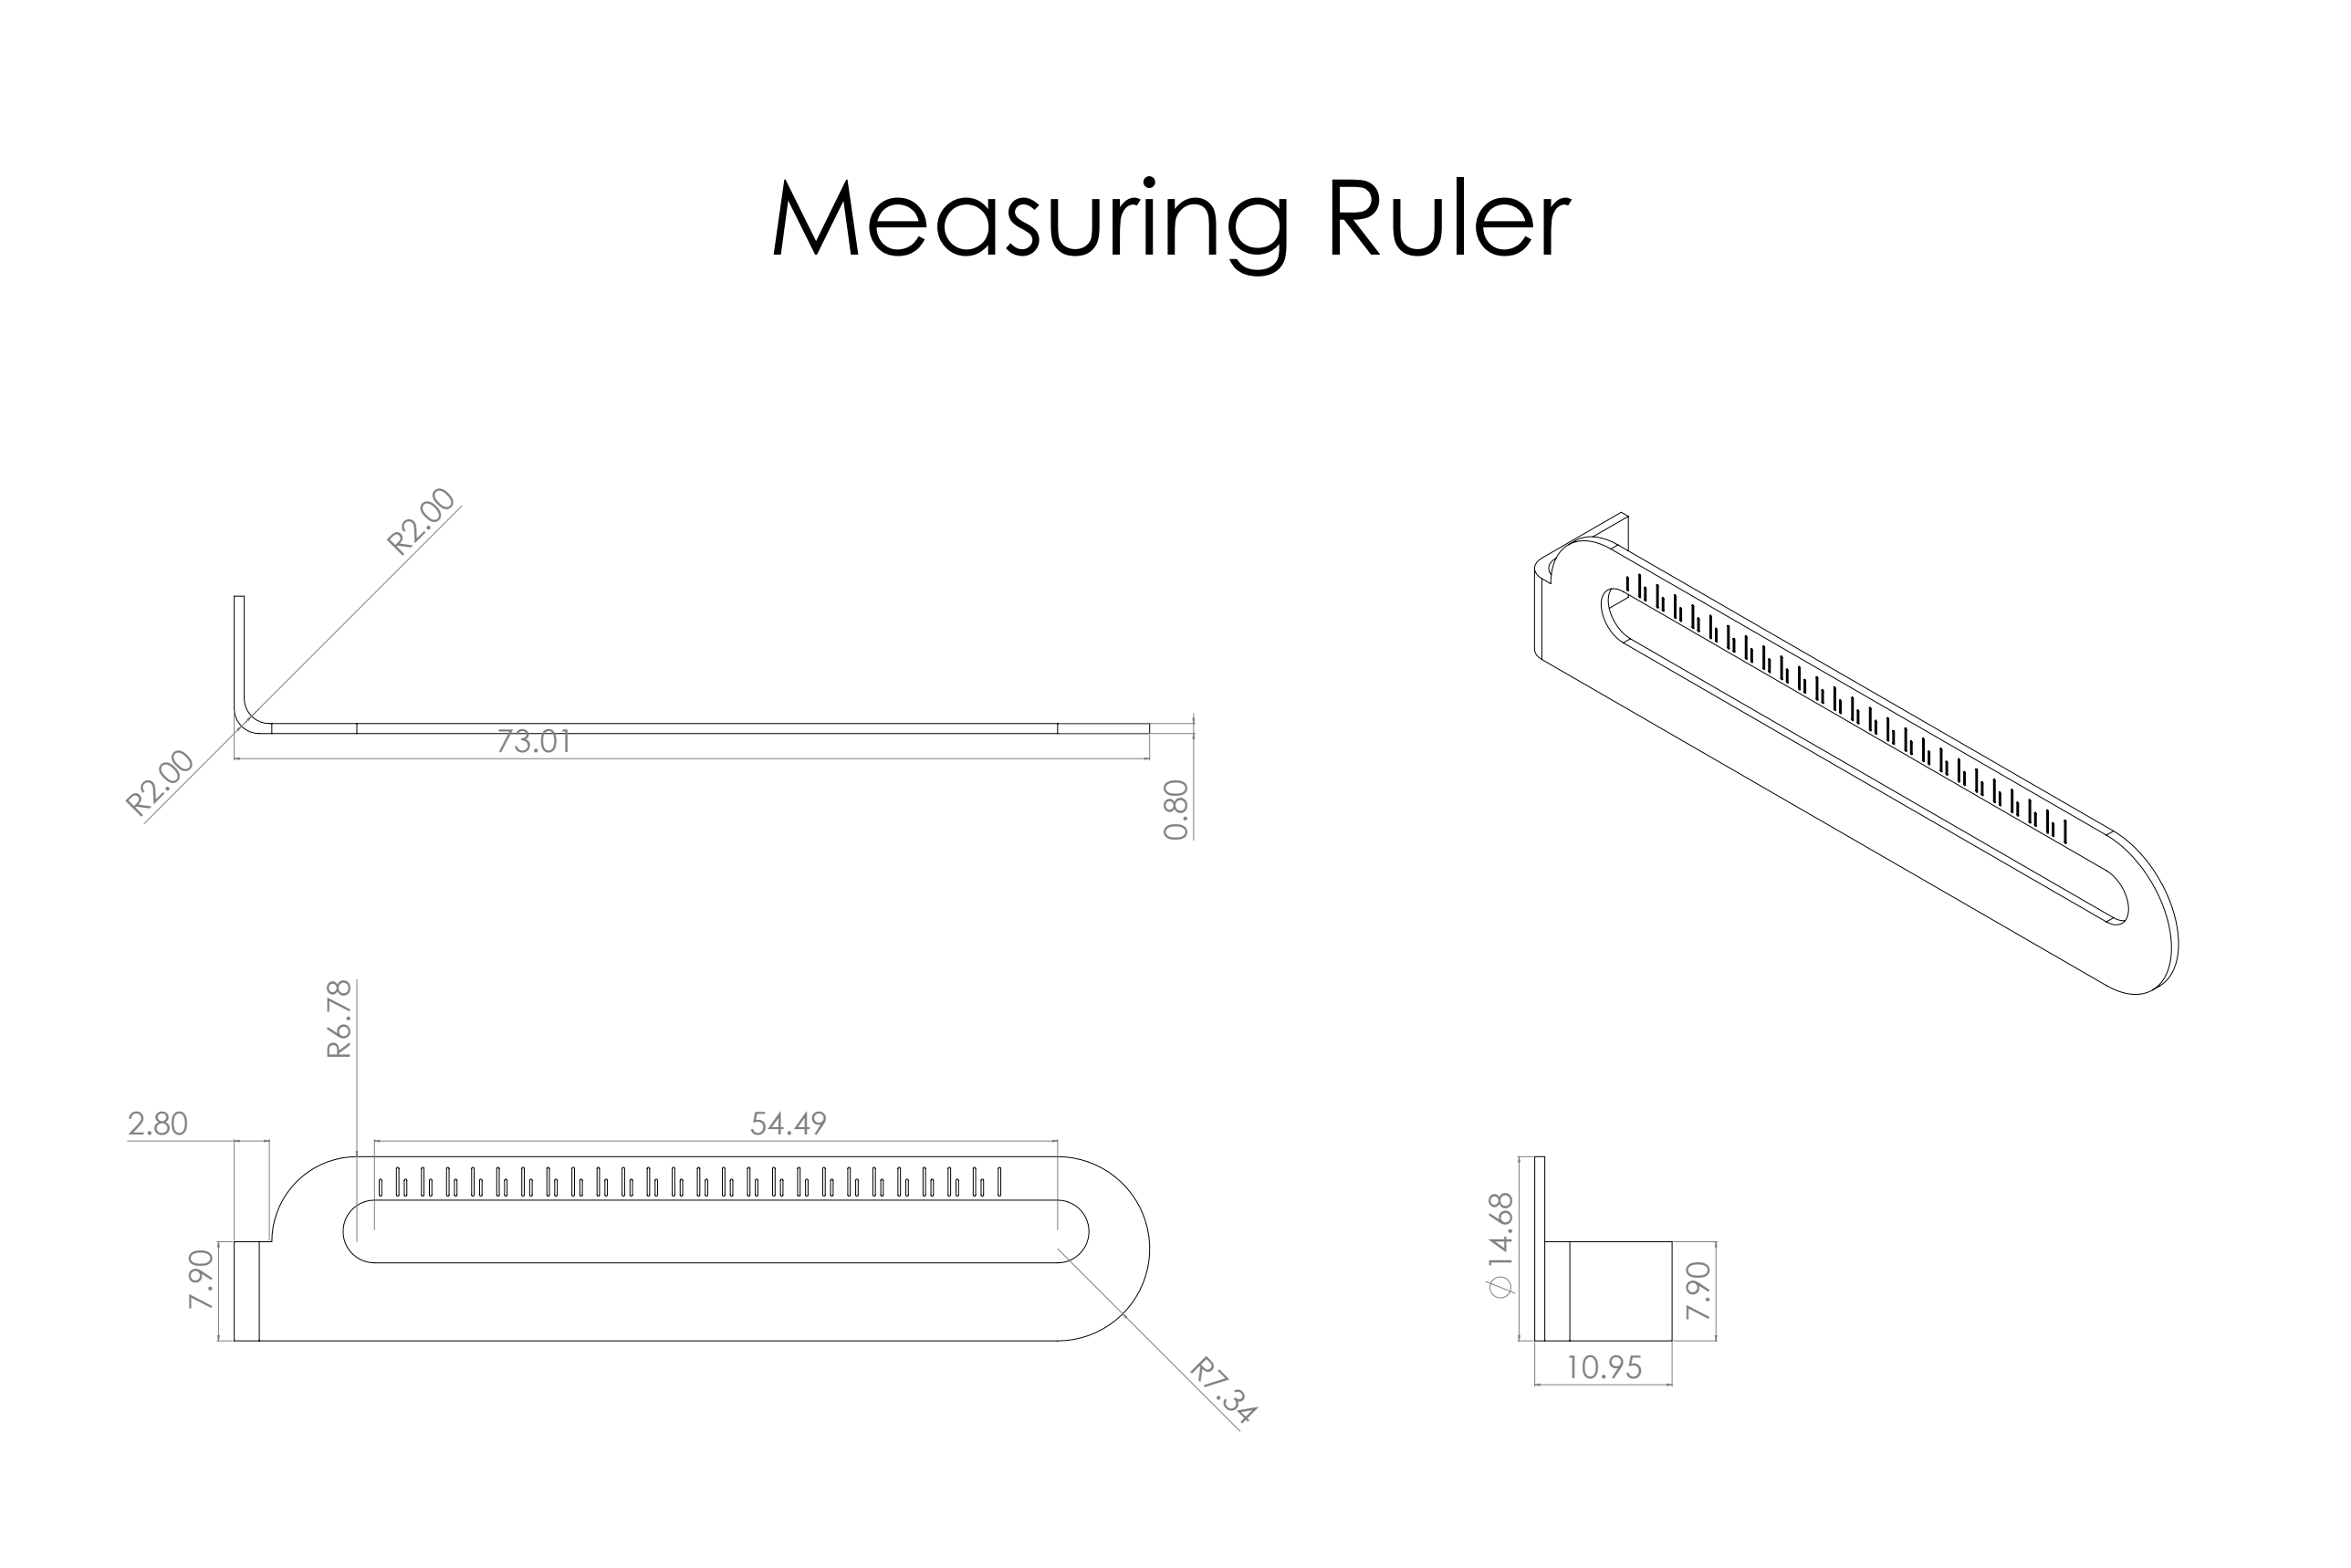
ISO-10303-21;
HEADER;
FILE_DESCRIPTION (('STEP AP214'),
    '1' );
FILE_NAME ('Measuring Ruler.step',
    '2026-10-24T22:54:28',
    ( '' ),
    ( '' ),
    'SwSTEP 2.0',
    'SolidWorks 2025',
    '' );
FILE_SCHEMA (( 'AUTOMOTIVE_DESIGN' ));
ENDSEC;

DATA;
#22=CIRCLE ( 'NONE', #10506, 0.1000000000000028644 ) ;
#24=ORIENTED_EDGE ( 'NONE', *, *, #28416, .F. ) ;
#30=EDGE_CURVE ( 'NONE', #25319, #33264, #34800, .T. ) ;
#32=ORIENTED_EDGE ( 'NONE', *, *, #7574, .F. ) ;
#37=DIRECTION ( 'NONE',  ( 1.000000000000000000, 0.000000000000000000, 0.000000000000000000 ) ) ;
#41=ORIENTED_EDGE ( 'NONE', *, *, #18908, .F. ) ;
#44=DIRECTION ( 'NONE',  ( -0.000000000000000000, -0.000000000000000000, 1.000000000000000000 ) ) ;
#48=CIRCLE ( 'NONE', #2012, 0.1000000000000028644 ) ;
#49=CARTESIAN_POINT ( 'NONE',  ( -32.87867591359218977, -26.64985754041175525, 6.700000000000000178 ) ) ;
#51=ORIENTED_EDGE ( 'NONE', *, *, #25814, .F. ) ;
#52=FACE_BOUND ( 'NONE', #30582, .T. ) ;
#54=EDGE_LOOP ( 'NONE', ( #15981, #402, #1244, #38858 ) ) ;
#57=EDGE_CURVE ( 'NONE', #6790, #7577, #6515, .T. ) ;
#60=ORIENTED_EDGE ( 'NONE', *, *, #39491, .F. ) ;
#63=CARTESIAN_POINT ( 'NONE',  ( -19.07867591359219972, -24.55319635012989110, 6.800000000000000711 ) ) ;
#69=DIRECTION ( 'NONE',  ( 0.000000000000000000, 0.000000000000000000, 1.000000000000000000 ) ) ;
#80=EDGE_CURVE ( 'NONE', #2391, #5443, #34066, .T. ) ;
#89=DIRECTION ( 'NONE',  ( -0.000000000000000000, -0.000000000000000000, 1.000000000000000000 ) ) ;
#92=CARTESIAN_POINT ( 'NONE',  ( -14.44874870218064089, -26.64985754041175525, 6.700000000000000178 ) ) ;
#93=ORIENTED_EDGE ( 'NONE', *, *, #2114, .F. ) ;
#96=AXIS2_PLACEMENT_3D ( 'NONE', #13585, #39295, #10487 ) ;
#107=VECTOR ( 'NONE', #13832, 1000.000000000000000 ) ;
#112=CARTESIAN_POINT ( 'NONE',  ( -40.44874870218063734, -26.64985754041175525, 6.700000000000000178 ) ) ;
#116=EDGE_CURVE ( 'NONE', #25222, #15928, #15693, .T. ) ;
#121=EDGE_LOOP ( 'NONE', ( #23412, #22869, #10746, #16528 ) ) ;
#138=VECTOR ( 'NONE', #4313, 1000.000000000000000 ) ;
#160=VERTEX_POINT ( 'NONE', #28468 ) ;
#162=DIRECTION ( 'NONE',  ( 1.000000000000000000, 0.000000000000000000, 0.000000000000000000 ) ) ;
#168=EDGE_CURVE ( 'NONE', #27559, #13108, #28679, .T. ) ;
#169=VERTEX_POINT ( 'NONE', #9734 ) ;
#172=ADVANCED_FACE ( 'NONE', ( #34882 ), #28059, .T. ) ;
#179=LINE ( 'NONE', #33956, #26669 ) ;
#182=CARTESIAN_POINT ( 'NONE',  ( -32.44874870218063734, -26.64985754041175525, 6.700000000000000178 ) ) ;
#188=EDGE_LOOP ( 'NONE', ( #27353, #29698, #8514, #37884 ) ) ;
#192=AXIS2_PLACEMENT_3D ( 'NONE', #26818, #39356, #4992 ) ;
#194=DIRECTION ( 'NONE',  ( -0.000000000000000000, -1.000000000000000000, -0.000000000000000000 ) ) ;
#203=ORIENTED_EDGE ( 'NONE', *, *, #13724, .F. ) ;
#205=CARTESIAN_POINT ( 'NONE',  ( -31.07867591359219617, -26.64985754041175525, 6.700000000000000178 ) ) ;
#210=VECTOR ( 'NONE', #7329, 1000.000000000000000 ) ;
#212=VERTEX_POINT ( 'NONE', #19008 ) ;
#219=VECTOR ( 'NONE', #28713, 1000.000000000000000 ) ;
#221=ORIENTED_EDGE ( 'NONE', *, *, #39543, .T. ) ;
#228=CARTESIAN_POINT ( 'NONE',  ( -38.34874870218063592, -25.49307895267003587, 6.800000000000000711 ) ) ;
#229=VECTOR ( 'NONE', #9739, 1000.000000000000000 ) ;
#230=AXIS2_PLACEMENT_3D ( 'NONE', #30843, #30009, #20734 ) ;
#232=ORIENTED_EDGE ( 'NONE', *, *, #27570, .F. ) ;
#236=EDGE_CURVE ( 'NONE', #37067, #38999, #489, .T. ) ;
#239=ORIENTED_EDGE ( 'NONE', *, *, #18400, .F. ) ;
#245=FACE_BOUND ( 'NONE', #8668, .T. ) ;
#247=ORIENTED_EDGE ( 'NONE', *, *, #38016, .F. ) ;
#253=ORIENTED_EDGE ( 'NONE', *, *, #18491, .F. ) ;
#256=CARTESIAN_POINT ( 'NONE',  ( -20.24874870218063805, -26.64985754041175525, 6.800000000000000711 ) ) ;
#261=CARTESIAN_POINT ( 'NONE',  ( -31.07867591359219617, -26.64985754041175525, 6.700000000000000178 ) ) ;
#264=EDGE_CURVE ( 'NONE', #4144, #39141, #13023, .T. ) ;
#273=VERTEX_POINT ( 'NONE', #6042 ) ;
#287=ORIENTED_EDGE ( 'NONE', *, *, #2540, .F. ) ;
#291=VECTOR ( 'NONE', #8251, 1000.000000000000000 ) ;
#292=ORIENTED_EDGE ( 'NONE', *, *, #32328, .T. ) ;
#295=CARTESIAN_POINT ( 'NONE',  ( -28.44874870218064444, -26.64985754041175525, 6.700000000000000178 ) ) ;
#301=VERTEX_POINT ( 'NONE', #29083 ) ;
#308=AXIS2_PLACEMENT_3D ( 'NONE', #26975, #18099, #31499 ) ;
#316=CARTESIAN_POINT ( 'NONE',  ( -20.24874870218063805, -25.49307895267003587, 6.800000000000000711 ) ) ;
#324=CIRCLE ( 'NONE', #4910, 0.1000000000000028644 ) ;
#325=AXIS2_PLACEMENT_3D ( 'NONE', #22553, #3830, #34311 ) ;
#333=CARTESIAN_POINT ( 'NONE',  ( -40.87867591359218977, -26.64985754041175525, 6.700000000000000178 ) ) ;
#334=LINE ( 'NONE', #37983, #38784 ) ;
#335=VECTOR ( 'NONE', #17674, 1000.000000000000000 ) ;
#337=DIRECTION ( 'NONE',  ( -0.000000000000000000, -0.000000000000000000, 1.000000000000000000 ) ) ;
#339=CARTESIAN_POINT ( 'NONE',  ( -18.44874870218064089, -26.64985754041175525, 6.800000000000000711 ) ) ;
#340=ORIENTED_EDGE ( 'NONE', *, *, #35850, .F. ) ;
#342=ADVANCED_FACE ( 'NONE', ( #36253 ), #23687, .F. ) ;
#351=EDGE_CURVE ( 'NONE', #2784, #15795, #11729, .T. ) ;
#356=AXIS2_PLACEMENT_3D ( 'NONE', #19003, #36206, #4906 ) ;
#365=ORIENTED_EDGE ( 'NONE', *, *, #29479, .F. ) ;
#366=PLANE ( 'NONE',  #31779 ) ;
#375=LINE ( 'NONE', #9824, #24005 ) ;
#387=AXIS2_PLACEMENT_3D ( 'NONE', #30030, #29821, #1845 ) ;
#388=AXIS2_PLACEMENT_3D ( 'NONE', #3065, #40471, #13104 ) ;
#390=CARTESIAN_POINT ( 'NONE',  ( -19.07867591359219972, -24.55319635012989110, 6.700000000000000178 ) ) ;
#397=ORIENTED_EDGE ( 'NONE', *, *, #11518, .F. ) ;
#402=ORIENTED_EDGE ( 'NONE', *, *, #15855, .F. ) ;
#403=CARTESIAN_POINT ( 'NONE',  ( -10.97867591359219475, -24.55319635012989110, 6.800000000000000711 ) ) ;
#405=ORIENTED_EDGE ( 'NONE', *, *, #6491, .T. ) ;
#406=CARTESIAN_POINT ( 'NONE',  ( 0.9213240864078056092, -26.64985754041175525, 6.800000000000000711 ) ) ;
#407=EDGE_CURVE ( 'NONE', #9686, #33055, #7841, .T. ) ;
#408=VERTEX_POINT ( 'NONE', #26392 ) ;
#414=VECTOR ( 'NONE', #27211, 1000.000000000000000 ) ;
#423=VECTOR ( 'NONE', #27841, 1000.000000000000000 ) ;
#430=EDGE_LOOP ( 'NONE', ( #38499, #2239, #5855, #4124 ) ) ;
#438=DIRECTION ( 'NONE',  ( 1.000000000000000000, 0.000000000000000000, 0.000000000000000000 ) ) ;
#439=FACE_OUTER_BOUND ( 'NONE', #33105, .T. ) ;
#442=ORIENTED_EDGE ( 'NONE', *, *, #39133, .F. ) ;
#444=DIRECTION ( 'NONE',  ( 1.000000000000000000, 0.000000000000000000, 0.000000000000000000 ) ) ;
#450=ORIENTED_EDGE ( 'NONE', *, *, #24702, .T. ) ;
#456=FACE_BOUND ( 'NONE', #19493, .T. ) ;
#457=ORIENTED_EDGE ( 'NONE', *, *, #19911, .F. ) ;
#469=DIRECTION ( 'NONE',  ( 1.000000000000000000, 0.000000000000000000, -0.000000000000000000 ) ) ;
#472=CARTESIAN_POINT ( 'NONE',  ( 7.021324086407807030, -26.64985754041175525, 6.800000000000000711 ) ) ;
#477=CARTESIAN_POINT ( 'NONE',  ( -36.44874870218064444, -26.64985754041175525, 6.800000000000000711 ) ) ;
#480=EDGE_CURVE ( 'NONE', #34939, #11908, #22301, .T. ) ;
#482=VECTOR ( 'NONE', #26893, 1000.000000000000000 ) ;
#484=AXIS2_PLACEMENT_3D ( 'NONE', #25294, #37829, #22816 ) ;
#489=LINE ( 'NONE', #19409, #17633 ) ;
#492=CARTESIAN_POINT ( 'NONE',  ( 3.121324086407806231, -24.55319635012989110, 6.800000000000000711 ) ) ;
#504=ORIENTED_EDGE ( 'NONE', *, *, #40555, .F. ) ;
#510=CIRCLE ( 'NONE', #40591, 0.1000000000000028644 ) ;
#511=AXIS2_PLACEMENT_3D ( 'NONE', #33114, #5508, #36395 ) ;
#512=DIRECTION ( 'NONE',  ( 1.000000000000000000, -0.000000000000000000, 0.000000000000000000 ) ) ;
#513=VERTEX_POINT ( 'NONE', #23285 ) ;
#525=CARTESIAN_POINT ( 'NONE',  ( -28.44874870218064444, -26.64985754041175525, 6.800000000000000711 ) ) ;
#528=EDGE_CURVE ( 'NONE', #40182, #12066, #7030, .T. ) ;
#529=DIRECTION ( 'NONE',  ( 0.000000000000000000, 1.000000000000000000, 0.000000000000000000 ) ) ;
#534=DIRECTION ( 'NONE',  ( 0.000000000000000000, 1.000000000000000000, 0.000000000000000000 ) ) ;
#543=EDGE_CURVE ( 'NONE', #29781, #29208, #27533, .T. ) ;
#547=CARTESIAN_POINT ( 'NONE',  ( -31.07867591359219617, -26.64985754041175525, 6.700000000000000178 ) ) ;
#554=ADVANCED_FACE ( 'NONE', ( #16885 ), #25774, .F. ) ;
#563=CIRCLE ( 'NONE', #18272, 0.1000000000000028644 ) ;
#570=AXIS2_PLACEMENT_3D ( 'NONE', #16960, #5023, #19858 ) ;
#578=DIRECTION ( 'NONE',  ( -0.000000000000000000, -0.000000000000000000, 1.000000000000000000 ) ) ;
#594=CARTESIAN_POINT ( 'NONE',  ( -26.87867591359219333, -26.64985754041175525, 6.700000000000000178 ) ) ;
#605=ORIENTED_EDGE ( 'NONE', *, *, #39024, .T. ) ;
#607=ORIENTED_EDGE ( 'NONE', *, *, #26724, .T. ) ;
#608=VECTOR ( 'NONE', #5163, 1000.000000000000000 ) ;
#619=DIRECTION ( 'NONE',  ( 0.000000000000000000, 0.000000000000000000, -1.000000000000000000 ) ) ;
#630=EDGE_LOOP ( 'NONE', ( #15162, #24602, #9016, #12961 ) ) ;
#641=ADVANCED_FACE ( 'NONE', ( #18306 ), #6386, .T. ) ;
#642=AXIS2_PLACEMENT_3D ( 'NONE', #18718, #9661, #9043 ) ;
#650=VERTEX_POINT ( 'NONE', #31702 ) ;
#653=CARTESIAN_POINT ( 'NONE',  ( -8.448748702180639114, -26.64985754041175525, 6.700000000000000178 ) ) ;
#656=EDGE_LOOP ( 'NONE', ( #16676, #14194, #23824, #26128 ) ) ;
#659=ORIENTED_EDGE ( 'NONE', *, *, #28607, .F. ) ;
#661=CARTESIAN_POINT ( 'NONE',  ( -4.978675913592189417, -26.64985754041175525, 6.800000000000000711 ) ) ;
#662=ORIENTED_EDGE ( 'NONE', *, *, #39276, .T. ) ;
#682=ADVANCED_FACE ( 'NONE', ( #22247 ), #28186, .F. ) ;
#683=AXIS2_PLACEMENT_3D ( 'NONE', #24668, #40497, #3294 ) ;
#687=CARTESIAN_POINT ( 'NONE',  ( 5.121324086407808451, -26.64985754041175525, 6.800000000000000711 ) ) ;
#697=AXIS2_PLACEMENT_3D ( 'NONE', #25369, #6431, #21672 ) ;
#699=VERTEX_POINT ( 'NONE', #31500 ) ;
#706=CARTESIAN_POINT ( 'NONE',  ( 2.921324086407800280, -26.64985754041175525, 6.700000000000000178 ) ) ;
#710=CARTESIAN_POINT ( 'NONE',  ( -24.87867591359218977, -26.64985754041175525, 6.700000000000000178 ) ) ;
#719=AXIS2_PLACEMENT_3D ( 'NONE', #16756, #1542, #11181 ) ;
#721=DIRECTION ( 'NONE',  ( -1.000000000000000000, 0.000000000000000000, 0.000000000000000000 ) ) ;
#730=EDGE_CURVE ( 'NONE', #28082, #6110, #14379, .T. ) ;
#739=VECTOR ( 'NONE', #13481, 1000.000000000000000 ) ;
#740=DIRECTION ( 'NONE',  ( 1.000000000000000000, 0.000000000000000000, -0.000000000000000000 ) ) ;
#744=VERTEX_POINT ( 'NONE', #2705 ) ;
#745=AXIS2_PLACEMENT_3D ( 'NONE', #8431, #24083, #11717 ) ;
#746=ORIENTED_EDGE ( 'NONE', *, *, #18980, .F. ) ;
#752=ORIENTED_EDGE ( 'NONE', *, *, #26701, .T. ) ;
#756=CYLINDRICAL_SURFACE ( 'NONE', #23191, 0.1000000000000028644 ) ;
#759=CARTESIAN_POINT ( 'NONE',  ( 6.921324086407803833, -24.55319635012989110, 6.800000000000000711 ) ) ;
#779=ADVANCED_FACE ( 'NONE', ( #28815 ), #25521, .F. ) ;
#793=EDGE_CURVE ( 'NONE', #37191, #15824, #9816, .T. ) ;
#794=LINE ( 'NONE', #22821, #9570 ) ;
#796=ORIENTED_EDGE ( 'NONE', *, *, #39201, .T. ) ;
#801=ORIENTED_EDGE ( 'NONE', *, *, #26499, .T. ) ;
#806=ORIENTED_EDGE ( 'NONE', *, *, #32982, .T. ) ;
#813=AXIS2_PLACEMENT_3D ( 'NONE', #2939, #28428, #28639 ) ;
#817=CARTESIAN_POINT ( 'NONE',  ( 5.751251297819365504, -25.49307895267003587, 6.700000000000000178 ) ) ;
#821=CYLINDRICAL_SURFACE ( 'NONE', #26427, 0.1000000000000028644 ) ;
#825=ORIENTED_EDGE ( 'NONE', *, *, #17697, .T. ) ;
#826=VERTEX_POINT ( 'NONE', #19549 ) ;
#840=CYLINDRICAL_SURFACE ( 'NONE', #9559, 0.1000000000000028644 ) ;
#844=CARTESIAN_POINT ( 'NONE',  ( 5.751251297819365504, -26.64985754041175525, 6.700000000000000178 ) ) ;
#846=LINE ( 'NONE', #13981, #2059 ) ;
#848=EDGE_LOOP ( 'NONE', ( #12316, #20240, #26085, #37691 ) ) ;
#849=ORIENTED_EDGE ( 'NONE', *, *, #22675, .F. ) ;
#854=EDGE_CURVE ( 'NONE', #36422, #301, #38867, .T. ) ;
#856=ORIENTED_EDGE ( 'NONE', *, *, #2258, .T. ) ;
#857=ADVANCED_FACE ( 'NONE', ( #8582 ), #23435, .F. ) ;
#860=ORIENTED_EDGE ( 'NONE', *, *, #25488, .F. ) ;
#861=FACE_BOUND ( 'NONE', #37475, .T. ) ;
#863=VERTEX_POINT ( 'NONE', #8375 ) ;
#865=EDGE_CURVE ( 'NONE', #14656, #4406, #26525, .T. ) ;
#876=LINE ( 'NONE', #31758, #28712 ) ;
#877=EDGE_CURVE ( 'NONE', #28154, #25277, #11252, .T. ) ;
#899=CARTESIAN_POINT ( 'NONE',  ( -54.01549048184568846, -38.28842912540938670, 4.800000000000000711 ) ) ;
#901=CYLINDRICAL_SURFACE ( 'NONE', #8152, 0.1000000000000028644 ) ;
#907=EDGE_CURVE ( 'NONE', #5789, #22409, #33321, .T. ) ;
#915=AXIS2_PLACEMENT_3D ( 'NONE', #29380, #4276, #4480 ) ;
#916=EDGE_CURVE ( 'NONE', #8305, #24066, #39886, .T. ) ;
#927=ORIENTED_EDGE ( 'NONE', *, *, #964, .F. ) ;
#930=ORIENTED_EDGE ( 'NONE', *, *, #27699, .T. ) ;
#935=EDGE_LOOP ( 'NONE', ( #34001, #29049, #22823, #20751 ) ) ;
#941=CARTESIAN_POINT ( 'NONE',  ( -4.878675913592187108, -26.64985754041175525, 6.700000000000000178 ) ) ;
#942=DIRECTION ( 'NONE',  ( 1.000000000000000000, 0.000000000000000000, -0.000000000000000000 ) ) ;
#943=CIRCLE ( 'NONE', #6193, 0.1000000000000028644 ) ;
#946=VECTOR ( 'NONE', #20283, 1000.000000000000000 ) ;
#956=CARTESIAN_POINT ( 'NONE',  ( -34.34874870218063592, -26.64985754041175525, 6.700000000000000178 ) ) ;
#964=EDGE_CURVE ( 'NONE', #14571, #23320, #17842, .T. ) ;
#967=CARTESIAN_POINT ( 'NONE',  ( -26.34874870218063947, -25.49307895267003587, 6.700000000000000178 ) ) ;
#970=EDGE_LOOP ( 'NONE', ( #15579, #17607, #22271, #8008 ) ) ;
#972=LINE ( 'NONE', #29558, #210 ) ;
#986=CARTESIAN_POINT ( 'NONE',  ( -26.34874870218063947, -26.64985754041175525, 6.700000000000000178 ) ) ;
#993=CARTESIAN_POINT ( 'NONE',  ( -32.87867591359218977, -24.55319635012989110, 6.700000000000000178 ) ) ;
#1000=ADVANCED_FACE ( 'NONE', ( #27123 ), #39673, .F. ) ;
#1001=AXIS2_PLACEMENT_3D ( 'NONE', #28881, #26404, #13835 ) ;
#1013=ORIENTED_EDGE ( 'NONE', *, *, #7946, .T. ) ;
#1018=FACE_OUTER_BOUND ( 'NONE', #9894, .T. ) ;
#1020=EDGE_LOOP ( 'NONE', ( #6917, #5481, #6006, #10397 ) ) ;
#1046=CARTESIAN_POINT ( 'NONE',  ( 4.921324086407802056, -26.64985754041175525, 6.800000000000000711 ) ) ;
#1049=EDGE_CURVE ( 'NONE', #35752, #27725, #24236, .T. ) ;
#1053=DIRECTION ( 'NONE',  ( 0.000000000000000000, 0.000000000000000000, 1.000000000000000000 ) ) ;
#1056=ORIENTED_EDGE ( 'NONE', *, *, #36941, .T. ) ;
#1062=CIRCLE ( 'NONE', #24030, 0.1000000000000028644 ) ;
#1065=DIRECTION ( 'NONE',  ( 0.000000000000000000, 0.000000000000000000, 1.000000000000000000 ) ) ;
#1066=ADVANCED_FACE ( 'NONE', ( #18462 ), #18664, .F. ) ;
#1074=CARTESIAN_POINT ( 'NONE',  ( -40.44874870218063734, -25.49307895267003587, 6.700000000000000178 ) ) ;
#1086=LINE ( 'NONE', #32373, #21513 ) ;
#1091=DIRECTION ( 'NONE',  ( -0.000000000000000000, -0.000000000000000000, -1.000000000000000000 ) ) ;
#1096=EDGE_CURVE ( 'NONE', #25156, #27940, #9398, .T. ) ;
#1104=EDGE_CURVE ( 'NONE', #38102, #33506, #2654, .T. ) ;
#1108=CIRCLE ( 'NONE', #9635, 0.1000000000000028644 ) ;
#1111=CARTESIAN_POINT ( 'NONE',  ( -34.44874870218064444, -26.64985754041175525, 6.800000000000000711 ) ) ;
#1125=CARTESIAN_POINT ( 'NONE',  ( -40.44874870218063734, -25.49307895267003587, 6.700000000000000178 ) ) ;
#1135=CIRCLE ( 'NONE', #6382, 0.1000000000000028644 ) ;
#1142=VERTEX_POINT ( 'NONE', #37201 ) ;
#1148=EDGE_CURVE ( 'NONE', #7017, #3657, #26261, .T. ) ;
#1149=VERTEX_POINT ( 'NONE', #37403 ) ;
#1152=DIRECTION ( 'NONE',  ( -0.000000000000000000, -0.000000000000000000, 1.000000000000000000 ) ) ;
#1166=CIRCLE ( 'NONE', #39261, 0.1000000000000028644 ) ;
#1173=DIRECTION ( 'NONE',  ( -0.000000000000000000, -0.000000000000000000, 1.000000000000000000 ) ) ;
#1174=ORIENTED_EDGE ( 'NONE', *, *, #2356, .F. ) ;
#1187=LINE ( 'NONE', #35955, #946 ) ;
#1190=VERTEX_POINT ( 'NONE', #4067 ) ;
#1195=DIRECTION ( 'NONE',  ( 0.000000000000000000, 1.000000000000000000, 0.000000000000000000 ) ) ;
#1207=AXIS2_PLACEMENT_3D ( 'NONE', #23187, #22594, #13911 ) ;
#1211=CYLINDRICAL_SURFACE ( 'NONE', #10209, 0.1000000000000028644 ) ;
#1216=AXIS2_PLACEMENT_3D ( 'NONE', #27119, #20943, #2227 ) ;
#1220=PLANE ( 'NONE',  #30647 ) ;
#1223=EDGE_LOOP ( 'NONE', ( #35956, #16011, #20211, #34093 ) ) ;
#1235=CARTESIAN_POINT ( 'NONE',  ( -40.44874870218063734, -26.64985754041175525, 6.700000000000000178 ) ) ;
#1237=ORIENTED_EDGE ( 'NONE', *, *, #1249, .T. ) ;
#1238=DIRECTION ( 'NONE',  ( 0.000000000000000000, 0.000000000000000000, 1.000000000000000000 ) ) ;
#1244=ORIENTED_EDGE ( 'NONE', *, *, #36356, .F. ) ;
#1249=EDGE_CURVE ( 'NONE', #12996, #5611, #7868, .T. ) ;
#1251=CARTESIAN_POINT ( 'NONE',  ( -14.24874870218063450, -25.49307895267003587, 6.700000000000000178 ) ) ;
#1255=DIRECTION ( 'NONE',  ( 1.000000000000000000, 0.000000000000000000, 0.000000000000000000 ) ) ;
#1267=EDGE_CURVE ( 'NONE', #26853, #22787, #24958, .T. ) ;
#1269=VERTEX_POINT ( 'NONE', #3673 ) ;
#1273=AXIS2_PLACEMENT_3D ( 'NONE', #4046, #3453, #6716 ) ;
#1285=CARTESIAN_POINT ( 'NONE',  ( -35.07867591359219972, -24.55319635012989110, 6.700000000000000178 ) ) ;
#1287=CARTESIAN_POINT ( 'NONE',  ( -5.078675913592192614, -26.64985754041175525, 6.800000000000000711 ) ) ;
#1291=CARTESIAN_POINT ( 'NONE',  ( 7.121324086407810228, -26.64985754041175525, 6.700000000000000178 ) ) ;
#1293=FACE_OUTER_BOUND ( 'NONE', #4220, .T. ) ;
#1298=LINE ( 'NONE', #26205, #3633 ) ;
#1299=FACE_OUTER_BOUND ( 'NONE', #3763, .T. ) ;
#1303=CYLINDRICAL_SURFACE ( 'NONE', #14814, 0.1000000000000028644 ) ;
#1316=DIRECTION ( 'NONE',  ( -0.000000000000000000, -0.000000000000000000, 1.000000000000000000 ) ) ;
#1326=CARTESIAN_POINT ( 'NONE',  ( -5.078675913592192614, -24.55319635012989110, 6.800000000000000711 ) ) ;
#1343=ORIENTED_EDGE ( 'NONE', *, *, #10404, .T. ) ;
#1344=CARTESIAN_POINT ( 'NONE',  ( -2.448748702180640446, -26.64985754041175525, 6.800000000000000711 ) ) ;
#1345=VECTOR ( 'NONE', #9294, 1000.000000000000000 ) ;
#1346=VERTEX_POINT ( 'NONE', #25375 ) ;
#1349=DIRECTION ( 'NONE',  ( -1.000000000000000000, 0.000000000000000000, 0.000000000000000000 ) ) ;
#1352=DIRECTION ( 'NONE',  ( 0.000000000000000000, 0.000000000000000000, 1.000000000000000000 ) ) ;
#1364=ORIENTED_EDGE ( 'NONE', *, *, #15068, .T. ) ;
#1368=CARTESIAN_POINT ( 'NONE',  ( -29.07867591359219617, -24.55319635012989110, 6.700000000000000178 ) ) ;
#1378=EDGE_CURVE ( 'NONE', #22687, #28211, #22091, .T. ) ;
#1389=CARTESIAN_POINT ( 'NONE',  ( -22.97867591359219119, -26.64985754041175525, 6.700000000000000178 ) ) ;
#1406=DIRECTION ( 'NONE',  ( -0.000000000000000000, -0.000000000000000000, 1.000000000000000000 ) ) ;
#1408=CARTESIAN_POINT ( 'NONE',  ( -6.878675913592188884, -26.64985754041175525, 6.800000000000000711 ) ) ;
#1412=FACE_OUTER_BOUND ( 'NONE', #24496, .T. ) ;
#1427=CARTESIAN_POINT ( 'NONE',  ( -20.87867591359218977, -24.55319635012989110, 6.700000000000000178 ) ) ;
#1435=CYLINDRICAL_SURFACE ( 'NONE', #15585, 0.1000000000000028644 ) ;
#1439=ORIENTED_EDGE ( 'NONE', *, *, #10916, .F. ) ;
#1445=CYLINDRICAL_SURFACE ( 'NONE', #14804, 0.1000000000000028644 ) ;
#1448=DIRECTION ( 'NONE',  ( 0.000000000000000000, 0.000000000000000000, 1.000000000000000000 ) ) ;
#1456=CARTESIAN_POINT ( 'NONE',  ( -4.248748702180636272, -26.64985754041175525, 6.700000000000000178 ) ) ;
#1461=CARTESIAN_POINT ( 'NONE',  ( -16.44874870218064089, -26.64985754041175525, 6.700000000000000178 ) ) ;
#1464=ORIENTED_EDGE ( 'NONE', *, *, #37587, .F. ) ;
#1472=FACE_OUTER_BOUND ( 'NONE', #14916, .T. ) ;
#1477=CARTESIAN_POINT ( 'NONE',  ( -14.44874870218064089, -25.49307895267003587, 6.800000000000000711 ) ) ;
#1478=CARTESIAN_POINT ( 'NONE',  ( 1.751251297819361730, -26.64985754041175525, 6.700000000000000178 ) ) ;
#1490=VECTOR ( 'NONE', #40411, 1000.000000000000000 ) ;
#1497=ORIENTED_EDGE ( 'NONE', *, *, #13901, .F. ) ;
#1528=ORIENTED_EDGE ( 'NONE', *, *, #12883, .F. ) ;
#1532=EDGE_CURVE ( 'NONE', #34807, #36832, #20388, .T. ) ;
#1535=ORIENTED_EDGE ( 'NONE', *, *, #18438, .F. ) ;
#1542=DIRECTION ( 'NONE',  ( 1.000000000000000000, -0.000000000000000000, 0.000000000000000000 ) ) ;
#1546=ADVANCED_FACE ( 'NONE', ( #35270 ), #19994, .F. ) ;
#1547=VERTEX_POINT ( 'NONE', #1477 ) ;
#1552=EDGE_LOOP ( 'NONE', ( #32484, #9373, #40170, #13436 ) ) ;
#1554=FACE_OUTER_BOUND ( 'NONE', #12637, .T. ) ;
#1555=LINE ( 'NONE', #1760, #19571 ) ;
#1558=CARTESIAN_POINT ( 'NONE',  ( -42.83131703149249603, -27.06993018339339585, 6.800000000000000711 ) ) ;
#1563=ORIENTED_EDGE ( 'NONE', *, *, #10637, .F. ) ;
#1569=CARTESIAN_POINT ( 'NONE',  ( -40.34874870218063592, -26.64985754041175525, 6.700000000000000178 ) ) ;
#1578=VECTOR ( 'NONE', #27868, 1000.000000000000000 ) ;
#1588=AXIS2_PLACEMENT_3D ( 'NONE', #33095, #29997, #36380 ) ;
#1593=AXIS2_PLACEMENT_3D ( 'NONE', #1881, #39938, #8632 ) ;
#1605=DIRECTION ( 'NONE',  ( 0.000000000000000000, 0.000000000000000000, 1.000000000000000000 ) ) ;
#1606=ORIENTED_EDGE ( 'NONE', *, *, #8051, .T. ) ;
#1608=AXIS2_PLACEMENT_3D ( 'NONE', #15904, #35622, #3386 ) ;
#1609=EDGE_LOOP ( 'NONE', ( #12170, #36601, #32369, #22372 ) ) ;
#1611=DIRECTION ( 'NONE',  ( 0.000000000000000000, 1.000000000000000000, 0.000000000000000000 ) ) ;
#1616=AXIS2_PLACEMENT_3D ( 'NONE', #28205, #37666, #37 ) ;
#1623=ORIENTED_EDGE ( 'NONE', *, *, #25818, .F. ) ;
#1625=ADVANCED_FACE ( 'NONE', ( #36450 ), #39738, .F. ) ;
#1632=ORIENTED_EDGE ( 'NONE', *, *, #32386, .F. ) ;
#1634=VERTEX_POINT ( 'NONE', #39327 ) ;
#1635=VECTOR ( 'NONE', #32985, 1000.000000000000000 ) ;
#1646=ADVANCED_FACE ( 'NONE', ( #4754 ), #33787, .T. ) ;
#1648=CARTESIAN_POINT ( 'NONE',  ( -10.97867591359219475, -26.64985754041175525, 6.800000000000000711 ) ) ;
#1651=ORIENTED_EDGE ( 'NONE', *, *, #17090, .F. ) ;
#1662=VERTEX_POINT ( 'NONE', #21427 ) ;
#1670=VECTOR ( 'NONE', #17832, 1000.000000000000000 ) ;
#1672=VERTEX_POINT ( 'NONE', #27382 ) ;
#1682=DIRECTION ( 'NONE',  ( -0.000000000000000000, -0.000000000000000000, 1.000000000000000000 ) ) ;
#1689=CARTESIAN_POINT ( 'NONE',  ( -40.87867591359218977, -26.64985754041175525, 6.700000000000000178 ) ) ;
#1694=DIRECTION ( 'NONE',  ( 0.000000000000000000, 1.000000000000000000, 0.000000000000000000 ) ) ;
#1699=CARTESIAN_POINT ( 'NONE',  ( -34.87867591359218977, -26.64985754041175525, 6.700000000000000178 ) ) ;
#1701=ADVANCED_FACE ( 'NONE', ( #1892 ), #8641, .F. ) ;
#1709=DIRECTION ( 'NONE',  ( 1.000000000000000000, 0.000000000000000000, 0.000000000000000000 ) ) ;
#1714=FACE_OUTER_BOUND ( 'NONE', #25111, .T. ) ;
#1720=ORIENTED_EDGE ( 'NONE', *, *, #30483, .F. ) ;
#1726=EDGE_CURVE ( 'NONE', #37911, #1142, #33590, .T. ) ;
#1728=CIRCLE ( 'NONE', #31979, 0.1000000000000028644 ) ;
#1739=EDGE_CURVE ( 'NONE', #13396, #17894, #21216, .T. ) ;
#1741=CYLINDRICAL_SURFACE ( 'NONE', #26897, 0.1000000000000028644 ) ;
#1751=EDGE_CURVE ( 'NONE', #39647, #9655, #36653, .T. ) ;
#1752=ORIENTED_EDGE ( 'NONE', *, *, #9288, .F. ) ;
#1759=CARTESIAN_POINT ( 'NONE',  ( -16.24874870218063450, -26.64985754041175525, 6.700000000000000178 ) ) ;
#1760=CARTESIAN_POINT ( 'NONE',  ( -38.87867591359218977, -24.55319635012989110, 6.700000000000000178 ) ) ;
#1763=CARTESIAN_POINT ( 'NONE',  ( -14.87867591359218977, -24.55319635012989110, 6.800000000000000711 ) ) ;
#1765=CARTESIAN_POINT ( 'NONE',  ( -42.44874870218064444, -26.64985754041175525, 6.800000000000000711 ) ) ;
#1776=ADVANCED_FACE ( 'NONE', ( #26788 ), #18106, .T. ) ;
#1783=CIRCLE ( 'NONE', #5060, 0.1000000000000028644 ) ;
#1789=CARTESIAN_POINT ( 'NONE',  ( -21.07867591359219617, -24.55319635012989110, 6.700000000000000178 ) ) ;
#1794=AXIS2_PLACEMENT_3D ( 'NONE', #16703, #23114, #7454 ) ;
#1797=FACE_OUTER_BOUND ( 'NONE', #1223, .T. ) ;
#1810=VERTEX_POINT ( 'NONE', #22041 ) ;
#1816=ORIENTED_EDGE ( 'NONE', *, *, #22261, .T. ) ;
#1824=ORIENTED_EDGE ( 'NONE', *, *, #4744, .F. ) ;
#1825=AXIS2_PLACEMENT_3D ( 'NONE', #26664, #13699, #35935 ) ;
#1831=FACE_OUTER_BOUND ( 'NONE', #14855, .T. ) ;
#1835=VERTEX_POINT ( 'NONE', #22257 ) ;
#1836=CARTESIAN_POINT ( 'NONE',  ( -4.878675913592187108, -26.64985754041175525, 6.700000000000000178 ) ) ;
#1845=DIRECTION ( 'NONE',  ( -1.000000000000000000, 0.000000000000000000, 0.000000000000000000 ) ) ;
#1846=ORIENTED_EDGE ( 'NONE', *, *, #6440, .T. ) ;
#1847=VECTOR ( 'NONE', #38622, 1000.000000000000000 ) ;
#1853=DIRECTION ( 'NONE',  ( 1.000000000000000000, -0.000000000000000000, 0.000000000000000000 ) ) ;
#1854=VERTEX_POINT ( 'NONE', #19145 ) ;
#1856=AXIS2_PLACEMENT_3D ( 'NONE', #19788, #35652, #4360 ) ;
#1858=ORIENTED_EDGE ( 'NONE', *, *, #20133, .T. ) ;
#1863=DIRECTION ( 'NONE',  ( 0.000000000000000000, 0.000000000000000000, 1.000000000000000000 ) ) ;
#1865=DIRECTION ( 'NONE',  ( 0.000000000000000000, 0.000000000000000000, -1.000000000000000000 ) ) ;
#1866=ORIENTED_EDGE ( 'NONE', *, *, #31728, .F. ) ;
#1870=EDGE_LOOP ( 'NONE', ( #14802, #25233, #20620, #14309 ) ) ;
#1874=VERTEX_POINT ( 'NONE', #34209 ) ;
#1875=EDGE_CURVE ( 'NONE', #37531, #18951, #31711, .T. ) ;
#1881=CARTESIAN_POINT ( 'NONE',  ( -38.97867591359219119, -24.55319635012989110, 6.700000000000000178 ) ) ;
#1886=ORIENTED_EDGE ( 'NONE', *, *, #30787, .T. ) ;
#1891=ADVANCED_FACE ( 'NONE', ( #11099 ), #39514, .F. ) ;
#1892=FACE_OUTER_BOUND ( 'NONE', #37559, .T. ) ;
#1894=DIRECTION ( 'NONE',  ( -0.000000000000000000, -0.000000000000000000, 1.000000000000000000 ) ) ;
#1908=CYLINDRICAL_SURFACE ( 'NONE', #36747, 0.1000000000000028644 ) ;
#1914=DIRECTION ( 'NONE',  ( 1.000000000000000000, 0.000000000000000000, 0.000000000000000000 ) ) ;
#1915=EDGE_LOOP ( 'NONE', ( #25208, #504, #34556, #14770 ) ) ;
#1922=CARTESIAN_POINT ( 'NONE',  ( -24.24874870218063450, -26.64985754041175525, 6.700000000000000178 ) ) ;
#1923=ORIENTED_EDGE ( 'NONE', *, *, #27065, .T. ) ;
#1927=VECTOR ( 'NONE', #36002, 1000.000000000000000 ) ;
#1938=EDGE_CURVE ( 'NONE', #11548, #21166, #3302, .T. ) ;
#1950=VECTOR ( 'NONE', #31112, 1000.000000000000000 ) ;
#1951=CARTESIAN_POINT ( 'NONE',  ( -42.34874870218063592, -25.49307895267003587, 6.700000000000000178 ) ) ;
#1963=AXIS2_PLACEMENT_3D ( 'NONE', #24863, #34356, #162 ) ;
#1977=ORIENTED_EDGE ( 'NONE', *, *, #3672, .F. ) ;
#1980=VERTEX_POINT ( 'NONE', #9444 ) ;
#1985=DIRECTION ( 'NONE',  ( 0.000000000000000000, 0.000000000000000000, 1.000000000000000000 ) ) ;
#2012=AXIS2_PLACEMENT_3D ( 'NONE', #37068, #27397, #30291 ) ;
#2021=ORIENTED_EDGE ( 'NONE', *, *, #4492, .F. ) ;
#2027=ORIENTED_EDGE ( 'NONE', *, *, #21238, .T. ) ;
#2039=CARTESIAN_POINT ( 'NONE',  ( -52.01549048184568846, -30.94667987854474234, 4.800000000000000711 ) ) ;
#2041=CIRCLE ( 'NONE', #39505, 0.1000000000000028644 ) ;
#2046=CARTESIAN_POINT ( 'NONE',  ( 2.921324086407800280, -26.64985754041175525, 6.700000000000000178 ) ) ;
#2051=CARTESIAN_POINT ( 'NONE',  ( 3.551251297819357777, -25.49307895267003587, 6.800000000000000711 ) ) ;
#2054=LINE ( 'NONE', #27347, #37824 ) ;
#2059=VECTOR ( 'NONE', #22867, 1000.000000000000000 ) ;
#2064=CIRCLE ( 'NONE', #23726, 0.1000000000000028644 ) ;
#2066=ADVANCED_FACE ( 'NONE', ( #19129 ), #29751, .F. ) ;
#2068=CYLINDRICAL_SURFACE ( 'NONE', #40521, 0.1000000000000028644 ) ;
#2070=ORIENTED_EDGE ( 'NONE', *, *, #18627, .T. ) ;
#2073=VERTEX_POINT ( 'NONE', #32454 ) ;
#2079=ORIENTED_EDGE ( 'NONE', *, *, #27186, .T. ) ;
#2091=CARTESIAN_POINT ( 'NONE',  ( -36.97867591359219119, -26.64985754041175525, 6.800000000000000711 ) ) ;
#2101=CIRCLE ( 'NONE', #19838, 0.1000000000000028644 ) ;
#2109=EDGE_CURVE ( 'NONE', #33369, #14626, #30795, .T. ) ;
#2114=EDGE_CURVE ( 'NONE', #39964, #16562, #33886, .T. ) ;
#2117=CARTESIAN_POINT ( 'NONE',  ( -10.44874870218064089, -25.49307895267003587, 6.800000000000000711 ) ) ;
#2121=CARTESIAN_POINT ( 'NONE',  ( -37.07867591359219261, -26.64985754041175525, 6.700000000000000178 ) ) ;
#2124=ORIENTED_EDGE ( 'NONE', *, *, #23648, .F. ) ;
#2128=DIRECTION ( 'NONE',  ( 0.000000000000000000, 0.000000000000000000, -1.000000000000000000 ) ) ;
#2136=ORIENTED_EDGE ( 'NONE', *, *, #11028, .F. ) ;
#2141=VERTEX_POINT ( 'NONE', #12018 ) ;
#2144=DIRECTION ( 'NONE',  ( -0.000000000000000000, -0.000000000000000000, 1.000000000000000000 ) ) ;
#2148=EDGE_CURVE ( 'NONE', #18519, #2141, #6073, .T. ) ;
#2157=FACE_OUTER_BOUND ( 'NONE', #188, .T. ) ;
#2167=EDGE_CURVE ( 'NONE', #3715, #26905, #3424, .T. ) ;
#2168=EDGE_LOOP ( 'NONE', ( #22253, #14634, #30880, #6210 ) ) ;
#2169=DIRECTION ( 'NONE',  ( 0.000000000000000000, 0.000000000000000000, 1.000000000000000000 ) ) ;
#2170=EDGE_CURVE ( 'NONE', #10700, #14079, #25417, .T. ) ;
#2177=VERTEX_POINT ( 'NONE', #112 ) ;
#2185=FACE_OUTER_BOUND ( 'NONE', #9760, .T. ) ;
#2191=AXIS2_PLACEMENT_3D ( 'NONE', #9283, #25359, #37897 ) ;
#2198=CARTESIAN_POINT ( 'NONE',  ( -24.87867591359218977, -26.64985754041175525, 6.800000000000000711 ) ) ;
#2202=DIRECTION ( 'NONE',  ( 1.000000000000000000, 0.000000000000000000, 0.000000000000000000 ) ) ;
#2214=DIRECTION ( 'NONE',  ( 1.000000000000000000, 0.000000000000000000, 0.000000000000000000 ) ) ;
#2220=EDGE_LOOP ( 'NONE', ( #19687, #27231, #11268, #39519 ) ) ;
#2226=ORIENTED_EDGE ( 'NONE', *, *, #20409, .T. ) ;
#2227=DIRECTION ( 'NONE',  ( 1.000000000000000000, 0.000000000000000000, 0.000000000000000000 ) ) ;
#2228=VECTOR ( 'NONE', #35385, 1000.000000000000000 ) ;
#2233=DIRECTION ( 'NONE',  ( -0.000000000000000000, -0.000000000000000000, 1.000000000000000000 ) ) ;
#2239=ORIENTED_EDGE ( 'NONE', *, *, #3669, .T. ) ;
#2246=CARTESIAN_POINT ( 'NONE',  ( -42.24874870218063450, -25.49307895267003587, 6.800000000000000711 ) ) ;
#2248=CARTESIAN_POINT ( 'NONE',  ( 3.021324086407803478, -26.64985754041175525, 6.700000000000000178 ) ) ;
#2258=EDGE_CURVE ( 'NONE', #12826, #20627, #22745, .T. ) ;
#2267=ORIENTED_EDGE ( 'NONE', *, *, #10039, .F. ) ;
#2270=VERTEX_POINT ( 'NONE', #1326 ) ;
#2275=ORIENTED_EDGE ( 'NONE', *, *, #4572, .T. ) ;
#2288=VECTOR ( 'NONE', #1694, 1000.000000000000000 ) ;
#2296=DIRECTION ( 'NONE',  ( 1.000000000000000000, 0.000000000000000000, 0.000000000000000000 ) ) ;
#2298=CARTESIAN_POINT ( 'NONE',  ( -18.24874870218063450, -25.49307895267003587, 6.700000000000000178 ) ) ;
#2307=CARTESIAN_POINT ( 'NONE',  ( -17.07867591359219617, -26.64985754041175525, 6.700000000000000178 ) ) ;
#2311=ADVANCED_FACE ( 'NONE', ( #39571 ), #33434, .F. ) ;
#2312=ORIENTED_EDGE ( 'NONE', *, *, #26458, .T. ) ;
#2324=LINE ( 'NONE', #31286, #29415 ) ;
#2325=AXIS2_PLACEMENT_3D ( 'NONE', #18583, #2989, #2368 ) ;
#2326=ORIENTED_EDGE ( 'NONE', *, *, #6440, .F. ) ;
#2329=ORIENTED_EDGE ( 'NONE', *, *, #16967, .F. ) ;
#2334=PLANE ( 'NONE',  #38990 ) ;
#2343=ORIENTED_EDGE ( 'NONE', *, *, #13097, .T. ) ;
#2345=EDGE_CURVE ( 'NONE', #33227, #4406, #24338, .T. ) ;
#2353=DIRECTION ( 'NONE',  ( 0.000000000000000000, 0.000000000000000000, 1.000000000000000000 ) ) ;
#2356=EDGE_CURVE ( 'NONE', #15938, #25969, #9713, .T. ) ;
#2368=DIRECTION ( 'NONE',  ( 0.000000000000000000, 0.000000000000000000, 1.000000000000000000 ) ) ;
#2386=ORIENTED_EDGE ( 'NONE', *, *, #14915, .F. ) ;
#2388=PLANE ( 'NONE',  #22227 ) ;
#2389=CIRCLE ( 'NONE', #35879, 2.500000000000002220 ) ;
#2391=VERTEX_POINT ( 'NONE', #27826 ) ;
#2399=ADVANCED_FACE ( 'NONE', ( #22292 ), #37301, .T. ) ;
#2406=EDGE_CURVE ( 'NONE', #25329, #39282, #6226, .T. ) ;
#2408=EDGE_CURVE ( 'NONE', #3093, #24473, #34891, .T. ) ;
#2410=DIRECTION ( 'NONE',  ( 0.000000000000000000, 1.000000000000000000, 0.000000000000000000 ) ) ;
#2420=ORIENTED_EDGE ( 'NONE', *, *, #24147, .F. ) ;
#2427=PLANE ( 'NONE',  #3026 ) ;
#2429=DIRECTION ( 'NONE',  ( -0.000000000000000000, -0.000000000000000000, 1.000000000000000000 ) ) ;
#2435=ORIENTED_EDGE ( 'NONE', *, *, #24869, .F. ) ;
#2437=PRODUCT_DEFINITION_CONTEXT ( 'detailed design', #18152, 'design' ) ;
#2438=ORIENTED_EDGE ( 'NONE', *, *, #17073, .F. ) ;
#2450=DIRECTION ( 'NONE',  ( 1.000000000000000000, 0.000000000000000000, 0.000000000000000000 ) ) ;
#2451=AXIS2_PLACEMENT_3D ( 'NONE', #38153, #18603, #31188 ) ;
#2452=CIRCLE ( 'NONE', #7688, 0.1000000000000028644 ) ;
#2455=DIRECTION ( 'NONE',  ( -0.000000000000000000, -0.000000000000000000, 1.000000000000000000 ) ) ;
#2459=EDGE_CURVE ( 'NONE', #32758, #699, #21468, .T. ) ;
#2465=ORIENTED_EDGE ( 'NONE', *, *, #16374, .T. ) ;
#2466=DIRECTION ( 'NONE',  ( 0.000000000000000000, 0.000000000000000000, 1.000000000000000000 ) ) ;
#2471=FACE_OUTER_BOUND ( 'NONE', #39837, .T. ) ;
#2485=DIRECTION ( 'NONE',  ( 1.000000000000000000, -0.000000000000000000, 0.000000000000000000 ) ) ;
#2497=CARTESIAN_POINT ( 'NONE',  ( -30.97867591359219119, -24.55319635012989110, 6.700000000000000178 ) ) ;
#2505=DIRECTION ( 'NONE',  ( 1.000000000000000000, 0.000000000000000000, 0.000000000000000000 ) ) ;
#2512=AXIS2_PLACEMENT_3D ( 'NONE', #3061, #34548, #38005 ) ;
#2517=DIRECTION ( 'NONE',  ( 0.000000000000000000, 0.000000000000000000, -1.000000000000000000 ) ) ;
#2529=DIRECTION ( 'NONE',  ( 0.000000000000000000, 0.000000000000000000, 1.000000000000000000 ) ) ;
#2535=CARTESIAN_POINT ( 'NONE',  ( 1.751251297819361730, -26.64985754041175525, 6.800000000000000711 ) ) ;
#2540=EDGE_CURVE ( 'NONE', #21166, #26423, #18557, .T. ) ;
#2542=DIRECTION ( 'NONE',  ( 1.000000000000000000, 0.000000000000000000, 0.000000000000000000 ) ) ;
#2551=ORIENTED_EDGE ( 'NONE', *, *, #18908, .T. ) ;
#2552=DIRECTION ( 'NONE',  ( 1.000000000000000000, 0.000000000000000000, 0.000000000000000000 ) ) ;
#2555=LINE ( 'NONE', #37703, #38851 ) ;
#2564=ORIENTED_EDGE ( 'NONE', *, *, #16447, .T. ) ;
#2573=DIRECTION ( 'NONE',  ( -0.000000000000000000, -1.000000000000000000, -0.000000000000000000 ) ) ;
#2580=EDGE_CURVE ( 'NONE', #29188, #40280, #39417, .T. ) ;
#2584=VERTEX_POINT ( 'NONE', #63 ) ;
#2586=VECTOR ( 'NONE', #39592, 1000.000000000000000 ) ;
#2587=LINE ( 'NONE', #15923, #15386 ) ;
#2596=EDGE_CURVE ( 'NONE', #17770, #15824, #30395, .T. ) ;
#2600=ORIENTED_EDGE ( 'NONE', *, *, #26276, .F. ) ;
#2611=DIRECTION ( 'NONE',  ( 0.000000000000000000, 0.000000000000000000, 1.000000000000000000 ) ) ;
#2621=CARTESIAN_POINT ( 'NONE',  ( -6.878675913592188884, -26.64985754041175525, 6.700000000000000178 ) ) ;
#2634=ADVANCED_FACE ( 'NONE', ( #40252 ), #27292, .F. ) ;
#2635=FACE_OUTER_BOUND ( 'NONE', #28603, .T. ) ;
#2639=DIRECTION ( 'NONE',  ( -0.000000000000000000, -0.000000000000000000, 1.000000000000000000 ) ) ;
#2640=CARTESIAN_POINT ( 'NONE',  ( -24.24874870218063450, -26.64985754041175525, 6.700000000000000178 ) ) ;
#2643=CARTESIAN_POINT ( 'NONE',  ( -31.07867591359219617, -26.64985754041175525, 6.800000000000000711 ) ) ;
#2654=LINE ( 'NONE', #25067, #28202 ) ;
#2656=DIRECTION ( 'NONE',  ( 0.000000000000000000, 0.000000000000000000, 1.000000000000000000 ) ) ;
#2660=CIRCLE ( 'NONE', #9179, 0.1000000000000028644 ) ;
#2663=CARTESIAN_POINT ( 'NONE',  ( -12.44874870218064267, -26.64985754041175525, 6.800000000000000711 ) ) ;
#2669=FACE_OUTER_BOUND ( 'NONE', #24846, .T. ) ;
#2670=CARTESIAN_POINT ( 'NONE',  ( -32.24874870218063450, -25.49307895267003587, 6.800000000000000711 ) ) ;
#2687=PLANE ( 'NONE',  #5345 ) ;
#2692=EDGE_CURVE ( 'NONE', #18497, #35180, #36018, .T. ) ;
#2693=VERTEX_POINT ( 'NONE', #8956 ) ;
#2698=VERTEX_POINT ( 'NONE', #18225 ) ;
#2705=CARTESIAN_POINT ( 'NONE',  ( -22.24874870218063094, -26.64985754041175525, 6.800000000000000711 ) ) ;
#2710=ORIENTED_EDGE ( 'NONE', *, *, #14447, .F. ) ;
#2713=ORIENTED_EDGE ( 'NONE', *, *, #16177, .T. ) ;
#2714=ORIENTED_EDGE ( 'NONE', *, *, #3312, .F. ) ;
#2718=AXIS2_PLACEMENT_3D ( 'NONE', #26055, #337, #6713 ) ;
#2725=FACE_OUTER_BOUND ( 'NONE', #4617, .T. ) ;
#2729=VERTEX_POINT ( 'NONE', #21541 ) ;
#2734=LINE ( 'NONE', #30105, #10837 ) ;
#2735=EDGE_LOOP ( 'NONE', ( #2713, #31186, #38254, #24909 ) ) ;
#2743=ORIENTED_EDGE ( 'NONE', *, *, #11848, .T. ) ;
#2756=CIRCLE ( 'NONE', #17813, 0.1000000000000028644 ) ;
#2757=EDGE_LOOP ( 'NONE', ( #4590, #16075, #13154, #2079 ) ) ;
#2762=ADVANCED_FACE ( 'NONE', ( #17811 ), #18848, .F. ) ;
#2767=DIRECTION ( 'NONE',  ( 1.000000000000000000, 0.000000000000000000, 0.000000000000000000 ) ) ;
#2768=CARTESIAN_POINT ( 'NONE',  ( -20.34874870218063947, -25.49307895267003587, 6.700000000000000178 ) ) ;
#2769=FACE_OUTER_BOUND ( 'NONE', #7988, .T. ) ;
#2775=CYLINDRICAL_SURFACE ( 'NONE', #5545, 0.1000000000000028644 ) ;
#2776=LINE ( 'NONE', #2988, #4179 ) ;
#2777=CARTESIAN_POINT ( 'NONE',  ( -30.97867591359219119, -26.64985754041175525, 6.700000000000000178 ) ) ;
#2783=LINE ( 'NONE', #92, #29740 ) ;
#2784=VERTEX_POINT ( 'NONE', #15763 ) ;
#2785=DIRECTION ( 'NONE',  ( 1.000000000000000000, 0.000000000000000000, 0.000000000000000000 ) ) ;
#2787=ORIENTED_EDGE ( 'NONE', *, *, #38252, .F. ) ;
#2791=EDGE_CURVE ( 'NONE', #34298, #15456, #334, .T. ) ;
#2795=DIRECTION ( 'NONE',  ( -0.000000000000000000, -1.000000000000000000, -0.000000000000000000 ) ) ;
#2798=DIRECTION ( 'NONE',  ( 0.000000000000000000, 1.000000000000000000, 0.000000000000000000 ) ) ;
#2804=ORIENTED_EDGE ( 'NONE', *, *, #10458, .F. ) ;
#2807=DIRECTION ( 'NONE',  ( -1.000000000000000000, 0.000000000000000000, 0.000000000000000000 ) ) ;
#2810=ORIENTED_EDGE ( 'NONE', *, *, #3895, .T. ) ;
#2819=DIRECTION ( 'NONE',  ( 1.000000000000000000, 0.000000000000000000, 0.000000000000000000 ) ) ;
#2821=EDGE_CURVE ( 'NONE', #15366, #19353, #12874, .T. ) ;
#2826=FACE_OUTER_BOUND ( 'NONE', #30564, .T. ) ;
#2836=EDGE_CURVE ( 'NONE', #29646, #9655, #23675, .T. ) ;
#2843=ORIENTED_EDGE ( 'NONE', *, *, #13113, .F. ) ;
#2853=EDGE_CURVE ( 'NONE', #28333, #35369, #3846, .T. ) ;
#2870=VERTEX_POINT ( 'NONE', #12666 ) ;
#2873=EDGE_CURVE ( 'NONE', #699, #18231, #22, .T. ) ;
#2877=CARTESIAN_POINT ( 'NONE',  ( -26.44874870218064089, -25.49307895267003587, 6.700000000000000178 ) ) ;
#2882=ORIENTED_EDGE ( 'NONE', *, *, #26330, .T. ) ;
#2886=EDGE_CURVE ( 'NONE', #7569, #10217, #33549, .T. ) ;
#2890=EDGE_LOOP ( 'NONE', ( #24900, #29553, #8918, #31388 ) ) ;
#2892=EDGE_LOOP ( 'NONE', ( #752, #2843, #31101, #8869 ) ) ;
#2893=AXIS2_PLACEMENT_3D ( 'NONE', #6882, #28906, #25819 ) ;
#2894=ORIENTED_EDGE ( 'NONE', *, *, #5735, .F. ) ;
#2900=VERTEX_POINT ( 'NONE', #10181 ) ;
#2912=CARTESIAN_POINT ( 'NONE',  ( 7.121324086407810228, -26.64985754041175525, 6.800000000000000711 ) ) ;
#2914=ADVANCED_FACE ( 'NONE', ( #17160 ), #29137, .F. ) ;
#2921=EDGE_CURVE ( 'NONE', #37024, #36180, #4023, .T. ) ;
#2924=VECTOR ( 'NONE', #30398, 1000.000000000000000 ) ;
#2927=ADVANCED_FACE ( 'NONE', ( #23160 ), #23562, .T. ) ;
#2933=FACE_OUTER_BOUND ( 'NONE', #10768, .T. ) ;
#2939=CARTESIAN_POINT ( 'NONE',  ( -29.07867591359219617, -26.64985754041175525, 6.700000000000000178 ) ) ;
#2940=ORIENTED_EDGE ( 'NONE', *, *, #7153, .T. ) ;
#2944=VERTEX_POINT ( 'NONE', #38584 ) ;
#2948=ORIENTED_EDGE ( 'NONE', *, *, #17006, .T. ) ;
#2951=VERTEX_POINT ( 'NONE', #10390 ) ;
#2954=PLANE ( 'NONE',  #20224 ) ;
#2960=CARTESIAN_POINT ( 'NONE',  ( 1.551251297819356001, -26.64985754041175525, 6.700000000000000178 ) ) ;
#2979=CARTESIAN_POINT ( 'NONE',  ( 5.751251297819365504, -26.64985754041175525, 6.800000000000000711 ) ) ;
#2981=ADVANCED_FACE ( 'NONE', ( #4231 ), #39188, .F. ) ;
#2988=CARTESIAN_POINT ( 'NONE',  ( -28.87867591359218977, -24.55319635012989110, 6.700000000000000178 ) ) ;
#2989=DIRECTION ( 'NONE',  ( -1.000000000000000000, 0.000000000000000000, 0.000000000000000000 ) ) ;
#2991=FACE_OUTER_BOUND ( 'NONE', #3896, .T. ) ;
#2994=AXIS2_PLACEMENT_3D ( 'NONE', #26694, #30179, #11019 ) ;
#3003=DIRECTION ( 'NONE',  ( -0.000000000000000000, -1.000000000000000000, -0.000000000000000000 ) ) ;
#3005=FACE_OUTER_BOUND ( 'NONE', #40567, .T. ) ;
#3009=FACE_OUTER_BOUND ( 'NONE', #16422, .T. ) ;
#3017=CIRCLE ( 'NONE', #26005, 0.1000000000000028644 ) ;
#3018=DIRECTION ( 'NONE',  ( -1.000000000000000000, 0.000000000000000000, 0.000000000000000000 ) ) ;
#3020=CARTESIAN_POINT ( 'NONE',  ( -36.44874870218064444, -25.49307895267003587, 6.800000000000000711 ) ) ;
#3022=CARTESIAN_POINT ( 'NONE',  ( -28.24874870218063805, -25.49307895267003587, 6.700000000000000178 ) ) ;
#3026=AXIS2_PLACEMENT_3D ( 'NONE', #14948, #11231, #40066 ) ;
#3033=LINE ( 'NONE', #31212, #6500 ) ;
#3042=ORIENTED_EDGE ( 'NONE', *, *, #26643, .F. ) ;
#3048=VECTOR ( 'NONE', #16281, 1000.000000000000000 ) ;
#3050=DIRECTION ( 'NONE',  ( 1.000000000000000000, 0.000000000000000000, 0.000000000000000000 ) ) ;
#3052=ORIENTED_EDGE ( 'NONE', *, *, #12468, .T. ) ;
#3061=CARTESIAN_POINT ( 'NONE',  ( -34.34874870218063592, -25.49307895267003587, 6.800000000000000711 ) ) ;
#3065=CARTESIAN_POINT ( 'NONE',  ( -18.34874870218063947, -26.64985754041175525, 6.700000000000000178 ) ) ;
#3067=DIRECTION ( 'NONE',  ( 0.000000000000000000, 0.000000000000000000, 1.000000000000000000 ) ) ;
#3068=ORIENTED_EDGE ( 'NONE', *, *, #28132, .F. ) ;
#3069=EDGE_CURVE ( 'NONE', #4028, #40382, #32262, .T. ) ;
#3076=VERTEX_POINT ( 'NONE', #11584 ) ;
#3082=CARTESIAN_POINT ( 'NONE',  ( -6.448748702180637338, -25.49307895267003587, 6.800000000000000711 ) ) ;
#3084=DIRECTION ( 'NONE',  ( 0.000000000000000000, 0.000000000000000000, 1.000000000000000000 ) ) ;
#3088=ORIENTED_EDGE ( 'NONE', *, *, #8921, .T. ) ;
#3092=CARTESIAN_POINT ( 'NONE',  ( -26.24874870218063450, -26.64985754041175525, 6.700000000000000178 ) ) ;
#3093=VERTEX_POINT ( 'NONE', #21702 ) ;
#3095=EDGE_CURVE ( 'NONE', #17020, #3093, #14479, .T. ) ;
#3097=ORIENTED_EDGE ( 'NONE', *, *, #6200, .T. ) ;
#3101=VERTEX_POINT ( 'NONE', #21288 ) ;
#3112=AXIS2_PLACEMENT_3D ( 'NONE', #38420, #10221, #7739 ) ;
#3116=CIRCLE ( 'NONE', #34051, 0.1000000000000028644 ) ;
#3119=DIRECTION ( 'NONE',  ( 1.000000000000000000, 0.000000000000000000, 0.000000000000000000 ) ) ;
#3121=FACE_OUTER_BOUND ( 'NONE', #16633, .T. ) ;
#3126=ORIENTED_EDGE ( 'NONE', *, *, #16718, .F. ) ;
#3132=DIRECTION ( 'NONE',  ( 0.000000000000000000, 1.000000000000000000, 0.000000000000000000 ) ) ;
#3136=ORIENTED_EDGE ( 'NONE', *, *, #2345, .T. ) ;
#3139=AXIS2_PLACEMENT_3D ( 'NONE', #13570, #7789, #3936 ) ;
#3145=AXIS2_PLACEMENT_3D ( 'NONE', #32185, #12812, #28876 ) ;
#3147=CARTESIAN_POINT ( 'NONE',  ( -9.078675913592196167, -24.55319635012989110, 6.700000000000000178 ) ) ;
#3148=ORIENTED_EDGE ( 'NONE', *, *, #13426, .F. ) ;
#3159=FACE_BOUND ( 'NONE', #38953, .T. ) ;
#3163=EDGE_CURVE ( 'NONE', #12201, #3101, #8559, .T. ) ;
#3165=DIRECTION ( 'NONE',  ( 1.000000000000000000, -0.000000000000000000, 0.000000000000000000 ) ) ;
#3167=EDGE_CURVE ( 'NONE', #40638, #37085, #34918, .T. ) ;
#3168=FACE_OUTER_BOUND ( 'NONE', #28355, .T. ) ;
#3169=VERTEX_POINT ( 'NONE', #23311 ) ;
#3190=CARTESIAN_POINT ( 'NONE',  ( -18.44874870218064089, -26.64985754041175525, 6.700000000000000178 ) ) ;
#3193=CARTESIAN_POINT ( 'NONE',  ( -6.248748702180631831, -26.64985754041175525, 6.700000000000000178 ) ) ;
#3196=DIRECTION ( 'NONE',  ( 1.000000000000000000, -0.000000000000000000, 0.000000000000000000 ) ) ;
#3200=VECTOR ( 'NONE', #2455, 1000.000000000000000 ) ;
#3230=PLANE ( 'NONE',  #27251 ) ;
#3243=CARTESIAN_POINT ( 'NONE',  ( -10.34874870218063769, -26.64985754041175525, 6.700000000000000178 ) ) ;
#3257=ORIENTED_EDGE ( 'NONE', *, *, #36684, .T. ) ;
#3261=VECTOR ( 'NONE', #12879, 1000.000000000000000 ) ;
#3263=CARTESIAN_POINT ( 'NONE',  ( 6.921324086407803833, -26.64985754041175525, 6.700000000000000178 ) ) ;
#3294=DIRECTION ( 'NONE',  ( 0.000000000000000000, 0.000000000000000000, 1.000000000000000000 ) ) ;
#3300=EDGE_CURVE ( 'NONE', #25120, #25461, #5379, .T. ) ;
#3302=CIRCLE ( 'NONE', #5912, 0.1000000000000028644 ) ;
#3303=ORIENTED_EDGE ( 'NONE', *, *, #38854, .T. ) ;
#3309=EDGE_LOOP ( 'NONE', ( #36708, #38314, #1720, #31914 ) ) ;
#3311=VERTEX_POINT ( 'NONE', #33604 ) ;
#3312=EDGE_CURVE ( 'NONE', #23027, #9241, #5790, .T. ) ;
#3321=CYLINDRICAL_SURFACE ( 'NONE', #25271, 0.1000000000000028644 ) ;
#3330=EDGE_CURVE ( 'NONE', #13148, #20646, #6623, .T. ) ;
#3332=VECTOR ( 'NONE', #34733, 1000.000000000000000 ) ;
#3338=CARTESIAN_POINT ( 'NONE',  ( -4.878675913592187108, -26.64985754041175525, 6.800000000000000711 ) ) ;
#3342=DIRECTION ( 'NONE',  ( 0.000000000000000000, 1.000000000000000000, 0.000000000000000000 ) ) ;
#3346=EDGE_CURVE ( 'NONE', #33732, #3833, #33188, .T. ) ;
#3358=VECTOR ( 'NONE', #29635, 1000.000000000000000 ) ;
#3359=CARTESIAN_POINT ( 'NONE',  ( -14.24874870218063450, -26.64985754041175525, 6.700000000000000178 ) ) ;
#3362=ADVANCED_FACE ( 'NONE', ( #2725 ), #36464, .F. ) ;
#3364=DIRECTION ( 'NONE',  ( -0.000000000000000000, -0.000000000000000000, 1.000000000000000000 ) ) ;
#3378=EDGE_CURVE ( 'NONE', #30874, #38045, #17111, .T. ) ;
#3379=CARTESIAN_POINT ( 'NONE',  ( -51.21549048184568420, -30.38627270959228710, 4.000000000000000000 ) ) ;
#3386=DIRECTION ( 'NONE',  ( 1.000000000000000000, 0.000000000000000000, 0.000000000000000000 ) ) ;
#3391=CARTESIAN_POINT ( 'NONE',  ( -34.24874870218063450, -26.64985754041175525, 6.800000000000000711 ) ) ;
#3398=LINE ( 'NONE', #34886, #229 ) ;
#3402=EDGE_CURVE ( 'NONE', #408, #14576, #40133, .T. ) ;
#3406=EDGE_LOOP ( 'NONE', ( #32169, #39923, #28166, #25877 ) ) ;
#3410=ORIENTED_EDGE ( 'NONE', *, *, #4155, .F. ) ;
#3414=CARTESIAN_POINT ( 'NONE',  ( -37.07867591359219261, -26.64985754041175525, 6.700000000000000178 ) ) ;
#3424=LINE ( 'NONE', #12444, #7899 ) ;
#3427=EDGE_CURVE ( 'NONE', #15456, #160, #48, .T. ) ;
#3432=LINE ( 'NONE', #29125, #39737 ) ;
#3437=DIRECTION ( 'NONE',  ( -0.000000000000000000, -0.000000000000000000, 1.000000000000000000 ) ) ;
#3447=EDGE_CURVE ( 'NONE', #19353, #20724, #23052, .T. ) ;
#3448=EDGE_CURVE ( 'NONE', #17630, #38045, #5583, .T. ) ;
#3453=DIRECTION ( 'NONE',  ( 0.000000000000000000, 0.000000000000000000, 1.000000000000000000 ) ) ;
#3474=CARTESIAN_POINT ( 'NONE',  ( 1.121324086407811338, -24.55319635012989110, 6.700000000000000178 ) ) ;
#3476=ORIENTED_EDGE ( 'NONE', *, *, #11914, .F. ) ;
#3477=CARTESIAN_POINT ( 'NONE',  ( -16.44874870218064089, -26.64985754041175525, 6.800000000000000711 ) ) ;
#3478=LINE ( 'NONE', #33592, #20811 ) ;
#3486=ORIENTED_EDGE ( 'NONE', *, *, #17233, .F. ) ;
#3489=EDGE_CURVE ( 'NONE', #513, #650, #9901, .T. ) ;
#3492=EDGE_CURVE ( 'NONE', #31820, #30682, #34836, .T. ) ;
#3493=CARTESIAN_POINT ( 'NONE',  ( -2.978675913592195190, -26.64985754041175525, 6.800000000000000711 ) ) ;
#3494=CARTESIAN_POINT ( 'NONE',  ( -8.348748702180635917, -26.64985754041175525, 6.700000000000000178 ) ) ;
#3498=ORIENTED_EDGE ( 'NONE', *, *, #20216, .T. ) ;
#3504=FACE_OUTER_BOUND ( 'NONE', #26138, .T. ) ;
#3524=VERTEX_POINT ( 'NONE', #3742 ) ;
#3528=CARTESIAN_POINT ( 'NONE',  ( 11.65737507970504439, -29.56993018339339940, 6.000000000000000000 ) ) ;
#3531=ORIENTED_EDGE ( 'NONE', *, *, #10084, .T. ) ;
#3541=CIRCLE ( 'NONE', #10089, 0.1000000000000028644 ) ;
#3545=ORIENTED_EDGE ( 'NONE', *, *, #17006, .F. ) ;
#3553=DIRECTION ( 'NONE',  ( 1.000000000000000000, 0.000000000000000000, 0.000000000000000000 ) ) ;
#3569=ORIENTED_EDGE ( 'NONE', *, *, #24702, .F. ) ;
#3574=CIRCLE ( 'NONE', #4234, 0.1000000000000028644 ) ;
#3583=FACE_OUTER_BOUND ( 'NONE', #12150, .T. ) ;
#3586=DIRECTION ( 'NONE',  ( 0.000000000000000000, 0.000000000000000000, 1.000000000000000000 ) ) ;
#3590=AXIS2_PLACEMENT_3D ( 'NONE', #23486, #17281, #20381 ) ;
#3598=VERTEX_POINT ( 'NONE', #23066 ) ;
#3601=EDGE_LOOP ( 'NONE', ( #37257, #11839, #2804, #30674 ) ) ;
#3608=DIRECTION ( 'NONE',  ( 1.000000000000000000, 0.000000000000000000, 0.000000000000000000 ) ) ;
#3609=ORIENTED_EDGE ( 'NONE', *, *, #7770, .T. ) ;
#3615=ORIENTED_EDGE ( 'NONE', *, *, #37587, .T. ) ;
#3622=ORIENTED_EDGE ( 'NONE', *, *, #38845, .F. ) ;
#3627=ORIENTED_EDGE ( 'NONE', *, *, #26001, .T. ) ;
#3633=VECTOR ( 'NONE', #35875, 1000.000000000000000 ) ;
#3641=CARTESIAN_POINT ( 'NONE',  ( -30.34874870218063947, -26.64985754041175525, 6.700000000000000178 ) ) ;
#3642=CARTESIAN_POINT ( 'NONE',  ( -30.34874870218063947, -26.64985754041175525, 6.800000000000000711 ) ) ;
#3646=DIRECTION ( 'NONE',  ( -0.000000000000000000, -1.000000000000000000, -0.000000000000000000 ) ) ;
#3654=EDGE_CURVE ( 'NONE', #13108, #18315, #10536, .T. ) ;
#3657=VERTEX_POINT ( 'NONE', #26550 ) ;
#3658=AXIS2_PLACEMENT_3D ( 'NONE', #36462, #5377, #8237 ) ;
#3660=EDGE_CURVE ( 'NONE', #2270, #27725, #32936, .T. ) ;
#3663=AXIS2_PLACEMENT_3D ( 'NONE', #7452, #13230, #35679 ) ;
#3664=CARTESIAN_POINT ( 'NONE',  ( -40.97867591359219119, -26.64985754041175525, 6.700000000000000178 ) ) ;
#3668=ORIENTED_EDGE ( 'NONE', *, *, #57, .F. ) ;
#3669=EDGE_CURVE ( 'NONE', #12826, #5793, #19960, .T. ) ;
#3672=EDGE_CURVE ( 'NONE', #3169, #15928, #20158, .T. ) ;
#3673=CARTESIAN_POINT ( 'NONE',  ( -23.07867591359219617, -24.55319635012989110, 6.700000000000000178 ) ) ;
#3677=VERTEX_POINT ( 'NONE', #844 ) ;
#3689=ORIENTED_EDGE ( 'NONE', *, *, #36684, .F. ) ;
#3691=AXIS2_PLACEMENT_3D ( 'NONE', #39772, #12383, #36683 ) ;
#3695=DIRECTION ( 'NONE',  ( 1.000000000000000000, 0.000000000000000000, -0.000000000000000000 ) ) ;
#3698=CIRCLE ( 'NONE', #37186, 0.1000000000000028644 ) ;
#3699=EDGE_CURVE ( 'NONE', #2951, #9053, #26343, .T. ) ;
#3706=FACE_OUTER_BOUND ( 'NONE', #25613, .T. ) ;
#3710=ORIENTED_EDGE ( 'NONE', *, *, #34804, .F. ) ;
#3713=FACE_OUTER_BOUND ( 'NONE', #630, .T. ) ;
#3715=VERTEX_POINT ( 'NONE', #20357 ) ;
#3740=DIRECTION ( 'NONE',  ( 1.000000000000000000, 0.000000000000000000, 0.000000000000000000 ) ) ;
#3742=CARTESIAN_POINT ( 'NONE',  ( -22.24874870218063450, -26.64985754041175525, 6.700000000000000178 ) ) ;
#3743=CARTESIAN_POINT ( 'NONE',  ( -32.24874870218063450, -25.49307895267003587, 6.700000000000000178 ) ) ;
#3749=FACE_OUTER_BOUND ( 'NONE', #22002, .T. ) ;
#3753=AXIS2_PLACEMENT_3D ( 'NONE', #2091, #24084, #14212 ) ;
#3756=ORIENTED_EDGE ( 'NONE', *, *, #15718, .T. ) ;
#3757=FACE_BOUND ( 'NONE', #36746, .T. ) ;
#3761=CARTESIAN_POINT ( 'NONE',  ( -28.44874870218064444, -25.49307895267003587, 6.700000000000000178 ) ) ;
#3762=EDGE_CURVE ( 'NONE', #27559, #34769, #8591, .T. ) ;
#3763=EDGE_LOOP ( 'NONE', ( #7650, #7726, #6876, #28087 ) ) ;
#3771=VERTEX_POINT ( 'NONE', #37021 ) ;
#3772=EDGE_LOOP ( 'NONE', ( #28412, #31133, #9049, #3622 ) ) ;
#3781=VECTOR ( 'NONE', #38443, 1000.000000000000000 ) ;
#3787=CARTESIAN_POINT ( 'NONE',  ( 4.921324086407802056, -26.64985754041175525, 6.700000000000000178 ) ) ;
#3795=LINE ( 'NONE', #19417, #35566 ) ;
#3800=EDGE_CURVE ( 'NONE', #18519, #31377, #13143, .T. ) ;
#3801=ORIENTED_EDGE ( 'NONE', *, *, #23984, .F. ) ;
#3808=VECTOR ( 'NONE', #39803, 1000.000000000000000 ) ;
#3811=VERTEX_POINT ( 'NONE', #34793 ) ;
#3815=ORIENTED_EDGE ( 'NONE', *, *, #11270, .F. ) ;
#3819=ORIENTED_EDGE ( 'NONE', *, *, #34391, .F. ) ;
#3830=DIRECTION ( 'NONE',  ( 0.000000000000000000, 0.000000000000000000, 1.000000000000000000 ) ) ;
#3833=VERTEX_POINT ( 'NONE', #9848 ) ;
#3835=CARTESIAN_POINT ( 'NONE',  ( -20.87867591359218977, -24.55319635012989110, 6.800000000000000711 ) ) ;
#3846=LINE ( 'NONE', #35131, #7227 ) ;
#3855=EDGE_CURVE ( 'NONE', #25870, #36487, #23079, .T. ) ;
#3858=CARTESIAN_POINT ( 'NONE',  ( -1.078675913592196167, -26.64985754041175525, 6.700000000000000178 ) ) ;
#3863=CARTESIAN_POINT ( 'NONE',  ( -12.44874870218064267, -25.49307895267003587, 6.700000000000000178 ) ) ;
#3865=DIRECTION ( 'NONE',  ( -0.000000000000000000, -0.000000000000000000, 1.000000000000000000 ) ) ;
#3866=VERTEX_POINT ( 'NONE', #40508 ) ;
#3872=EDGE_LOOP ( 'NONE', ( #3689, #3486, #29987, #31844 ) ) ;
#3875=CARTESIAN_POINT ( 'NONE',  ( -22.44874870218064089, -26.64985754041175525, 6.700000000000000178 ) ) ;
#3881=ORIENTED_EDGE ( 'NONE', *, *, #35632, .F. ) ;
#3888=DIRECTION ( 'NONE',  ( 0.000000000000000000, 0.000000000000000000, 1.000000000000000000 ) ) ;
#3895=EDGE_CURVE ( 'NONE', #22787, #9079, #34183, .T. ) ;
#3896=EDGE_LOOP ( 'NONE', ( #15633, #1632, #6291, #8277 ) ) ;
#3897=CYLINDRICAL_SURFACE ( 'NONE', #13830, 2.500000000000002220 ) ;
#3901=CARTESIAN_POINT ( 'NONE',  ( 11.65737507970504439, -27.06993018339339940, 6.800000000000000711 ) ) ;
#3909=ORIENTED_EDGE ( 'NONE', *, *, #9581, .F. ) ;
#3930=ORIENTED_EDGE ( 'NONE', *, *, #18262, .T. ) ;
#3931=ORIENTED_EDGE ( 'NONE', *, *, #36941, .F. ) ;
#3932=AXIS2_PLACEMENT_3D ( 'NONE', #8235, #11127, #36264 ) ;
#3936=DIRECTION ( 'NONE',  ( 1.000000000000000000, 0.000000000000000000, 0.000000000000000000 ) ) ;
#3945=ORIENTED_EDGE ( 'NONE', *, *, #17399, .F. ) ;
#3946=DIRECTION ( 'NONE',  ( 1.000000000000000000, 0.000000000000000000, 0.000000000000000000 ) ) ;
#3949=CARTESIAN_POINT ( 'NONE',  ( 5.551251297819359110, -26.64985754041175525, 6.700000000000000178 ) ) ;
#3952=ORIENTED_EDGE ( 'NONE', *, *, #38992, .F. ) ;
#3962=FACE_BOUND ( 'NONE', #16065, .T. ) ;
#3964=ORIENTED_EDGE ( 'NONE', *, *, #3660, .F. ) ;
#3967=VECTOR ( 'NONE', #18154, 1000.000000000000000 ) ;
#3968=EDGE_LOOP ( 'NONE', ( #12840, #27144, #6953, #34302 ) ) ;
#3971=CARTESIAN_POINT ( 'NONE',  ( -40.97867591359219119, -24.55319635012989110, 6.700000000000000178 ) ) ;
#3974=DIRECTION ( 'NONE',  ( 0.000000000000000000, 0.000000000000000000, 1.000000000000000000 ) ) ;
#3995=DIRECTION ( 'NONE',  ( -0.000000000000000000, -1.000000000000000000, -0.000000000000000000 ) ) ;
#4000=CARTESIAN_POINT ( 'NONE',  ( -6.248748702180631831, -26.64985754041175525, 6.800000000000000711 ) ) ;
#4002=LINE ( 'NONE', #16520, #6221 ) ;
#4007=CARTESIAN_POINT ( 'NONE',  ( 5.121324086407808451, -24.55319635012989110, 6.700000000000000178 ) ) ;
#4023=CIRCLE ( 'NONE', #27001, 2.499999999999996891 ) ;
#4028=VERTEX_POINT ( 'NONE', #35194 ) ;
#4031=ADVANCED_FACE ( 'NONE', ( #32694 ), #19525, .F. ) ;
#4041=DIRECTION ( 'NONE',  ( -0.000000000000000000, -0.000000000000000000, 1.000000000000000000 ) ) ;
#4046=CARTESIAN_POINT ( 'NONE',  ( -40.97867591359219119, -26.64985754041175525, 6.800000000000000711 ) ) ;
#4052=AXIS2_PLACEMENT_3D ( 'NONE', #25499, #15615, #27965 ) ;
#4067=CARTESIAN_POINT ( 'NONE',  ( 1.121324086407811338, -26.64985754041175525, 6.700000000000000178 ) ) ;
#4076=DIRECTION ( 'NONE',  ( -0.000000000000000000, -0.000000000000000000, 1.000000000000000000 ) ) ;
#4088=FACE_OUTER_BOUND ( 'NONE', #21208, .T. ) ;
#4091=CARTESIAN_POINT ( 'NONE',  ( 5.551251297819359110, -25.49307895267003587, 6.700000000000000178 ) ) ;
#4092=EDGE_CURVE ( 'NONE', #5244, #28284, #2041, .T. ) ;
#4094=DIRECTION ( 'NONE',  ( -0.000000000000000000, -1.000000000000000000, -0.000000000000000000 ) ) ;
#4100=ORIENTED_EDGE ( 'NONE', *, *, #38297, .T. ) ;
#4101=DIRECTION ( 'NONE',  ( -1.000000000000000000, 0.000000000000000000, 0.000000000000000000 ) ) ;
#4102=ADVANCED_FACE ( 'NONE', ( #21142 ), #8146, .T. ) ;
#4107=DIRECTION ( 'NONE',  ( 0.000000000000000000, 0.000000000000000000, -1.000000000000000000 ) ) ;
#4109=VECTOR ( 'NONE', #24731, 1000.000000000000000 ) ;
#4113=DIRECTION ( 'NONE',  ( -0.000000000000000000, -0.000000000000000000, 1.000000000000000000 ) ) ;
#4115=DIRECTION ( 'NONE',  ( 0.000000000000000000, 0.000000000000000000, 1.000000000000000000 ) ) ;
#4118=FACE_OUTER_BOUND ( 'NONE', #13101, .T. ) ;
#4124=ORIENTED_EDGE ( 'NONE', *, *, #17105, .T. ) ;
#4127=LINE ( 'NONE', #2663, #8332 ) ;
#4129=FACE_OUTER_BOUND ( 'NONE', #15584, .T. ) ;
#4135=DIRECTION ( 'NONE',  ( 1.000000000000000000, 0.000000000000000000, 0.000000000000000000 ) ) ;
#4139=CARTESIAN_POINT ( 'NONE',  ( -15.07867591359219439, -24.55319635012989110, 6.700000000000000178 ) ) ;
#4140=AXIS2_PLACEMENT_3D ( 'NONE', #17782, #34902, #6266 ) ;
#4144=VERTEX_POINT ( 'NONE', #18646 ) ;
#4152=ORIENTED_EDGE ( 'NONE', *, *, #32289, .F. ) ;
#4155=EDGE_CURVE ( 'NONE', #10309, #8273, #5221, .T. ) ;
#4157=EDGE_CURVE ( 'NONE', #27773, #21932, #29647, .T. ) ;
#4158=CARTESIAN_POINT ( 'NONE',  ( 1.551251297819356001, -26.64985754041175525, 6.800000000000000711 ) ) ;
#4159=ORIENTED_EDGE ( 'NONE', *, *, #19877, .F. ) ;
#4165=AXIS2_PLACEMENT_3D ( 'NONE', #661, #38303, #22686 ) ;
#4168=CARTESIAN_POINT ( 'NONE',  ( -25.07867591359219617, -24.55319635012989110, 6.700000000000000178 ) ) ;
#4175=DIRECTION ( 'NONE',  ( -0.000000000000000000, -0.000000000000000000, 1.000000000000000000 ) ) ;
#4179=VECTOR ( 'NONE', #33858, 1000.000000000000000 ) ;
#4180=CARTESIAN_POINT ( 'NONE',  ( -32.44874870218063734, -26.64985754041175525, 6.700000000000000178 ) ) ;
#4194=DIRECTION ( 'NONE',  ( -0.000000000000000000, -0.000000000000000000, 1.000000000000000000 ) ) ;
#4213=LINE ( 'NONE', #23142, #19482 ) ;
#4214=EDGE_CURVE ( 'NONE', #35240, #7017, #18171, .T. ) ;
#4220=EDGE_LOOP ( 'NONE', ( #29010, #34951, #25458, #26842 ) ) ;
#4224=DIRECTION ( 'NONE',  ( -0.000000000000000000, -1.000000000000000000, -0.000000000000000000 ) ) ;
#4231=FACE_OUTER_BOUND ( 'NONE', #31859, .T. ) ;
#4232=AXIS2_PLACEMENT_3D ( 'NONE', #23405, #35581, #23014 ) ;
#4234=AXIS2_PLACEMENT_3D ( 'NONE', #39315, #38712, #39111 ) ;
#4241=AXIS2_PLACEMENT_3D ( 'NONE', #40332, #15841, #31299 ) ;
#4242=LINE ( 'NONE', #16766, #24136 ) ;
#4243=ORIENTED_EDGE ( 'NONE', *, *, #22801, .T. ) ;
#4248=ORIENTED_EDGE ( 'NONE', *, *, #11834, .F. ) ;
#4252=ORIENTED_EDGE ( 'NONE', *, *, #35132, .F. ) ;
#4257=CARTESIAN_POINT ( 'NONE',  ( 1.121324086407811338, -26.64985754041175525, 6.700000000000000178 ) ) ;
#4265=VERTEX_POINT ( 'NONE', #37115 ) ;
#4271=LINE ( 'NONE', #39016, #18168 ) ;
#4276=DIRECTION ( 'NONE',  ( 1.000000000000000000, -0.000000000000000000, 0.000000000000000000 ) ) ;
#4286=FACE_OUTER_BOUND ( 'NONE', #22251, .T. ) ;
#4287=AXIS2_PLACEMENT_3D ( 'NONE', #2046, #29624, #29430 ) ;
#4294=LINE ( 'NONE', #23612, #3781 ) ;
#4298=DIRECTION ( 'NONE',  ( 0.000000000000000000, 0.000000000000000000, 1.000000000000000000 ) ) ;
#4301=EDGE_CURVE ( 'NONE', #6453, #2951, #8287, .T. ) ;
#4305=CARTESIAN_POINT ( 'NONE',  ( -10.24874870218063450, -26.64985754041175525, 6.800000000000000711 ) ) ;
#4308=EDGE_LOOP ( 'NONE', ( #6577, #29939, #38675, #39208 ) ) ;
#4312=CARTESIAN_POINT ( 'NONE',  ( -6.978675913592191193, -26.64985754041175525, 6.800000000000000711 ) ) ;
#4313=DIRECTION ( 'NONE',  ( -0.000000000000000000, -0.000000000000000000, 1.000000000000000000 ) ) ;
#4320=AXIS2_PLACEMENT_3D ( 'NONE', #3092, #18276, #15609 ) ;
#4322=AXIS2_PLACEMENT_3D ( 'NONE', #14388, #15006, #21195 ) ;
#4324=DIRECTION ( 'NONE',  ( 1.000000000000000000, 0.000000000000000000, 0.000000000000000000 ) ) ;
#4329=VECTOR ( 'NONE', #5012, 1000.000000000000000 ) ;
#4339=CARTESIAN_POINT ( 'NONE',  ( -36.97867591359219119, -26.64985754041175525, 6.700000000000000178 ) ) ;
#4350=ORIENTED_EDGE ( 'NONE', *, *, #15951, .T. ) ;
#4351=VECTOR ( 'NONE', #19120, 1000.000000000000000 ) ;
#4360=DIRECTION ( 'NONE',  ( 1.000000000000000000, 0.000000000000000000, 0.000000000000000000 ) ) ;
#4362=ORIENTED_EDGE ( 'NONE', *, *, #2791, .T. ) ;
#4365=DIRECTION ( 'NONE',  ( 1.000000000000000000, 0.000000000000000000, 0.000000000000000000 ) ) ;
#4369=FACE_OUTER_BOUND ( 'NONE', #18702, .T. ) ;
#4370=PLANE ( 'NONE',  #14875 ) ;
#4372=DIRECTION ( 'NONE',  ( -0.000000000000000000, -1.000000000000000000, -0.000000000000000000 ) ) ;
#4379=CARTESIAN_POINT ( 'NONE',  ( -4.248748702180636272, -26.64985754041175525, 6.700000000000000178 ) ) ;
#4387=AXIS2_PLACEMENT_3D ( 'NONE', #27264, #33883, #12014 ) ;
#4390=CIRCLE ( 'NONE', #10298, 0.1000000000000028644 ) ;
#4391=CARTESIAN_POINT ( 'NONE',  ( -4.978675913592189417, -24.55319635012989110, 6.700000000000000178 ) ) ;
#4393=EDGE_LOOP ( 'NONE', ( #6668, #17644, #20082, #37851 ) ) ;
#4400=DIRECTION ( 'NONE',  ( -0.000000000000000000, -0.000000000000000000, 1.000000000000000000 ) ) ;
#4401=CARTESIAN_POINT ( 'NONE',  ( -10.87867591359219155, -24.55319635012989110, 6.800000000000000711 ) ) ;
#4405=FACE_OUTER_BOUND ( 'NONE', #21105, .T. ) ;
#4406=VERTEX_POINT ( 'NONE', #21890 ) ;
#4411=EDGE_LOOP ( 'NONE', ( #7261, #14166, #16448, #34763 ) ) ;
#4415=AXIS2_PLACEMENT_3D ( 'NONE', #37432, #16225, #25098 ) ;
#4418=AXIS2_PLACEMENT_3D ( 'NONE', #26393, #38923, #23294 ) ;
#4425=VERTEX_POINT ( 'NONE', #2979 ) ;
#4433=CARTESIAN_POINT ( 'NONE',  ( -20.44874870218064444, -26.64985754041175525, 6.800000000000000711 ) ) ;
#4435=DIRECTION ( 'NONE',  ( -0.000000000000000000, -0.000000000000000000, 1.000000000000000000 ) ) ;
#4441=ORIENTED_EDGE ( 'NONE', *, *, #2167, .F. ) ;
#4444=AXIS2_PLACEMENT_3D ( 'NONE', #38323, #10122, #34878 ) ;
#4446=AXIS2_PLACEMENT_3D ( 'NONE', #36574, #2429, #8353 ) ;
#4458=ORIENTED_EDGE ( 'NONE', *, *, #7264, .T. ) ;
#4474=CARTESIAN_POINT ( 'NONE',  ( -32.97867591359219119, -26.64985754041175525, 6.700000000000000178 ) ) ;
#4480=DIRECTION ( 'NONE',  ( 0.000000000000000000, 0.000000000000000000, -1.000000000000000000 ) ) ;
#4482=CARTESIAN_POINT ( 'NONE',  ( -11.07867591359219794, -24.55319635012989110, 6.700000000000000178 ) ) ;
#4485=VECTOR ( 'NONE', #38614, 1000.000000000000000 ) ;
#4490=CARTESIAN_POINT ( 'NONE',  ( -22.87867591359218977, -26.64985754041175525, 6.700000000000000178 ) ) ;
#4492=EDGE_CURVE ( 'NONE', #20522, #9487, #10929, .T. ) ;
#4500=VERTEX_POINT ( 'NONE', #23508 ) ;
#4504=DIRECTION ( 'NONE',  ( 1.000000000000000000, 0.000000000000000000, 0.000000000000000000 ) ) ;
#4507=ORIENTED_EDGE ( 'NONE', *, *, #11914, .T. ) ;
#4509=VECTOR ( 'NONE', #17851, 1000.000000000000000 ) ;
#4514=EDGE_CURVE ( 'NONE', #36371, #25629, #23732, .T. ) ;
#4517=DIRECTION ( 'NONE',  ( 0.000000000000000000, 1.000000000000000000, 0.000000000000000000 ) ) ;
#4521=ORIENTED_EDGE ( 'NONE', *, *, #15019, .F. ) ;
#4528=EDGE_CURVE ( 'NONE', #4832, #6790, #17102, .T. ) ;
#4536=DIRECTION ( 'NONE',  ( 0.000000000000000000, 0.000000000000000000, 1.000000000000000000 ) ) ;
#4538=AXIS2_PLACEMENT_3D ( 'NONE', #3971, #16292, #23092 ) ;
#4539=EDGE_CURVE ( 'NONE', #32235, #8986, #22906, .T. ) ;
#4543=LINE ( 'NONE', #17667, #14581 ) ;
#4546=ORIENTED_EDGE ( 'NONE', *, *, #33575, .F. ) ;
#4551=ORIENTED_EDGE ( 'NONE', *, *, #18980, .T. ) ;
#4559=CARTESIAN_POINT ( 'NONE',  ( -18.24874870218063450, -26.64985754041175525, 6.700000000000000178 ) ) ;
#4563=DIRECTION ( 'NONE',  ( 1.000000000000000000, 0.000000000000000000, 0.000000000000000000 ) ) ;
#4567=CARTESIAN_POINT ( 'NONE',  ( -16.97867591359219475, -24.55319635012989110, 6.700000000000000178 ) ) ;
#4572=EDGE_CURVE ( 'NONE', #28407, #3811, #25791, .T. ) ;
#4583=CARTESIAN_POINT ( 'NONE',  ( 5.751251297819365504, -25.49307895267003587, 6.700000000000000178 ) ) ;
#4585=VERTEX_POINT ( 'NONE', #33182 ) ;
#4590=ORIENTED_EDGE ( 'NONE', *, *, #24841, .T. ) ;
#4591=CARTESIAN_POINT ( 'NONE',  ( -15.07867591359219439, -26.64985754041175525, 6.700000000000000178 ) ) ;
#4592=DIRECTION ( 'NONE',  ( 0.000000000000000000, 1.000000000000000000, 0.000000000000000000 ) ) ;
#4602=CARTESIAN_POINT ( 'NONE',  ( -0.2487487021806331078, -26.64985754041175525, 6.800000000000000711 ) ) ;
#4603=ORIENTED_EDGE ( 'NONE', *, *, #28455, .F. ) ;
#4610=AXIS2_PLACEMENT_3D ( 'NONE', #5051, #32862, #39212 ) ;
#4617=EDGE_LOOP ( 'NONE', ( #34756, #10277, #8001, #23565 ) ) ;
#4620=ADVANCED_FACE ( 'NONE', ( #8851 ), #23886, .F. ) ;
#4622=ORIENTED_EDGE ( 'NONE', *, *, #14827, .T. ) ;
#4623=CARTESIAN_POINT ( 'NONE',  ( -14.97867591359219119, -26.64985754041175525, 6.700000000000000178 ) ) ;
#4625=ORIENTED_EDGE ( 'NONE', *, *, #37239, .F. ) ;
#4628=LINE ( 'NONE', #20452, #28830 ) ;
#4632=DIRECTION ( 'NONE',  ( 0.000000000000000000, 0.000000000000000000, 1.000000000000000000 ) ) ;
#4646=VECTOR ( 'NONE', #21031, 1000.000000000000000 ) ;
#4654=DIRECTION ( 'NONE',  ( 1.000000000000000000, 0.000000000000000000, 0.000000000000000000 ) ) ;
#4668=DIRECTION ( 'NONE',  ( -0.000000000000000000, -1.000000000000000000, -0.000000000000000000 ) ) ;
#4677=EDGE_LOOP ( 'NONE', ( #22942, #38986, #34738, #33814 ) ) ;
#4685=DIRECTION ( 'NONE',  ( 0.000000000000000000, 1.000000000000000000, 0.000000000000000000 ) ) ;
#4686=CARTESIAN_POINT ( 'NONE',  ( -10.44874870218064089, -26.64985754041175525, 6.700000000000000178 ) ) ;
#4692=CARTESIAN_POINT ( 'NONE',  ( -44.23414840393349579, -23.60493063168010153, 6.800000000000000711 ) ) ;
#4717=LINE ( 'NONE', #32928, #20366 ) ;
#4728=ORIENTED_EDGE ( 'NONE', *, *, #1875, .F. ) ;
#4733=CARTESIAN_POINT ( 'NONE',  ( -16.24874870218063450, -26.64985754041175525, 6.800000000000000711 ) ) ;
#4744=EDGE_CURVE ( 'NONE', #21196, #22883, #2756, .T. ) ;
#4746=ORIENTED_EDGE ( 'NONE', *, *, #11028, .T. ) ;
#4753=DIRECTION ( 'NONE',  ( 1.000000000000000000, 0.000000000000000000, 0.000000000000000000 ) ) ;
#4754=FACE_OUTER_BOUND ( 'NONE', #38298, .T. ) ;
#4761=CARTESIAN_POINT ( 'NONE',  ( -22.44874870218064089, -26.64985754041175525, 6.700000000000000178 ) ) ;
#4766=CARTESIAN_POINT ( 'NONE',  ( -7.078675913592194391, -26.64985754041175525, 6.700000000000000178 ) ) ;
#4790=EDGE_LOOP ( 'NONE', ( #8217, #38242, #16637, #40483 ) ) ;
#4805=DIRECTION ( 'NONE',  ( -0.000000000000000000, -0.000000000000000000, 1.000000000000000000 ) ) ;
#4808=CARTESIAN_POINT ( 'NONE',  ( -34.44874870218064444, -25.49307895267003587, 6.700000000000000178 ) ) ;
#4819=CARTESIAN_POINT ( 'NONE',  ( -35.07867591359219972, -26.64985754041175525, 6.700000000000000178 ) ) ;
#4822=DIRECTION ( 'NONE',  ( 1.000000000000000000, 0.000000000000000000, 0.000000000000000000 ) ) ;
#4823=FACE_OUTER_BOUND ( 'NONE', #17882, .T. ) ;
#4825=VECTOR ( 'NONE', #18143, 1000.000000000000000 ) ;
#4828=ORIENTED_EDGE ( 'NONE', *, *, #30544, .F. ) ;
#4831=CIRCLE ( 'NONE', #14654, 0.1000000000000028644 ) ;
#4832=VERTEX_POINT ( 'NONE', #1456 ) ;
#4839=EDGE_CURVE ( 'NONE', #33506, #35057, #11091, .T. ) ;
#4842=ORIENTED_EDGE ( 'NONE', *, *, #35132, .T. ) ;
#4847=FACE_OUTER_BOUND ( 'NONE', #37542, .T. ) ;
#4854=VECTOR ( 'NONE', #8552, 1000.000000000000000 ) ;
#4863=VECTOR ( 'NONE', #5598, 1000.000000000000000 ) ;
#4869=EDGE_CURVE ( 'NONE', #25288, #31282, #24273, .T. ) ;
#4881=AXIS2_PLACEMENT_3D ( 'NONE', #5832, #8280, #14872 ) ;
#4882=ADVANCED_FACE ( 'NONE', ( #24472 ), #21193, .F. ) ;
#4890=ORIENTED_EDGE ( 'NONE', *, *, #80, .F. ) ;
#4891=CIRCLE ( 'NONE', #6231, 2.500000000000002220 ) ;
#4892=PLANE ( 'NONE',  #31853 ) ;
#4893=CARTESIAN_POINT ( 'NONE',  ( -36.24874870218063450, -26.64985754041175525, 6.700000000000000178 ) ) ;
#4900=ORIENTED_EDGE ( 'NONE', *, *, #17343, .F. ) ;
#4906=DIRECTION ( 'NONE',  ( 0.000000000000000000, 0.000000000000000000, -1.000000000000000000 ) ) ;
#4907=ORIENTED_EDGE ( 'NONE', *, *, #28416, .T. ) ;
#4910=AXIS2_PLACEMENT_3D ( 'NONE', #5636, #18175, #30767 ) ;
#4911=AXIS2_PLACEMENT_3D ( 'NONE', #20494, #14318, #26888 ) ;
#4916=VECTOR ( 'NONE', #15508, 1000.000000000000000 ) ;
#4924=ORIENTED_EDGE ( 'NONE', *, *, #25531, .F. ) ;
#4930=VERTEX_POINT ( 'NONE', #23850 ) ;
#4932=ADVANCED_FACE ( 'NONE', ( #33975 ), #15004, .T. ) ;
#4934=EDGE_CURVE ( 'NONE', #863, #14484, #14790, .T. ) ;
#4935=VERTEX_POINT ( 'NONE', #39501 ) ;
#4940=ORIENTED_EDGE ( 'NONE', *, *, #31498, .F. ) ;
#4948=DIRECTION ( 'NONE',  ( -0.000000000000000000, -0.000000000000000000, 1.000000000000000000 ) ) ;
#4949=ORIENTED_EDGE ( 'NONE', *, *, #39881, .T. ) ;
#4957=VECTOR ( 'NONE', #11637, 1000.000000000000000 ) ;
#4959=DIRECTION ( 'NONE',  ( 1.000000000000000000, 0.000000000000000000, 0.000000000000000000 ) ) ;
#4961=DIRECTION ( 'NONE',  ( 1.000000000000000000, 0.000000000000000000, -0.000000000000000000 ) ) ;
#4973=LINE ( 'NONE', #17709, #10149 ) ;
#4977=DIRECTION ( 'NONE',  ( 0.000000000000000000, 0.000000000000000000, 1.000000000000000000 ) ) ;
#4978=CIRCLE ( 'NONE', #27982, 0.1000000000000028644 ) ;
#4984=CYLINDRICAL_SURFACE ( 'NONE', #7589, 0.1000000000000028644 ) ;
#4987=CARTESIAN_POINT ( 'NONE',  ( -25.07867591359219617, -26.64985754041175525, 6.700000000000000178 ) ) ;
#4989=LINE ( 'NONE', #32804, #14108 ) ;
#4992=DIRECTION ( 'NONE',  ( 1.000000000000000000, 0.000000000000000000, 0.000000000000000000 ) ) ;
#5005=ORIENTED_EDGE ( 'NONE', *, *, #9333, .F. ) ;
#5011=EDGE_CURVE ( 'NONE', #36027, #10700, #34327, .T. ) ;
#5012=DIRECTION ( 'NONE',  ( -0.000000000000000000, -0.000000000000000000, 1.000000000000000000 ) ) ;
#5017=LINE ( 'NONE', #20054, #3808 ) ;
#5023=DIRECTION ( 'NONE',  ( 0.000000000000000000, 0.000000000000000000, 1.000000000000000000 ) ) ;
#5028=ADVANCED_FACE ( 'NONE', ( #40120 ), #2687, .F. ) ;
#5041=VECTOR ( 'NONE', #37740, 1000.000000000000000 ) ;
#5046=CARTESIAN_POINT ( 'NONE',  ( -20.97867591359219475, -26.64985754041175525, 6.800000000000000711 ) ) ;
#5051=CARTESIAN_POINT ( 'NONE',  ( -8.978675913592192970, -26.64985754041175525, 6.700000000000000178 ) ) ;
#5055=DIRECTION ( 'NONE',  ( -0.000000000000000000, -0.000000000000000000, 1.000000000000000000 ) ) ;
#5060=AXIS2_PLACEMENT_3D ( 'NONE', #18013, #26884, #8543 ) ;
#5073=EDGE_CURVE ( 'NONE', #37085, #9686, #6771, .T. ) ;
#5076=DIRECTION ( 'NONE',  ( 0.000000000000000000, 0.000000000000000000, 1.000000000000000000 ) ) ;
#5089=VERTEX_POINT ( 'NONE', #28382 ) ;
#5101=DIRECTION ( 'NONE',  ( -0.000000000000000000, -0.000000000000000000, 1.000000000000000000 ) ) ;
#5103=DIRECTION ( 'NONE',  ( 0.000000000000000000, 1.000000000000000000, 0.000000000000000000 ) ) ;
#5105=CARTESIAN_POINT ( 'NONE',  ( -26.87867591359219333, -26.64985754041175525, 6.800000000000000711 ) ) ;
#5109=EDGE_CURVE ( 'NONE', #28333, #18637, #38050, .T. ) ;
#5117=AXIS2_PLACEMENT_3D ( 'NONE', #13719, #32667, #10011 ) ;
#5118=DIRECTION ( 'NONE',  ( 1.000000000000000000, 0.000000000000000000, 0.000000000000000000 ) ) ;
#5126=PLANE ( 'NONE',  #21569 ) ;
#5129=AXIS2_PLACEMENT_3D ( 'NONE', #36415, #8187, #26945 ) ;
#5134=CARTESIAN_POINT ( 'NONE',  ( -24.24874870218063450, -26.64985754041175525, 6.800000000000000711 ) ) ;
#5136=DIRECTION ( 'NONE',  ( 0.000000000000000000, 0.000000000000000000, -1.000000000000000000 ) ) ;
#5139=ORIENTED_EDGE ( 'NONE', *, *, #23602, .F. ) ;
#5141=LINE ( 'NONE', #22179, #335 ) ;
#5147=EDGE_LOOP ( 'NONE', ( #39421, #20925, #29885, #31121 ) ) ;
#5151=ORIENTED_EDGE ( 'NONE', *, *, #14720, .F. ) ;
#5155=DIRECTION ( 'NONE',  ( 1.000000000000000000, 0.000000000000000000, 0.000000000000000000 ) ) ;
#5159=ORIENTED_EDGE ( 'NONE', *, *, #33812, .T. ) ;
#5160=DIRECTION ( 'NONE',  ( 0.000000000000000000, 1.000000000000000000, 0.000000000000000000 ) ) ;
#5163=DIRECTION ( 'NONE',  ( -0.000000000000000000, -0.000000000000000000, 1.000000000000000000 ) ) ;
#5177=CARTESIAN_POINT ( 'NONE',  ( -36.87867591359218977, -26.64985754041175525, 6.800000000000000711 ) ) ;
#5179=DIRECTION ( 'NONE',  ( 0.000000000000000000, 0.000000000000000000, 1.000000000000000000 ) ) ;
#5181=CARTESIAN_POINT ( 'NONE',  ( 3.651251297819360531, -26.64985754041175525, 6.700000000000000178 ) ) ;
#5182=ORIENTED_EDGE ( 'NONE', *, *, #28685, .F. ) ;
#5188=ORIENTED_EDGE ( 'NONE', *, *, #34210, .T. ) ;
#5191=DIRECTION ( 'NONE',  ( 0.000000000000000000, 1.000000000000000000, 0.000000000000000000 ) ) ;
#5195=ORIENTED_EDGE ( 'NONE', *, *, #10863, .T. ) ;
#5199=VECTOR ( 'NONE', #12699, 1000.000000000000000 ) ;
#5219=AXIS2_PLACEMENT_3D ( 'NONE', #28928, #16551, #25632 ) ;
#5221=LINE ( 'NONE', #8904, #5314 ) ;
#5223=ADVANCED_FACE ( 'NONE', ( #38512 ), #10912, .F. ) ;
#5224=DIRECTION ( 'NONE',  ( 0.000000000000000000, 0.000000000000000000, 1.000000000000000000 ) ) ;
#5232=CARTESIAN_POINT ( 'NONE',  ( 5.021324086407805254, -24.55319635012989110, 6.700000000000000178 ) ) ;
#5238=PLANE ( 'NONE',  #14687 ) ;
#5243=CARTESIAN_POINT ( 'NONE',  ( -18.87867591359219333, -24.55319635012989110, 6.700000000000000178 ) ) ;
#5244=VERTEX_POINT ( 'NONE', #23680 ) ;
#5255=VECTOR ( 'NONE', #6690, 1000.000000000000000 ) ;
#5257=DIRECTION ( 'NONE',  ( 0.000000000000000000, 0.000000000000000000, 1.000000000000000000 ) ) ;
#5259=ORIENTED_EDGE ( 'NONE', *, *, #2873, .F. ) ;
#5261=DIRECTION ( 'NONE',  ( 1.000000000000000000, 0.000000000000000000, 0.000000000000000000 ) ) ;
#5265=DIRECTION ( 'NONE',  ( 1.000000000000000000, 0.000000000000000000, -0.000000000000000000 ) ) ;
#5280=ADVANCED_FACE ( 'NONE', ( #13405 ), #25979, .F. ) ;
#5284=AXIS2_PLACEMENT_3D ( 'NONE', #26803, #7453, #10729 ) ;
#5291=DIRECTION ( 'NONE',  ( -0.000000000000000000, -0.000000000000000000, 1.000000000000000000 ) ) ;
#5299=VERTEX_POINT ( 'NONE', #29659 ) ;
#5300=ADVANCED_FACE ( 'NONE', ( #1472 ), #14005, .F. ) ;
#5301=CIRCLE ( 'NONE', #28319, 0.1000000000000028644 ) ;
#5312=CARTESIAN_POINT ( 'NONE',  ( -4.448748702180642667, -26.64985754041175525, 6.700000000000000178 ) ) ;
#5314=VECTOR ( 'NONE', #24355, 1000.000000000000000 ) ;
#5315=CARTESIAN_POINT ( 'NONE',  ( -8.248748702180632719, -26.64985754041175525, 6.800000000000000711 ) ) ;
#5321=CARTESIAN_POINT ( 'NONE',  ( -18.87867591359219333, -26.64985754041175525, 6.700000000000000178 ) ) ;
#5330=ORIENTED_EDGE ( 'NONE', *, *, #24841, .F. ) ;
#5334=EDGE_LOOP ( 'NONE', ( #5182, #27575, #7327, #28510 ) ) ;
#5341=ORIENTED_EDGE ( 'NONE', *, *, #26282, .F. ) ;
#5345=AXIS2_PLACEMENT_3D ( 'NONE', #12105, #14386, #5136 ) ;
#5356=LINE ( 'NONE', #12122, #16059 ) ;
#5363=ORIENTED_EDGE ( 'NONE', *, *, #1726, .T. ) ;
#5377=DIRECTION ( 'NONE',  ( -1.000000000000000000, 0.000000000000000000, 0.000000000000000000 ) ) ;
#5379=LINE ( 'NONE', #8856, #5964 ) ;
#5382=DIRECTION ( 'NONE',  ( 0.000000000000000000, 0.000000000000000000, 1.000000000000000000 ) ) ;
#5391=EDGE_CURVE ( 'NONE', #11501, #26758, #2101, .T. ) ;
#5392=CARTESIAN_POINT ( 'NONE',  ( -18.44874870218064089, -25.49307895267003587, 6.700000000000000178 ) ) ;
#5395=DIRECTION ( 'NONE',  ( -0.000000000000000000, -0.000000000000000000, 1.000000000000000000 ) ) ;
#5402=EDGE_CURVE ( 'NONE', #40691, #2270, #39729, .T. ) ;
#5419=LINE ( 'NONE', #11569, #13437 ) ;
#5423=ORIENTED_EDGE ( 'NONE', *, *, #6943, .T. ) ;
#5425=DIRECTION ( 'NONE',  ( -0.000000000000000000, -0.000000000000000000, 1.000000000000000000 ) ) ;
#5428=CARTESIAN_POINT ( 'NONE',  ( -26.44874870218064089, -25.49307895267003587, 6.700000000000000178 ) ) ;
#5430=FACE_OUTER_BOUND ( 'NONE', #25314, .T. ) ;
#5434=CARTESIAN_POINT ( 'NONE',  ( 0.9213240864078056092, -24.55319635012989110, 6.700000000000000178 ) ) ;
#5435=DIRECTION ( 'NONE',  ( -0.000000000000000000, -1.000000000000000000, -0.000000000000000000 ) ) ;
#5437=ORIENTED_EDGE ( 'NONE', *, *, #14775, .T. ) ;
#5441=VECTOR ( 'NONE', #6477, 1000.000000000000000 ) ;
#5442=DIRECTION ( 'NONE',  ( -0.000000000000000000, -0.000000000000000000, 1.000000000000000000 ) ) ;
#5443=VERTEX_POINT ( 'NONE', #34202 ) ;
#5451=CARTESIAN_POINT ( 'NONE',  ( -42.44874870218064444, -26.64985754041175525, 6.700000000000000178 ) ) ;
#5453=CARTESIAN_POINT ( 'NONE',  ( -32.34874870218063592, -25.49307895267003587, 6.700000000000000178 ) ) ;
#5454=ADVANCED_FACE ( 'NONE', ( #28400 ), #34814, .F. ) ;
#5455=LINE ( 'NONE', #17785, #26064 ) ;
#5472=LINE ( 'NONE', #12462, #20278 ) ;
#5477=VECTOR ( 'NONE', #38979, 1000.000000000000000 ) ;
#5481=ORIENTED_EDGE ( 'NONE', *, *, #22427, .F. ) ;
#5486=CARTESIAN_POINT ( 'NONE',  ( -16.34874870218063592, -26.64985754041175525, 6.800000000000000711 ) ) ;
#5489=CARTESIAN_POINT ( 'NONE',  ( 1.121324086407811338, -26.64985754041175525, 6.800000000000000711 ) ) ;
#5490=DIRECTION ( 'NONE',  ( -0.000000000000000000, -0.000000000000000000, 1.000000000000000000 ) ) ;
#5495=EDGE_LOOP ( 'NONE', ( #9432, #29567, #37334, #13445 ) ) ;
#5508=DIRECTION ( 'NONE',  ( -0.000000000000000000, -0.000000000000000000, 1.000000000000000000 ) ) ;
#5512=PLANE ( 'NONE',  #32765 ) ;
#5521=ORIENTED_EDGE ( 'NONE', *, *, #10304, .F. ) ;
#5523=EDGE_CURVE ( 'NONE', #31377, #37191, #31501, .T. ) ;
#5530=VERTEX_POINT ( 'NONE', #37858 ) ;
#5534=VECTOR ( 'NONE', #37854, 1000.000000000000000 ) ;
#5537=EDGE_LOOP ( 'NONE', ( #33426, #26109, #21146, #39525, #33214 ) ) ;
#5544=CARTESIAN_POINT ( 'NONE',  ( 3.751251297819363728, -26.64985754041175525, 6.700000000000000178 ) ) ;
#5545=AXIS2_PLACEMENT_3D ( 'NONE', #40010, #14476, #9123 ) ;
#5555=ORIENTED_EDGE ( 'NONE', *, *, #16967, .T. ) ;
#5566=ADVANCED_FACE ( 'NONE', ( #25116 ), #34610, .F. ) ;
#5567=CARTESIAN_POINT ( 'NONE',  ( -30.24874870218063450, -26.64985754041175525, 6.700000000000000178 ) ) ;
#5573=CARTESIAN_POINT ( 'NONE',  ( -33.07867591359219972, -26.64985754041175525, 6.800000000000000711 ) ) ;
#5579=DIRECTION ( 'NONE',  ( 0.000000000000000000, -1.000000000000000000, 0.000000000000000000 ) ) ;
#5581=EDGE_CURVE ( 'NONE', #10252, #32142, #15843, .T. ) ;
#5582=EDGE_CURVE ( 'NONE', #30328, #29646, #9044, .T. ) ;
#5583=LINE ( 'NONE', #30714, #4646 ) ;
#5587=ORIENTED_EDGE ( 'NONE', *, *, #18430, .F. ) ;
#5594=VECTOR ( 'NONE', #7551, 1000.000000000000000 ) ;
#5598=DIRECTION ( 'NONE',  ( -0.000000000000000000, -0.000000000000000000, 1.000000000000000000 ) ) ;
#5601=DIRECTION ( 'NONE',  ( 0.000000000000000000, 0.000000000000000000, 1.000000000000000000 ) ) ;
#5604=LINE ( 'NONE', #30731, #15499 ) ;
#5605=CARTESIAN_POINT ( 'NONE',  ( 5.751251297819365504, -26.64985754041175525, 6.800000000000000711 ) ) ;
#5611=VERTEX_POINT ( 'NONE', #37450 ) ;
#5618=FACE_OUTER_BOUND ( 'NONE', #20905, .T. ) ;
#5624=DIRECTION ( 'NONE',  ( -0.000000000000000000, -0.000000000000000000, 1.000000000000000000 ) ) ;
#5631=CIRCLE ( 'NONE', #22722, 0.1000000000000028644 ) ;
#5633=EDGE_CURVE ( 'NONE', #650, #10252, #9247, .T. ) ;
#5636=CARTESIAN_POINT ( 'NONE',  ( -26.34874870218063947, -25.49307895267003587, 6.700000000000000178 ) ) ;
#5642=EDGE_CURVE ( 'NONE', #4832, #15795, #7378, .T. ) ;
#5644=DIRECTION ( 'NONE',  ( -0.000000000000000000, -0.000000000000000000, 1.000000000000000000 ) ) ;
#5648=ORIENTED_EDGE ( 'NONE', *, *, #40236, .F. ) ;
#5653=CARTESIAN_POINT ( 'NONE',  ( -6.978675913592191193, -26.64985754041175525, 6.700000000000000178 ) ) ;
#5657=DIRECTION ( 'NONE',  ( -0.000000000000000000, -1.000000000000000000, -0.000000000000000000 ) ) ;
#5661=AXIS2_PLACEMENT_3D ( 'NONE', #23400, #11424, #36364 ) ;
#5662=AXIS2_PLACEMENT_3D ( 'NONE', #19730, #23224, #25908 ) ;
#5663=EDGE_LOOP ( 'NONE', ( #32801, #30202, #33750, #22974 ) ) ;
#5670=LINE ( 'NONE', #18208, #23214 ) ;
#5680=CARTESIAN_POINT ( 'NONE',  ( -0.4487487021806388365, -25.49307895267003587, 6.700000000000000178 ) ) ;
#5681=DIRECTION ( 'NONE',  ( 0.000000000000000000, 0.000000000000000000, 1.000000000000000000 ) ) ;
#5690=AXIS2_PLACEMENT_3D ( 'NONE', #19486, #18867, #12686 ) ;
#5694=CIRCLE ( 'NONE', #3753, 0.1000000000000028644 ) ;
#5705=VERTEX_POINT ( 'NONE', #32126 ) ;
#5717=VECTOR ( 'NONE', #39706, 1000.000000000000000 ) ;
#5731=DIRECTION ( 'NONE',  ( -1.000000000000000000, 0.000000000000000000, 0.000000000000000000 ) ) ;
#5735=EDGE_CURVE ( 'NONE', #20646, #1547, #35212, .T. ) ;
#5739=CARTESIAN_POINT ( 'NONE',  ( 5.021324086407805254, -26.64985754041175525, 6.700000000000000178 ) ) ;
#5741=VERTEX_POINT ( 'NONE', #1427 ) ;
#5748=AXIS2_PLACEMENT_3D ( 'NONE', #1951, #7896, #20859 ) ;
#5749=DIRECTION ( 'NONE',  ( 0.000000000000000000, -0.000000000000000000, 1.000000000000000000 ) ) ;
#5751=EDGE_LOOP ( 'NONE', ( #40519, #36610, #36898, #6468 ) ) ;
#5753=ORIENTED_EDGE ( 'NONE', *, *, #32289, .T. ) ;
#5755=LINE ( 'NONE', #28542, #34558 ) ;
#5766=DIRECTION ( 'NONE',  ( 1.000000000000000000, 0.000000000000000000, 0.000000000000000000 ) ) ;
#5770=ORIENTED_EDGE ( 'NONE', *, *, #21819, .T. ) ;
#5773=EDGE_CURVE ( 'NONE', #2073, #26853, #6984, .T. ) ;
#5789=VERTEX_POINT ( 'NONE', #23238 ) ;
#5790=LINE ( 'NONE', #40355, #11847 ) ;
#5793=VERTEX_POINT ( 'NONE', #35609 ) ;
#5795=LINE ( 'NONE', #40361, #4109 ) ;
#5798=CARTESIAN_POINT ( 'NONE',  ( -0.3487487021806359722, -25.49307895267003587, 6.800000000000000711 ) ) ;
#5818=CARTESIAN_POINT ( 'NONE',  ( -14.24874870218063450, -26.64985754041175525, 6.700000000000000178 ) ) ;
#5819=ADVANCED_FACE ( 'NONE', ( #4118 ), #821, .F. ) ;
#5823=EDGE_CURVE ( 'NONE', #27773, #26423, #39061, .T. ) ;
#5825=VECTOR ( 'NONE', #34273, 1000.000000000000000 ) ;
#5829=VECTOR ( 'NONE', #17337, 1000.000000000000000 ) ;
#5832=CARTESIAN_POINT ( 'NONE',  ( -32.34874870218063592, -25.49307895267003587, 6.700000000000000178 ) ) ;
#5855=ORIENTED_EDGE ( 'NONE', *, *, #34299, .T. ) ;
#5858=EDGE_CURVE ( 'NONE', #21009, #37250, #30426, .T. ) ;
#5864=EDGE_CURVE ( 'NONE', #26146, #34445, #11457, .T. ) ;
#5872=DIRECTION ( 'NONE',  ( -0.000000000000000000, -1.000000000000000000, -0.000000000000000000 ) ) ;
#5876=AXIS2_PLACEMENT_3D ( 'NONE', #3190, #18378, #25181 ) ;
#5877=LINE ( 'NONE', #28093, #28062 ) ;
#5878=DIRECTION ( 'NONE',  ( 1.000000000000000000, 0.000000000000000000, -0.000000000000000000 ) ) ;
#5889=CARTESIAN_POINT ( 'NONE',  ( -0.2487487021806331078, -25.49307895267003587, 6.800000000000000711 ) ) ;
#5890=CARTESIAN_POINT ( 'NONE',  ( -10.34874870218063769, -25.49307895267003587, 6.700000000000000178 ) ) ;
#5900=AXIS2_PLACEMENT_3D ( 'NONE', #34352, #3067, #12282 ) ;
#5910=FACE_OUTER_BOUND ( 'NONE', #27777, .T. ) ;
#5911=ADVANCED_FACE ( 'NONE', ( #8583 ), #33729, .F. ) ;
#5912=AXIS2_PLACEMENT_3D ( 'NONE', #39931, #33573, #17273 ) ;
#5913=ORIENTED_EDGE ( 'NONE', *, *, #6200, .F. ) ;
#5922=ADVANCED_FACE ( 'NONE', ( #1831 ), #21162, .F. ) ;
#5928=CARTESIAN_POINT ( 'NONE',  ( -12.24874870218063627, -25.49307895267003587, 6.700000000000000178 ) ) ;
#5943=CARTESIAN_POINT ( 'NONE',  ( 5.021324086407805254, -26.64985754041175525, 6.700000000000000178 ) ) ;
#5945=DIRECTION ( 'NONE',  ( 1.000000000000000000, 0.000000000000000000, 0.000000000000000000 ) ) ;
#5951=CARTESIAN_POINT ( 'NONE',  ( -24.44874870218064089, -26.64985754041175525, 6.700000000000000178 ) ) ;
#5963=EDGE_CURVE ( 'NONE', #14079, #38489, #9989, .T. ) ;
#5964=VECTOR ( 'NONE', #24099, 1000.000000000000000 ) ;
#5966=EDGE_CURVE ( 'NONE', #16055, #32703, #39966, .T. ) ;
#5968=DIRECTION ( 'NONE',  ( 0.000000000000000000, 0.000000000000000000, -1.000000000000000000 ) ) ;
#5981=ORIENTED_EDGE ( 'NONE', *, *, #29570, .T. ) ;
#5982=CARTESIAN_POINT ( 'NONE',  ( -54.01549048184568846, -30.38627270959228710, 6.799999999999999822 ) ) ;
#5986=VECTOR ( 'NONE', #5435, 1000.000000000000000 ) ;
#5994=CIRCLE ( 'NONE', #13956, 0.1000000000000028644 ) ;
#6002=FACE_OUTER_BOUND ( 'NONE', #31807, .T. ) ;
#6003=VERTEX_POINT ( 'NONE', #8376 ) ;
#6006=ORIENTED_EDGE ( 'NONE', *, *, #10369, .F. ) ;
#6011=FACE_OUTER_BOUND ( 'NONE', #32748, .T. ) ;
#6027=ORIENTED_EDGE ( 'NONE', *, *, #15336, .T. ) ;
#6029=DIRECTION ( 'NONE',  ( -0.000000000000000000, -1.000000000000000000, -0.000000000000000000 ) ) ;
#6042=CARTESIAN_POINT ( 'NONE',  ( -14.24874870218063450, -25.49307895267003587, 6.800000000000000711 ) ) ;
#6049=FACE_OUTER_BOUND ( 'NONE', #23211, .T. ) ;
#6055=EDGE_CURVE ( 'NONE', #30629, #40311, #24864, .T. ) ;
#6056=PLANE ( 'NONE',  #33753 ) ;
#6059=EDGE_CURVE ( 'NONE', #31323, #3657, #24652, .T. ) ;
#6061=CARTESIAN_POINT ( 'NONE',  ( -20.34874870218063947, -26.64985754041175525, 6.700000000000000178 ) ) ;
#6062=VECTOR ( 'NONE', #17032, 1000.000000000000000 ) ;
#6065=AXIS2_PLACEMENT_3D ( 'NONE', #16273, #10095, #12988 ) ;
#6067=ORIENTED_EDGE ( 'NONE', *, *, #1096, .F. ) ;
#6073=LINE ( 'NONE', #28292, #15127 ) ;
#6080=DIRECTION ( 'NONE',  ( -0.000000000000000000, -0.000000000000000000, 1.000000000000000000 ) ) ;
#6094=DIRECTION ( 'NONE',  ( -0.000000000000000000, -1.000000000000000000, -0.000000000000000000 ) ) ;
#6100=ORIENTED_EDGE ( 'NONE', *, *, #15103, .T. ) ;
#6106=DIRECTION ( 'NONE',  ( 0.000000000000000000, 0.000000000000000000, 1.000000000000000000 ) ) ;
#6110=VERTEX_POINT ( 'NONE', #30848 ) ;
#6112=VECTOR ( 'NONE', #28962, 1000.000000000000000 ) ;
#6115=VERTEX_POINT ( 'NONE', #19087 ) ;
#6123=CARTESIAN_POINT ( 'NONE',  ( -26.24874870218063450, -25.49307895267003587, 6.800000000000000711 ) ) ;
#6132=ORIENTED_EDGE ( 'NONE', *, *, #33263, .F. ) ;
#6135=CARTESIAN_POINT ( 'NONE',  ( -4.348748702180639469, -26.64985754041175525, 6.700000000000000178 ) ) ;
#6139=EDGE_LOOP ( 'NONE', ( #28431, #9454, #31126, #36309 ) ) ;
#6141=CARTESIAN_POINT ( 'NONE',  ( -0.8786759135921904385, -26.64985754041175525, 6.700000000000000178 ) ) ;
#6147=PLANE ( 'NONE',  #39109 ) ;
#6152=EDGE_CURVE ( 'NONE', #29514, #3715, #10420, .T. ) ;
#6153=EDGE_CURVE ( 'NONE', #33795, #1662, #9074, .T. ) ;
#6155=ORIENTED_EDGE ( 'NONE', *, *, #35181, .F. ) ;
#6161=DIRECTION ( 'NONE',  ( 0.000000000000000000, 0.000000000000000000, 1.000000000000000000 ) ) ;
#6175=DIRECTION ( 'NONE',  ( 1.000000000000000000, 0.000000000000000000, 0.000000000000000000 ) ) ;
#6186=LINE ( 'NONE', #31310, #14249 ) ;
#6191=ORIENTED_EDGE ( 'NONE', *, *, #528, .F. ) ;
#6193=AXIS2_PLACEMENT_3D ( 'NONE', #11837, #39644, #36563 ) ;
#6198=LINE ( 'NONE', #12765, #25954 ) ;
#6200=EDGE_CURVE ( 'NONE', #35146, #23027, #35755, .T. ) ;
#6202=CARTESIAN_POINT ( 'NONE',  ( -16.97867591359219475, -26.64985754041175525, 6.700000000000000178 ) ) ;
#6203=ADVANCED_FACE ( 'NONE', ( #16198 ), #7531, .F. ) ;
#6205=ORIENTED_EDGE ( 'NONE', *, *, #12515, .F. ) ;
#6210=ORIENTED_EDGE ( 'NONE', *, *, #22675, .T. ) ;
#6215=FACE_BOUND ( 'NONE', #8974, .T. ) ;
#6216=DIRECTION ( 'NONE',  ( -1.000000000000000000, 0.000000000000000000, 0.000000000000000000 ) ) ;
#6221=VECTOR ( 'NONE', #36089, 1000.000000000000000 ) ;
#6226=LINE ( 'NONE', #18358, #16451 ) ;
#6230=ORIENTED_EDGE ( 'NONE', *, *, #17686, .T. ) ;
#6231=AXIS2_PLACEMENT_3D ( 'NONE', #40551, #28835, #3740 ) ;
#6232=CARTESIAN_POINT ( 'NONE',  ( -6.978675913592191193, -26.64985754041175525, 6.700000000000000178 ) ) ;
#6247=DIRECTION ( 'NONE',  ( -0.000000000000000000, -0.000000000000000000, 1.000000000000000000 ) ) ;
#6249=FACE_OUTER_BOUND ( 'NONE', #18452, .T. ) ;
#6251=LINE ( 'NONE', #9125, #29264 ) ;
#6253=DIRECTION ( 'NONE',  ( -1.000000000000000000, 0.000000000000000000, 0.000000000000000000 ) ) ;
#6255=CARTESIAN_POINT ( 'NONE',  ( -4.448748702180642667, -26.64985754041175525, 6.800000000000000711 ) ) ;
#6258=EDGE_LOOP ( 'NONE', ( #35709, #15630, #24145, #13795 ) ) ;
#6264=DIRECTION ( 'NONE',  ( 1.000000000000000000, 0.000000000000000000, 0.000000000000000000 ) ) ;
#6266=DIRECTION ( 'NONE',  ( 0.000000000000000000, 0.000000000000000000, 1.000000000000000000 ) ) ;
#6269=CARTESIAN_POINT ( 'NONE',  ( -30.24874870218063450, -26.64985754041175525, 6.700000000000000178 ) ) ;
#6288=AXIS2_PLACEMENT_3D ( 'NONE', #12706, #23001, #6341 ) ;
#6289=EDGE_CURVE ( 'NONE', #19079, #5789, #38414, .T. ) ;
#6291=ORIENTED_EDGE ( 'NONE', *, *, #16389, .F. ) ;
#6300=DIRECTION ( 'NONE',  ( -1.000000000000000000, 0.000000000000000000, 0.000000000000000000 ) ) ;
#6310=AXIS2_PLACEMENT_3D ( 'NONE', #23528, #7468, #36485 ) ;
#6313=DIRECTION ( 'NONE',  ( 1.000000000000000000, 0.000000000000000000, 0.000000000000000000 ) ) ;
#6316=VECTOR ( 'NONE', #24301, 1000.000000000000000 ) ;
#6317=CARTESIAN_POINT ( 'NONE',  ( -20.44874870218064444, -25.49307895267003587, 6.700000000000000178 ) ) ;
#6333=EDGE_CURVE ( 'NONE', #26136, #19316, #32070, .T. ) ;
#6341=DIRECTION ( 'NONE',  ( 1.000000000000000000, 0.000000000000000000, -0.000000000000000000 ) ) ;
#6349=ORIENTED_EDGE ( 'NONE', *, *, #5523, .T. ) ;
#6352=AXIS2_PLACEMENT_3D ( 'NONE', #34950, #10408, #38808 ) ;
#6355=PLANE ( 'NONE',  #683 ) ;
#6369=ORIENTED_EDGE ( 'NONE', *, *, #36472, .T. ) ;
#6371=ORIENTED_EDGE ( 'NONE', *, *, #38462, .F. ) ;
#6372=ORIENTED_EDGE ( 'NONE', *, *, #18388, .T. ) ;
#6377=VECTOR ( 'NONE', #4372, 1000.000000000000000 ) ;
#6382=AXIS2_PLACEMENT_3D ( 'NONE', #21703, #18801, #31577 ) ;
#6383=EDGE_CURVE ( 'NONE', #18497, #20724, #32866, .T. ) ;
#6385=PLANE ( 'NONE',  #39715 ) ;
#6386=PLANE ( 'NONE',  #18323 ) ;
#6391=ADVANCED_FACE ( 'NONE', ( #29757 ), #7931, .F. ) ;
#6401=AXIS2_PLACEMENT_3D ( 'NONE', #4474, #7541, #20289 ) ;
#6406=AXIS2_PLACEMENT_3D ( 'NONE', #37633, #33618, #36887 ) ;
#6408=VERTEX_POINT ( 'NONE', #11209 ) ;
#6409=ORIENTED_EDGE ( 'NONE', *, *, #17137, .T. ) ;
#6412=EDGE_LOOP ( 'NONE', ( #6894, #22846, #12491, #36115 ) ) ;
#6420=FACE_BOUND ( 'NONE', #19084, .T. ) ;
#6431=DIRECTION ( 'NONE',  ( 0.000000000000000000, 0.000000000000000000, 1.000000000000000000 ) ) ;
#6435=DIRECTION ( 'NONE',  ( 0.000000000000000000, 0.000000000000000000, 1.000000000000000000 ) ) ;
#6439=AXIS2_PLACEMENT_3D ( 'NONE', #5046, #29747, #36339 ) ;
#6440=EDGE_CURVE ( 'NONE', #30761, #29356, #38641, .T. ) ;
#6442=DIRECTION ( 'NONE',  ( 1.000000000000000000, 0.000000000000000000, 0.000000000000000000 ) ) ;
#6450=PLANE ( 'NONE',  #356 ) ;
#6453=VERTEX_POINT ( 'NONE', #40041 ) ;
#6455=CARTESIAN_POINT ( 'NONE',  ( -36.44874870218064444, -26.64985754041175525, 6.700000000000000178 ) ) ;
#6461=CARTESIAN_POINT ( 'NONE',  ( -20.87867591359218977, -26.64985754041175525, 6.800000000000000711 ) ) ;
#6463=CARTESIAN_POINT ( 'NONE',  ( -24.87867591359218977, -24.55319635012989110, 6.700000000000000178 ) ) ;
#6468=ORIENTED_EDGE ( 'NONE', *, *, #11786, .T. ) ;
#6469=DIRECTION ( 'NONE',  ( 0.000000000000000000, 0.000000000000000000, 1.000000000000000000 ) ) ;
#6472=VERTEX_POINT ( 'NONE', #36750 ) ;
#6474=FACE_OUTER_BOUND ( 'NONE', #25608, .T. ) ;
#6477=DIRECTION ( 'NONE',  ( -0.000000000000000000, -1.000000000000000000, -0.000000000000000000 ) ) ;
#6481=ORIENTED_EDGE ( 'NONE', *, *, #27065, .F. ) ;
#6483=ORIENTED_EDGE ( 'NONE', *, *, #24625, .F. ) ;
#6485=CIRCLE ( 'NONE', #29491, 0.1000000000000028644 ) ;
#6491=EDGE_CURVE ( 'NONE', #26477, #9234, #30592, .T. ) ;
#6500=VECTOR ( 'NONE', #37368, 1000.000000000000000 ) ;
#6515=CIRCLE ( 'NONE', #7144, 0.1000000000000028644 ) ;
#6516=DIRECTION ( 'NONE',  ( 0.000000000000000000, 1.000000000000000000, 0.000000000000000000 ) ) ;
#6524=VERTEX_POINT ( 'NONE', #3020 ) ;
#6534=LINE ( 'NONE', #27927, #32594 ) ;
#6546=LINE ( 'NONE', #31258, #26177 ) ;
#6552=DIRECTION ( 'NONE',  ( 0.000000000000000000, 0.000000000000000000, -1.000000000000000000 ) ) ;
#6556=VERTEX_POINT ( 'NONE', #34715 ) ;
#6559=VECTOR ( 'NONE', #16747, 1000.000000000000000 ) ;
#6561=LINE ( 'NONE', #390, #37033 ) ;
#6571=ADVANCED_FACE ( 'NONE', ( #37556 ), #36956, .T. ) ;
#6577=ORIENTED_EDGE ( 'NONE', *, *, #23602, .T. ) ;
#6579=ORIENTED_EDGE ( 'NONE', *, *, #10559, .T. ) ;
#6589=ADVANCED_FACE ( 'NONE', ( #9351 ), #33893, .F. ) ;
#6596=ORIENTED_EDGE ( 'NONE', *, *, #37720, .T. ) ;
#6604=VERTEX_POINT ( 'NONE', #37753 ) ;
#6610=CARTESIAN_POINT ( 'NONE',  ( -42.83131703149249603, -27.06993018339339585, 6.800000000000000711 ) ) ;
#6611=AXIS2_PLACEMENT_3D ( 'NONE', #15556, #6300, #14940 ) ;
#6612=CYLINDRICAL_SURFACE ( 'NONE', #15856, 0.1000000000000028644 ) ;
#6614=EDGE_LOOP ( 'NONE', ( #12890, #1464, #34820, #26927 ) ) ;
#6617=LINE ( 'NONE', #653, #16564 ) ;
#6623=CIRCLE ( 'NONE', #15154, 0.1000000000000028644 ) ;
#6629=FACE_BOUND ( 'NONE', #40683, .T. ) ;
#6632=ORIENTED_EDGE ( 'NONE', *, *, #19877, .T. ) ;
#6635=DIRECTION ( 'NONE',  ( -1.000000000000000000, 0.000000000000000000, 0.000000000000000000 ) ) ;
#6643=ORIENTED_EDGE ( 'NONE', *, *, #13623, .T. ) ;
#6653=ORIENTED_EDGE ( 'NONE', *, *, #13729, .F. ) ;
#6656=VECTOR ( 'NONE', #21075, 1000.000000000000000 ) ;
#6661=CARTESIAN_POINT ( 'NONE',  ( 1.551251297819356001, -25.49307895267003587, 6.700000000000000178 ) ) ;
#6668=ORIENTED_EDGE ( 'NONE', *, *, #3660, .T. ) ;
#6675=ADVANCED_FACE ( 'NONE', ( #32627 ), #35514, .F. ) ;
#6679=DIRECTION ( 'NONE',  ( 1.000000000000000000, 0.000000000000000000, 0.000000000000000000 ) ) ;
#6685=CARTESIAN_POINT ( 'NONE',  ( -24.87867591359218977, -26.64985754041175525, 6.700000000000000178 ) ) ;
#6686=ORIENTED_EDGE ( 'NONE', *, *, #14897, .F. ) ;
#6690=DIRECTION ( 'NONE',  ( -0.000000000000000000, -1.000000000000000000, -0.000000000000000000 ) ) ;
#6693=ORIENTED_EDGE ( 'NONE', *, *, #9864, .T. ) ;
#6698=CARTESIAN_POINT ( 'NONE',  ( -11.07867591359219794, -26.64985754041175525, 6.700000000000000178 ) ) ;
#6712=CARTESIAN_POINT ( 'NONE',  ( -6.248748702180631831, -25.49307895267003587, 6.700000000000000178 ) ) ;
#6713=DIRECTION ( 'NONE',  ( 1.000000000000000000, 0.000000000000000000, 0.000000000000000000 ) ) ;
#6716=DIRECTION ( 'NONE',  ( 1.000000000000000000, 0.000000000000000000, 0.000000000000000000 ) ) ;
#6727=DIRECTION ( 'NONE',  ( -0.000000000000000000, -0.000000000000000000, 1.000000000000000000 ) ) ;
#6728=DIRECTION ( 'NONE',  ( 0.000000000000000000, 0.000000000000000000, -1.000000000000000000 ) ) ;
#6729=EDGE_LOOP ( 'NONE', ( #31427, #607, #8420, #24274 ) ) ;
#6737=CARTESIAN_POINT ( 'NONE',  ( -30.34874870218063947, -26.64985754041175525, 6.700000000000000178 ) ) ;
#6744=ORIENTED_EDGE ( 'NONE', *, *, #34109, .F. ) ;
#6749=CARTESIAN_POINT ( 'NONE',  ( 1.751251297819361730, -25.49307895267003587, 6.700000000000000178 ) ) ;
#6754=ORIENTED_EDGE ( 'NONE', *, *, #3069, .T. ) ;
#6758=DIRECTION ( 'NONE',  ( -0.000000000000000000, -0.000000000000000000, 1.000000000000000000 ) ) ;
#6761=DIRECTION ( 'NONE',  ( 0.000000000000000000, 0.000000000000000000, 1.000000000000000000 ) ) ;
#6771=LINE ( 'NONE', #5951, #38864 ) ;
#6772=VERTEX_POINT ( 'NONE', #26635 ) ;
#6780=ORIENTED_EDGE ( 'NONE', *, *, #17592, .F. ) ;
#6781=VERTEX_POINT ( 'NONE', #26439 ) ;
#6783=DIRECTION ( 'NONE',  ( 1.000000000000000000, 0.000000000000000000, 0.000000000000000000 ) ) ;
#6789=ADVANCED_FACE ( 'NONE', ( #39170 ), #27035, .F. ) ;
#6790=VERTEX_POINT ( 'NONE', #8276 ) ;
#6804=EDGE_CURVE ( 'NONE', #22388, #33136, #32823, .T. ) ;
#6813=DIRECTION ( 'NONE',  ( -0.000000000000000000, -0.000000000000000000, 1.000000000000000000 ) ) ;
#6814=EDGE_CURVE ( 'NONE', #38692, #24999, #38965, .T. ) ;
#6815=ORIENTED_EDGE ( 'NONE', *, *, #3855, .F. ) ;
#6817=ORIENTED_EDGE ( 'NONE', *, *, #10084, .F. ) ;
#6819=DIRECTION ( 'NONE',  ( 0.000000000000000000, 0.000000000000000000, 1.000000000000000000 ) ) ;
#6821=ORIENTED_EDGE ( 'NONE', *, *, #19078, .F. ) ;
#6826=FACE_BOUND ( 'NONE', #6412, .T. ) ;
#6827=ORIENTED_EDGE ( 'NONE', *, *, #30174, .F. ) ;
#6839=VECTOR ( 'NONE', #4400, 1000.000000000000000 ) ;
#6840=DIRECTION ( 'NONE',  ( -0.000000000000000000, -0.000000000000000000, 1.000000000000000000 ) ) ;
#6850=EDGE_CURVE ( 'NONE', #8480, #28895, #20440, .T. ) ;
#6855=DIRECTION ( 'NONE',  ( 1.000000000000000000, 0.000000000000000000, -0.000000000000000000 ) ) ;
#6870=EDGE_LOOP ( 'NONE', ( #27558, #14894, #28426, #31324 ) ) ;
#6876=ORIENTED_EDGE ( 'NONE', *, *, #10404, .F. ) ;
#6879=AXIS2_PLACEMENT_3D ( 'NONE', #17255, #29828, #35234 ) ;
#6882=CARTESIAN_POINT ( 'NONE',  ( -10.34874870218063769, -25.49307895267003587, 6.800000000000000711 ) ) ;
#6893=FACE_OUTER_BOUND ( 'NONE', #6870, .T. ) ;
#6894=ORIENTED_EDGE ( 'NONE', *, *, #12422, .F. ) ;
#6899=AXIS2_PLACEMENT_3D ( 'NONE', #14024, #25997, #36075 ) ;
#6908=CARTESIAN_POINT ( 'NONE',  ( 1.651251297819358754, -26.64985754041175525, 6.800000000000000711 ) ) ;
#6912=CARTESIAN_POINT ( 'NONE',  ( -27.07867591359219972, -26.64985754041175525, 6.700000000000000178 ) ) ;
#6917=ORIENTED_EDGE ( 'NONE', *, *, #24253, .T. ) ;
#6927=CIRCLE ( 'NONE', #17381, 0.1000000000000028644 ) ;
#6932=DIRECTION ( 'NONE',  ( 0.000000000000000000, 0.000000000000000000, 1.000000000000000000 ) ) ;
#6933=CARTESIAN_POINT ( 'NONE',  ( -22.34874870218063947, -25.49307895267003587, 6.800000000000000711 ) ) ;
#6938=DIRECTION ( 'NONE',  ( 0.000000000000000000, -1.000000000000000000, 0.000000000000000000 ) ) ;
#6941=DIRECTION ( 'NONE',  ( -0.000000000000000000, -0.000000000000000000, 1.000000000000000000 ) ) ;
#6943=EDGE_CURVE ( 'NONE', #6524, #34445, #31974, .T. ) ;
#6946=CARTESIAN_POINT ( 'NONE',  ( -7.078675913592194391, -26.64985754041175525, 6.800000000000000711 ) ) ;
#6953=ORIENTED_EDGE ( 'NONE', *, *, #35080, .F. ) ;
#6958=LINE ( 'NONE', #594, #27331 ) ;
#6962=PLANE ( 'NONE',  #37833 ) ;
#6964=EDGE_LOOP ( 'NONE', ( #26060, #5151, #18093, #13155 ) ) ;
#6970=ORIENTED_EDGE ( 'NONE', *, *, #10830, .T. ) ;
#6971=DIRECTION ( 'NONE',  ( 0.000000000000000000, 0.000000000000000000, -1.000000000000000000 ) ) ;
#6972=EDGE_LOOP ( 'NONE', ( #16882, #33945, #29542, #10257 ) ) ;
#6978=ORIENTED_EDGE ( 'NONE', *, *, #24100, .F. ) ;
#6980=AXIS2_PLACEMENT_3D ( 'NONE', #40127, #11907, #18297 ) ;
#6984=LINE ( 'NONE', #23043, #28387 ) ;
#6989=AXIS2_PLACEMENT_3D ( 'NONE', #6232, #34665, #6442 ) ;
#6998=ORIENTED_EDGE ( 'NONE', *, *, #32982, .F. ) ;
#6999=CARTESIAN_POINT ( 'NONE',  ( -6.878675913592188884, -26.64985754041175525, 6.700000000000000178 ) ) ;
#7009=ORIENTED_EDGE ( 'NONE', *, *, #17233, .T. ) ;
#7013=CIRCLE ( 'NONE', #10295, 0.1000000000000028644 ) ;
#7016=AXIS2_PLACEMENT_3D ( 'NONE', #1389, #13311, #13732 ) ;
#7017=VERTEX_POINT ( 'NONE', #29619 ) ;
#7020=FACE_BOUND ( 'NONE', #8160, .T. ) ;
#7022=ORIENTED_EDGE ( 'NONE', *, *, #28607, .T. ) ;
#7026=ORIENTED_EDGE ( 'NONE', *, *, #28164, .T. ) ;
#7027=VERTEX_POINT ( 'NONE', #37209 ) ;
#7029=DIRECTION ( 'NONE',  ( 0.000000000000000000, 0.000000000000000000, 1.000000000000000000 ) ) ;
#7030=LINE ( 'NONE', #13404, #19640 ) ;
#7036=DIRECTION ( 'NONE',  ( -0.000000000000000000, -0.000000000000000000, 1.000000000000000000 ) ) ;
#7042=VECTOR ( 'NONE', #36961, 1000.000000000000000 ) ;
#7044=VECTOR ( 'NONE', #22113, 1000.000000000000000 ) ;
#7046=CARTESIAN_POINT ( 'NONE',  ( 5.551251297819359110, -26.64985754041175525, 6.700000000000000178 ) ) ;
#7057=ORIENTED_EDGE ( 'NONE', *, *, #30, .F. ) ;
#7062=ORIENTED_EDGE ( 'NONE', *, *, #31451, .F. ) ;
#7069=DIRECTION ( 'NONE',  ( 0.000000000000000000, 0.000000000000000000, 1.000000000000000000 ) ) ;
#7073=EDGE_CURVE ( 'NONE', #24284, #826, #6485, .T. ) ;
#7076=CARTESIAN_POINT ( 'NONE',  ( -15.07867591359219439, -26.64985754041175525, 6.700000000000000178 ) ) ;
#7089=ORIENTED_EDGE ( 'NONE', *, *, #34804, .T. ) ;
#7106=VECTOR ( 'NONE', #19544, 1000.000000000000000 ) ;
#7108=CARTESIAN_POINT ( 'NONE',  ( -21.07867591359219617, -26.64985754041175525, 6.700000000000000178 ) ) ;
#7128=EDGE_CURVE ( 'NONE', #20627, #30874, #39475, .T. ) ;
#7140=CARTESIAN_POINT ( 'NONE',  ( 11.65737507970504439, -23.60493063168009442, 6.800000000000000711 ) ) ;
#7144=AXIS2_PLACEMENT_3D ( 'NONE', #15089, #33650, #20863 ) ;
#7146=CARTESIAN_POINT ( 'NONE',  ( -26.24874870218063450, -26.64985754041175525, 6.800000000000000711 ) ) ;
#7153=EDGE_CURVE ( 'NONE', #12332, #4935, #19095, .T. ) ;
#7164=ORIENTED_EDGE ( 'NONE', *, *, #30019, .T. ) ;
#7170=VERTEX_POINT ( 'NONE', #28309 ) ;
#7177=DIRECTION ( 'NONE',  ( -0.000000000000000000, -1.000000000000000000, -0.000000000000000000 ) ) ;
#7179=ORIENTED_EDGE ( 'NONE', *, *, #21238, .F. ) ;
#7182=DIRECTION ( 'NONE',  ( -0.000000000000000000, -0.000000000000000000, 1.000000000000000000 ) ) ;
#7187=CARTESIAN_POINT ( 'NONE',  ( -6.978675913592191193, -24.55319635012989110, 6.700000000000000178 ) ) ;
#7193=FACE_OUTER_BOUND ( 'NONE', #17869, .T. ) ;
#7207=DIRECTION ( 'NONE',  ( 1.000000000000000000, 0.000000000000000000, 0.000000000000000000 ) ) ;
#7209=ORIENTED_EDGE ( 'NONE', *, *, #18438, .T. ) ;
#7215=VERTEX_POINT ( 'NONE', #27892 ) ;
#7220=CARTESIAN_POINT ( 'NONE',  ( -18.97867591359219475, -26.64985754041175525, 6.800000000000000711 ) ) ;
#7225=ORIENTED_EDGE ( 'NONE', *, *, #31175, .T. ) ;
#7227=VECTOR ( 'NONE', #19059, 1000.000000000000000 ) ;
#7245=DIRECTION ( 'NONE',  ( -1.000000000000000000, 0.000000000000000000, 0.000000000000000000 ) ) ;
#7250=FACE_OUTER_BOUND ( 'NONE', #24531, .T. ) ;
#7255=AXIS2_PLACEMENT_3D ( 'NONE', #23360, #4632, #942 ) ;
#7261=ORIENTED_EDGE ( 'NONE', *, *, #12068, .T. ) ;
#7262=DIRECTION ( 'NONE',  ( -0.000000000000000000, -1.000000000000000000, -0.000000000000000000 ) ) ;
#7264=EDGE_CURVE ( 'NONE', #2177, #7027, #23350, .T. ) ;
#7283=VECTOR ( 'NONE', #13224, 1000.000000000000000 ) ;
#7292=FACE_OUTER_BOUND ( 'NONE', #33331, .T. ) ;
#7294=CARTESIAN_POINT ( 'NONE',  ( -2.448748702180640446, -26.64985754041175525, 6.700000000000000178 ) ) ;
#7303=CIRCLE ( 'NONE', #96, 0.1000000000000028644 ) ;
#7304=EDGE_CURVE ( 'NONE', #10217, #18938, #35523, .T. ) ;
#7307=LINE ( 'NONE', #28735, #26249 ) ;
#7313=ADVANCED_FACE ( 'NONE', ( #10772 ), #13072, .F. ) ;
#7319=ORIENTED_EDGE ( 'NONE', *, *, #13383, .T. ) ;
#7327=ORIENTED_EDGE ( 'NONE', *, *, #32705, .F. ) ;
#7328=EDGE_CURVE ( 'NONE', #20273, #18938, #35123, .T. ) ;
#7329=DIRECTION ( 'NONE',  ( 0.000000000000000000, 1.000000000000000000, 0.000000000000000000 ) ) ;
#7340=CARTESIAN_POINT ( 'NONE',  ( -30.44874870218064089, -25.49307895267003587, 6.800000000000000711 ) ) ;
#7345=DIRECTION ( 'NONE',  ( 1.000000000000000000, 0.000000000000000000, 0.000000000000000000 ) ) ;
#7349=EDGE_CURVE ( 'NONE', #34241, #24116, #9979, .T. ) ;
#7354=ORIENTED_EDGE ( 'NONE', *, *, #17829, .F. ) ;
#7358=CARTESIAN_POINT ( 'NONE',  ( -40.87867591359218977, -24.55319635012989110, 6.700000000000000178 ) ) ;
#7378=LINE ( 'NONE', #13558, #17838 ) ;
#7405=CARTESIAN_POINT ( 'NONE',  ( -5.078675913592192614, -26.64985754041175525, 6.800000000000000711 ) ) ;
#7412=LINE ( 'NONE', #4733, #37241 ) ;
#7416=ORIENTED_EDGE ( 'NONE', *, *, #27185, .T. ) ;
#7427=DIRECTION ( 'NONE',  ( 0.000000000000000000, 1.000000000000000000, 0.000000000000000000 ) ) ;
#7441=ADVANCED_FACE ( 'NONE', ( #33027 ), #1741, .F. ) ;
#7444=ORIENTED_EDGE ( 'NONE', *, *, #15097, .F. ) ;
#7445=CARTESIAN_POINT ( 'NONE',  ( -24.97867591359219475, -24.55319635012989110, 6.800000000000000711 ) ) ;
#7447=LINE ( 'NONE', #687, #9836 ) ;
#7450=DIRECTION ( 'NONE',  ( -0.000000000000000000, -1.000000000000000000, -0.000000000000000000 ) ) ;
#7452=CARTESIAN_POINT ( 'NONE',  ( -34.97867591359219830, -24.55319635012989110, 6.800000000000000711 ) ) ;
#7453=DIRECTION ( 'NONE',  ( 0.000000000000000000, 0.000000000000000000, 1.000000000000000000 ) ) ;
#7454=DIRECTION ( 'NONE',  ( 0.000000000000000000, 0.000000000000000000, 1.000000000000000000 ) ) ;
#7468=DIRECTION ( 'NONE',  ( -0.000000000000000000, -0.000000000000000000, 1.000000000000000000 ) ) ;
#7472=DIRECTION ( 'NONE',  ( 1.000000000000000000, 0.000000000000000000, 0.000000000000000000 ) ) ;
#7474=VECTOR ( 'NONE', #27507, 1000.000000000000000 ) ;
#7476=DIRECTION ( 'NONE',  ( -0.000000000000000000, -0.000000000000000000, -1.000000000000000000 ) ) ;
#7485=AXIS2_PLACEMENT_3D ( 'NONE', #12835, #40223, #22123 ) ;
#7491=ORIENTED_EDGE ( 'NONE', *, *, #36349, .F. ) ;
#7500=DIRECTION ( 'NONE',  ( 0.000000000000000000, 0.000000000000000000, 1.000000000000000000 ) ) ;
#7501=CARTESIAN_POINT ( 'NONE',  ( 5.751251297819365504, -26.64985754041175525, 6.700000000000000178 ) ) ;
#7506=ORIENTED_EDGE ( 'NONE', *, *, #29570, .F. ) ;
#7512=AXIS2_PLACEMENT_3D ( 'NONE', #11605, #20890, #20470 ) ;
#7513=DIRECTION ( 'NONE',  ( 1.000000000000000000, -0.000000000000000000, 0.000000000000000000 ) ) ;
#7515=ADVANCED_FACE ( 'NONE', ( #36515 ), #23743, .F. ) ;
#7518=CARTESIAN_POINT ( 'NONE',  ( -54.01549048184568846, -38.28842912540938670, 6.000000000000000000 ) ) ;
#7521=ORIENTED_EDGE ( 'NONE', *, *, #21855, .T. ) ;
#7528=CIRCLE ( 'NONE', #10783, 0.1000000000000028644 ) ;
#7531=PLANE ( 'NONE',  #5117 ) ;
#7541=DIRECTION ( 'NONE',  ( -0.000000000000000000, -0.000000000000000000, 1.000000000000000000 ) ) ;
#7546=CARTESIAN_POINT ( 'NONE',  ( -40.34874870218063592, -25.49307895267003587, 6.700000000000000178 ) ) ;
#7547=FACE_OUTER_BOUND ( 'NONE', #14020, .T. ) ;
#7551=DIRECTION ( 'NONE',  ( -0.000000000000000000, -0.000000000000000000, 1.000000000000000000 ) ) ;
#7557=LINE ( 'NONE', #30619, #4957 ) ;
#7566=CIRCLE ( 'NONE', #37162, 0.1000000000000028644 ) ;
#7569=VERTEX_POINT ( 'NONE', #15909 ) ;
#7574=EDGE_CURVE ( 'NONE', #2073, #1149, #26272, .T. ) ;
#7577=VERTEX_POINT ( 'NONE', #34065 ) ;
#7583=DIRECTION ( 'NONE',  ( 1.000000000000000000, 0.000000000000000000, 0.000000000000000000 ) ) ;
#7589=AXIS2_PLACEMENT_3D ( 'NONE', #20820, #17511, #30927 ) ;
#7606=DIRECTION ( 'NONE',  ( -0.000000000000000000, -1.000000000000000000, -0.000000000000000000 ) ) ;
#7607=CARTESIAN_POINT ( 'NONE',  ( -26.44874870218064089, -26.64985754041175525, 6.700000000000000178 ) ) ;
#7617=AXIS2_PLACEMENT_3D ( 'NONE', #39230, #7746, #17600 ) ;
#7619=AXIS2_PLACEMENT_3D ( 'NONE', #21458, #15060, #18547 ) ;
#7620=ADVANCED_FACE ( 'NONE', ( #11985 ), #25388, .F. ) ;
#7627=VECTOR ( 'NONE', #19445, 1000.000000000000000 ) ;
#7631=ORIENTED_EDGE ( 'NONE', *, *, #3895, .F. ) ;
#7633=CARTESIAN_POINT ( 'NONE',  ( -28.87867591359218977, -26.64985754041175525, 6.700000000000000178 ) ) ;
#7638=CARTESIAN_POINT ( 'NONE',  ( -17.07867591359219617, -26.64985754041175525, 6.700000000000000178 ) ) ;
#7650=ORIENTED_EDGE ( 'NONE', *, *, #38567, .T. ) ;
#7655=DIRECTION ( 'NONE',  ( -1.000000000000000000, 0.000000000000000000, 0.000000000000000000 ) ) ;
#7658=EDGE_CURVE ( 'NONE', #13011, #26146, #9520, .T. ) ;
#7659=CARTESIAN_POINT ( 'NONE',  ( -14.24874870218063450, -25.49307895267003587, 6.700000000000000178 ) ) ;
#7667=LINE ( 'NONE', #4591, #39735 ) ;
#7673=EDGE_LOOP ( 'NONE', ( #2551, #26103, #29495, #25941 ) ) ;
#7675=EDGE_CURVE ( 'NONE', #22775, #26905, #31568, .T. ) ;
#7688=AXIS2_PLACEMENT_3D ( 'NONE', #8541, #36553, #5261 ) ;
#7690=DIRECTION ( 'NONE',  ( -0.000000000000000000, -1.000000000000000000, -0.000000000000000000 ) ) ;
#7720=DIRECTION ( 'NONE',  ( 0.000000000000000000, 1.000000000000000000, 0.000000000000000000 ) ) ;
#7721=CYLINDRICAL_SURFACE ( 'NONE', #33152, 0.1000000000000028644 ) ;
#7726=ORIENTED_EDGE ( 'NONE', *, *, #31680, .F. ) ;
#7734=DIRECTION ( 'NONE',  ( -0.000000000000000000, -0.000000000000000000, 1.000000000000000000 ) ) ;
#7739=DIRECTION ( 'NONE',  ( 1.000000000000000000, 0.000000000000000000, 0.000000000000000000 ) ) ;
#7742=CARTESIAN_POINT ( 'NONE',  ( -24.44874870218064089, -25.49307895267003587, 6.700000000000000178 ) ) ;
#7746=DIRECTION ( 'NONE',  ( -1.000000000000000000, 0.000000000000000000, 0.000000000000000000 ) ) ;
#7752=PLANE ( 'NONE',  #22838 ) ;
#7753=DIRECTION ( 'NONE',  ( 1.000000000000000000, 0.000000000000000000, 0.000000000000000000 ) ) ;
#7764=ORIENTED_EDGE ( 'NONE', *, *, #34848, .T. ) ;
#7770=EDGE_CURVE ( 'NONE', #22883, #10139, #16311, .T. ) ;
#7773=DIRECTION ( 'NONE',  ( -0.000000000000000000, -0.000000000000000000, -1.000000000000000000 ) ) ;
#7780=CARTESIAN_POINT ( 'NONE',  ( -39.07867591359219261, -26.64985754041175525, 6.700000000000000178 ) ) ;
#7783=CARTESIAN_POINT ( 'NONE',  ( -34.44874870218064444, -26.64985754041175525, 6.700000000000000178 ) ) ;
#7789=DIRECTION ( 'NONE',  ( 0.000000000000000000, 0.000000000000000000, 1.000000000000000000 ) ) ;
#7793=ORIENTED_EDGE ( 'NONE', *, *, #37643, .T. ) ;
#7794=EDGE_CURVE ( 'NONE', #18315, #24999, #7447, .T. ) ;
#7802=ADVANCED_FACE ( 'NONE', ( #16906 ), #38325, .F. ) ;
#7806=ADVANCED_FACE ( 'NONE', ( #19614 ), #16505, .T. ) ;
#7811=ORIENTED_EDGE ( 'NONE', *, *, #24794, .T. ) ;
#7815=CARTESIAN_POINT ( 'NONE',  ( -32.44874870218063734, -26.64985754041175525, 6.800000000000000711 ) ) ;
#7817=DIRECTION ( 'NONE',  ( 1.000000000000000000, 0.000000000000000000, 0.000000000000000000 ) ) ;
#7828=CARTESIAN_POINT ( 'NONE',  ( -24.44874870218064089, -26.64985754041175525, 6.800000000000000711 ) ) ;
#7841=LINE ( 'NONE', #20797, #608 ) ;
#7846=PLANE ( 'NONE',  #34616 ) ;
#7849=DIRECTION ( 'NONE',  ( -0.000000000000000000, -0.000000000000000000, 1.000000000000000000 ) ) ;
#7852=FACE_OUTER_BOUND ( 'NONE', #38071, .T. ) ;
#7856=ADVANCED_FACE ( 'NONE', ( #20599 ), #17104, .F. ) ;
#7857=AXIS2_PLACEMENT_3D ( 'NONE', #33183, #23305, #23696 ) ;
#7862=CYLINDRICAL_SURFACE ( 'NONE', #33041, 0.1000000000000028644 ) ;
#7863=ADVANCED_FACE ( 'NONE', ( #20402 ), #30496, .F. ) ;
#7867=CARTESIAN_POINT ( 'NONE',  ( -2.448748702180640446, -25.49307895267003587, 6.700000000000000178 ) ) ;
#7868=CIRCLE ( 'NONE', #34858, 0.1000000000000028644 ) ;
#7869=DIRECTION ( 'NONE',  ( -0.000000000000000000, -0.000000000000000000, 1.000000000000000000 ) ) ;
#7878=FACE_OUTER_BOUND ( 'NONE', #25909, .T. ) ;
#7879=VERTEX_POINT ( 'NONE', #33402 ) ;
#7884=CARTESIAN_POINT ( 'NONE',  ( -26.34874870218063947, -26.64985754041175525, 6.800000000000000711 ) ) ;
#7892=VERTEX_POINT ( 'NONE', #23888 ) ;
#7893=CARTESIAN_POINT ( 'NONE',  ( -28.44874870218064444, -26.64985754041175525, 6.700000000000000178 ) ) ;
#7896=DIRECTION ( 'NONE',  ( 0.000000000000000000, 0.000000000000000000, 1.000000000000000000 ) ) ;
#7898=EDGE_CURVE ( 'NONE', #3715, #8480, #21655, .T. ) ;
#7899=VECTOR ( 'NONE', #37749, 1000.000000000000000 ) ;
#7900=VERTEX_POINT ( 'NONE', #20805 ) ;
#7918=LINE ( 'NONE', #21302, #14937 ) ;
#7920=CARTESIAN_POINT ( 'NONE',  ( 1.751251297819361730, -26.64985754041175525, 6.700000000000000178 ) ) ;
#7921=DIRECTION ( 'NONE',  ( -0.000000000000000000, -0.000000000000000000, -1.000000000000000000 ) ) ;
#7923=VECTOR ( 'NONE', #11994, 1000.000000000000000 ) ;
#7929=CARTESIAN_POINT ( 'NONE',  ( -26.44874870218064089, -26.64985754041175525, 6.700000000000000178 ) ) ;
#7931=CYLINDRICAL_SURFACE ( 'NONE', #20241, 0.1000000000000028644 ) ;
#7946=EDGE_CURVE ( 'NONE', #6604, #21608, #21639, .T. ) ;
#7948=LINE ( 'NONE', #30183, #2924 ) ;
#7961=ORIENTED_EDGE ( 'NONE', *, *, #11418, .F. ) ;
#7973=CARTESIAN_POINT ( 'NONE',  ( -37.07867591359219261, -26.64985754041175525, 6.800000000000000711 ) ) ;
#7974=DIRECTION ( 'NONE',  ( -0.000000000000000000, -0.000000000000000000, 1.000000000000000000 ) ) ;
#7979=ORIENTED_EDGE ( 'NONE', *, *, #3163, .T. ) ;
#7982=CARTESIAN_POINT ( 'NONE',  ( -38.87867591359218977, -26.64985754041175525, 6.700000000000000178 ) ) ;
#7986=VERTEX_POINT ( 'NONE', #24512 ) ;
#7988=EDGE_LOOP ( 'NONE', ( #39774, #40644, #14063, #11904 ) ) ;
#7993=CARTESIAN_POINT ( 'NONE',  ( -39.07867591359219261, -24.55319635012989110, 6.700000000000000178 ) ) ;
#8001=ORIENTED_EDGE ( 'NONE', *, *, #480, .F. ) ;
#8002=ORIENTED_EDGE ( 'NONE', *, *, #25950, .T. ) ;
#8008=ORIENTED_EDGE ( 'NONE', *, *, #22195, .F. ) ;
#8011=ORIENTED_EDGE ( 'NONE', *, *, #20725, .T. ) ;
#8013=EDGE_LOOP ( 'NONE', ( #39260, #22502, #40043, #10733 ) ) ;
#8026=LINE ( 'NONE', #39119, #31334 ) ;
#8031=PLANE ( 'NONE',  #16870 ) ;
#8035=DIRECTION ( 'NONE',  ( -0.000000000000000000, -0.000000000000000000, 1.000000000000000000 ) ) ;
#8041=EDGE_CURVE ( 'NONE', #31820, #32857, #9866, .T. ) ;
#8043=LINE ( 'NONE', #14425, #1635 ) ;
#8051=EDGE_CURVE ( 'NONE', #25629, #408, #21227, .T. ) ;
#8059=AXIS2_PLACEMENT_3D ( 'NONE', #37949, #28283, #6679 ) ;
#8065=DIRECTION ( 'NONE',  ( -0.000000000000000000, -0.000000000000000000, 1.000000000000000000 ) ) ;
#8069=CARTESIAN_POINT ( 'NONE',  ( -42.34874870218063592, -25.49307895267003587, 6.700000000000000178 ) ) ;
#8086=CARTESIAN_POINT ( 'NONE',  ( -18.97867591359219475, -24.55319635012989110, 6.700000000000000178 ) ) ;
#8094=CIRCLE ( 'NONE', #38982, 0.1000000000000028644 ) ;
#8097=CARTESIAN_POINT ( 'NONE',  ( -18.24874870218063450, -26.64985754041175525, 6.700000000000000178 ) ) ;
#8099=AXIS2_PLACEMENT_3D ( 'NONE', #37717, #11782, #21084 ) ;
#8104=CARTESIAN_POINT ( 'NONE',  ( -54.01549048184568846, -30.38627270959228710, -4.152976064860135708 ) ) ;
#8106=FACE_OUTER_BOUND ( 'NONE', #2892, .T. ) ;
#8107=DIRECTION ( 'NONE',  ( 1.000000000000000000, 0.000000000000000000, 0.000000000000000000 ) ) ;
#8115=EDGE_CURVE ( 'NONE', #7900, #34397, #2660, .T. ) ;
#8124=AXIS2_PLACEMENT_3D ( 'NONE', #30782, #11593, #15108 ) ;
#8125=VECTOR ( 'NONE', #22758, 1000.000000000000000 ) ;
#8134=VECTOR ( 'NONE', #4592, 1000.000000000000000 ) ;
#8146=PLANE ( 'NONE',  #32315 ) ;
#8147=DIRECTION ( 'NONE',  ( 0.000000000000000000, 0.000000000000000000, 1.000000000000000000 ) ) ;
#8152=AXIS2_PLACEMENT_3D ( 'NONE', #13438, #4194, #38544 ) ;
#8156=LINE ( 'NONE', #39875, #39806 ) ;
#8160=EDGE_LOOP ( 'NONE', ( #20889, #22797, #17847, #14792 ) ) ;
#8167=DIRECTION ( 'NONE',  ( -0.000000000000000000, -0.000000000000000000, 1.000000000000000000 ) ) ;
#8168=DIRECTION ( 'NONE',  ( 0.000000000000000000, 0.000000000000000000, 1.000000000000000000 ) ) ;
#8171=ORIENTED_EDGE ( 'NONE', *, *, #23351, .T. ) ;
#8174=DIRECTION ( 'NONE',  ( 1.000000000000000000, 0.000000000000000000, 0.000000000000000000 ) ) ;
#8179=ORIENTED_EDGE ( 'NONE', *, *, #28275, .T. ) ;
#8185=DIRECTION ( 'NONE',  ( -0.000000000000000000, -0.000000000000000000, 1.000000000000000000 ) ) ;
#8187=DIRECTION ( 'NONE',  ( 0.000000000000000000, 0.000000000000000000, 1.000000000000000000 ) ) ;
#8188=ORIENTED_EDGE ( 'NONE', *, *, #2821, .T. ) ;
#8197=LINE ( 'NONE', #20767, #38559 ) ;
#8209=DIRECTION ( 'NONE',  ( -1.000000000000000000, 0.000000000000000000, 0.000000000000000000 ) ) ;
#8210=EDGE_LOOP ( 'NONE', ( #4949, #33053, #15625, #39246 ) ) ;
#8213=VECTOR ( 'NONE', #35432, 1000.000000000000000 ) ;
#8217=ORIENTED_EDGE ( 'NONE', *, *, #26139, .T. ) ;
#8224=VECTOR ( 'NONE', #25451, 1000.000000000000000 ) ;
#8226=DIRECTION ( 'NONE',  ( -0.000000000000000000, -1.000000000000000000, -0.000000000000000000 ) ) ;
#8235=CARTESIAN_POINT ( 'NONE',  ( -34.34874870218063592, -25.49307895267003587, 6.700000000000000178 ) ) ;
#8237=DIRECTION ( 'NONE',  ( 0.000000000000000000, 0.000000000000000000, 1.000000000000000000 ) ) ;
#8240=DIRECTION ( 'NONE',  ( -0.000000000000000000, -0.000000000000000000, 1.000000000000000000 ) ) ;
#8242=CARTESIAN_POINT ( 'NONE',  ( -38.97867591359219119, -24.55319635012989110, 6.800000000000000711 ) ) ;
#8243=AXIS2_PLACEMENT_3D ( 'NONE', #31883, #26108, #3695 ) ;
#8251=DIRECTION ( 'NONE',  ( -0.000000000000000000, -0.000000000000000000, 1.000000000000000000 ) ) ;
#8252=LINE ( 'NONE', #10741, #8134 ) ;
#8253=CARTESIAN_POINT ( 'NONE',  ( -14.87867591359218977, -26.64985754041175525, 6.800000000000000711 ) ) ;
#8258=CARTESIAN_POINT ( 'NONE',  ( -17.07867591359219617, -24.55319635012989110, 6.700000000000000178 ) ) ;
#8273=VERTEX_POINT ( 'NONE', #6123 ) ;
#8275=LINE ( 'NONE', #33842, #32967 ) ;
#8276=CARTESIAN_POINT ( 'NONE',  ( -4.248748702180636272, -25.49307895267003587, 6.700000000000000178 ) ) ;
#8277=ORIENTED_EDGE ( 'NONE', *, *, #3672, .T. ) ;
#8279=LINE ( 'NONE', #20854, #12239 ) ;
#8280=DIRECTION ( 'NONE',  ( 0.000000000000000000, 0.000000000000000000, 1.000000000000000000 ) ) ;
#8281=VERTEX_POINT ( 'NONE', #37801 ) ;
#8284=CIRCLE ( 'NONE', #14231, 0.1000000000000028644 ) ;
#8285=ADVANCED_FACE ( 'NONE', ( #24858 ), #31246, .T. ) ;
#8287=LINE ( 'NONE', #20861, #10568 ) ;
#8292=DIRECTION ( 'NONE',  ( 0.000000000000000000, 1.000000000000000000, 0.000000000000000000 ) ) ;
#8294=DIRECTION ( 'NONE',  ( 0.000000000000000000, 0.000000000000000000, -1.000000000000000000 ) ) ;
#8296=DIRECTION ( 'NONE',  ( 1.000000000000000000, 0.000000000000000000, 0.000000000000000000 ) ) ;
#8299=ORIENTED_EDGE ( 'NONE', *, *, #3346, .T. ) ;
#8302=EDGE_CURVE ( 'NONE', #24328, #25004, #24309, .T. ) ;
#8305=VERTEX_POINT ( 'NONE', #18875 ) ;
#8312=AXIS2_PLACEMENT_3D ( 'NONE', #34478, #6253, #37126 ) ;
#8315=CARTESIAN_POINT ( 'NONE',  ( -14.34874870218063769, -26.64985754041175525, 6.800000000000000711 ) ) ;
#8316=CARTESIAN_POINT ( 'NONE',  ( -2.248748702180634940, -26.64985754041175525, 6.700000000000000178 ) ) ;
#8323=DIRECTION ( 'NONE',  ( 0.000000000000000000, 1.000000000000000000, 0.000000000000000000 ) ) ;
#8327=ORIENTED_EDGE ( 'NONE', *, *, #32242, .F. ) ;
#8332=VECTOR ( 'NONE', #26931, 1000.000000000000000 ) ;
#8338=CARTESIAN_POINT ( 'NONE',  ( -45.33131703149249603, -29.56993018339339940, 6.000000000000000000 ) ) ;
#8341=VECTOR ( 'NONE', #24629, 1000.000000000000000 ) ;
#8349=EDGE_CURVE ( 'NONE', #13245, #21734, #9812, .T. ) ;
#8353=DIRECTION ( 'NONE',  ( 1.000000000000000000, 0.000000000000000000, 0.000000000000000000 ) ) ;
#8360=DIRECTION ( 'NONE',  ( 1.000000000000000000, -0.000000000000000000, 0.000000000000000000 ) ) ;
#8370=ORIENTED_EDGE ( 'NONE', *, *, #18209, .T. ) ;
#8375=CARTESIAN_POINT ( 'NONE',  ( -45.33131703149249603, -29.56993018339339940, 6.800000000000000711 ) ) ;
#8376=CARTESIAN_POINT ( 'NONE',  ( 2.921324086407800280, -24.55319635012989110, 6.800000000000000711 ) ) ;
#8380=LINE ( 'NONE', #21580, #22219 ) ;
#8384=DIRECTION ( 'NONE',  ( -0.000000000000000000, -0.000000000000000000, 1.000000000000000000 ) ) ;
#8401=ORIENTED_EDGE ( 'NONE', *, *, #38992, .T. ) ;
#8406=ORIENTED_EDGE ( 'NONE', *, *, #12472, .T. ) ;
#8407=ORIENTED_EDGE ( 'NONE', *, *, #15587, .T. ) ;
#8413=FACE_OUTER_BOUND ( 'NONE', #6964, .T. ) ;
#8415=ORIENTED_EDGE ( 'NONE', *, *, #11932, .F. ) ;
#8420=ORIENTED_EDGE ( 'NONE', *, *, #16134, .T. ) ;
#8427=DIRECTION ( 'NONE',  ( -0.000000000000000000, -0.000000000000000000, 1.000000000000000000 ) ) ;
#8431=CARTESIAN_POINT ( 'NONE',  ( -22.97867591359219119, -26.64985754041175525, 6.700000000000000178 ) ) ;
#8443=VECTOR ( 'NONE', #15501, 1000.000000000000000 ) ;
#8450=DIRECTION ( 'NONE',  ( -0.000000000000000000, -0.000000000000000000, 1.000000000000000000 ) ) ;
#8452=EDGE_LOOP ( 'NONE', ( #20078, #36416, #14998, #36877 ) ) ;
#8458=VERTEX_POINT ( 'NONE', #16193 ) ;
#8464=ORIENTED_EDGE ( 'NONE', *, *, #27974, .F. ) ;
#8466=FACE_OUTER_BOUND ( 'NONE', #34624, .T. ) ;
#8473=ORIENTED_EDGE ( 'NONE', *, *, #16389, .T. ) ;
#8480=VERTEX_POINT ( 'NONE', #38207 ) ;
#8490=CARTESIAN_POINT ( 'NONE',  ( -40.44874870218063734, -25.49307895267003587, 6.800000000000000711 ) ) ;
#8495=DIRECTION ( 'NONE',  ( -0.000000000000000000, -0.000000000000000000, 1.000000000000000000 ) ) ;
#8501=CARTESIAN_POINT ( 'NONE',  ( 1.751251297819361730, -26.64985754041175525, 6.700000000000000178 ) ) ;
#8504=CARTESIAN_POINT ( 'NONE',  ( 3.551251297819357777, -26.64985754041175525, 6.700000000000000178 ) ) ;
#8506=AXIS2_PLACEMENT_3D ( 'NONE', #23861, #8209, #39721 ) ;
#8514=ORIENTED_EDGE ( 'NONE', *, *, #25204, .F. ) ;
#8516=DIRECTION ( 'NONE',  ( -0.000000000000000000, -0.000000000000000000, 1.000000000000000000 ) ) ;
#8518=FACE_OUTER_BOUND ( 'NONE', #34853, .T. ) ;
#8532=ORIENTED_EDGE ( 'NONE', *, *, #27516, .F. ) ;
#8533=PLANE ( 'NONE',  #33059 ) ;
#8534=AXIS2_PLACEMENT_3D ( 'NONE', #37772, #13274, #35336 ) ;
#8541=CARTESIAN_POINT ( 'NONE',  ( -16.97867591359219475, -24.55319635012989110, 6.800000000000000711 ) ) ;
#8543=DIRECTION ( 'NONE',  ( 1.000000000000000000, 0.000000000000000000, 0.000000000000000000 ) ) ;
#8552=DIRECTION ( 'NONE',  ( -0.000000000000000000, -0.000000000000000000, 1.000000000000000000 ) ) ;
#8554=ADVANCED_FACE ( 'NONE', ( #30947 ), #17184, .F. ) ;
#8559=CIRCLE ( 'NONE', #23705, 0.1000000000000028644 ) ;
#8561=DIRECTION ( 'NONE',  ( 1.000000000000000000, 0.000000000000000000, 0.000000000000000000 ) ) ;
#8562=FACE_OUTER_BOUND ( 'NONE', #30996, .T. ) ;
#8563=DIRECTION ( 'NONE',  ( 1.000000000000000000, 0.000000000000000000, -0.000000000000000000 ) ) ;
#8581=DIRECTION ( 'NONE',  ( -0.000000000000000000, -0.000000000000000000, 1.000000000000000000 ) ) ;
#8582=FACE_OUTER_BOUND ( 'NONE', #4411, .T. ) ;
#8583=FACE_OUTER_BOUND ( 'NONE', #9438, .T. ) ;
#8591=CIRCLE ( 'NONE', #21785, 0.1000000000000028644 ) ;
#8596=LINE ( 'NONE', #27948, #18067 ) ;
#8601=DIRECTION ( 'NONE',  ( -0.000000000000000000, 1.000000000000000000, -0.000000000000000000 ) ) ;
#8614=ORIENTED_EDGE ( 'NONE', *, *, #3330, .F. ) ;
#8628=EDGE_CURVE ( 'NONE', #13813, #36848, #17067, .T. ) ;
#8632=DIRECTION ( 'NONE',  ( 1.000000000000000000, 0.000000000000000000, 0.000000000000000000 ) ) ;
#8636=ORIENTED_EDGE ( 'NONE', *, *, #28164, .F. ) ;
#8641=PLANE ( 'NONE',  #25633 ) ;
#8642=ORIENTED_EDGE ( 'NONE', *, *, #24250, .F. ) ;
#8654=DIRECTION ( 'NONE',  ( 0.000000000000000000, 0.000000000000000000, 1.000000000000000000 ) ) ;
#8657=EDGE_LOOP ( 'NONE', ( #40116, #7631, #35354, #22525 ) ) ;
#8668=EDGE_LOOP ( 'NONE', ( #8936, #10975, #28700, #6191 ) ) ;
#8675=CARTESIAN_POINT ( 'NONE',  ( 1.551251297819356001, -26.64985754041175525, 6.700000000000000178 ) ) ;
#8682=VECTOR ( 'NONE', #22919, 1000.000000000000000 ) ;
#8688=AXIS2_PLACEMENT_3D ( 'NONE', #12217, #9532, #22116 ) ;
#8690=DIRECTION ( 'NONE',  ( 0.000000000000000000, 1.000000000000000000, 0.000000000000000000 ) ) ;
#8694=CYLINDRICAL_SURFACE ( 'NONE', #8805, 0.1000000000000028644 ) ;
#8700=DIRECTION ( 'NONE',  ( 1.000000000000000000, 0.000000000000000000, 0.000000000000000000 ) ) ;
#8714=CARTESIAN_POINT ( 'NONE',  ( -4.978675913592189417, -26.64985754041175525, 6.700000000000000178 ) ) ;
#8716=CIRCLE ( 'NONE', #2191, 0.1000000000000028644 ) ;
#8717=VERTEX_POINT ( 'NONE', #19952 ) ;
#8734=CARTESIAN_POINT ( 'NONE',  ( -12.24874870218063627, -26.64985754041175525, 6.800000000000000711 ) ) ;
#8738=VERTEX_POINT ( 'NONE', #38282 ) ;
#8752=DIRECTION ( 'NONE',  ( 0.000000000000000000, 0.000000000000000000, 1.000000000000000000 ) ) ;
#8755=ORIENTED_EDGE ( 'NONE', *, *, #22243, .F. ) ;
#8765=DIRECTION ( 'NONE',  ( 1.000000000000000000, 0.000000000000000000, 0.000000000000000000 ) ) ;
#8767=ORIENTED_EDGE ( 'NONE', *, *, #3492, .F. ) ;
#8779=EDGE_CURVE ( 'NONE', #11908, #37911, #4717, .T. ) ;
#8782=CARTESIAN_POINT ( 'NONE',  ( -4.248748702180636272, -26.64985754041175525, 6.700000000000000178 ) ) ;
#8785=VERTEX_POINT ( 'NONE', #2051 ) ;
#8794=VERTEX_POINT ( 'NONE', #17251 ) ;
#8798=ADVANCED_FACE ( 'NONE', ( #20546 ), #33130, .F. ) ;
#8805=AXIS2_PLACEMENT_3D ( 'NONE', #23935, #2144, #18166 ) ;
#8818=CIRCLE ( 'NONE', #1616, 0.1000000000000028644 ) ;
#8819=ORIENTED_EDGE ( 'NONE', *, *, #5963, .F. ) ;
#8820=ORIENTED_EDGE ( 'NONE', *, *, #28455, .T. ) ;
#8835=DIRECTION ( 'NONE',  ( -0.000000000000000000, -0.000000000000000000, 1.000000000000000000 ) ) ;
#8838=CIRCLE ( 'NONE', #39764, 0.1000000000000028644 ) ;
#8841=CARTESIAN_POINT ( 'NONE',  ( -22.34874870218063947, -26.64985754041175525, 6.700000000000000178 ) ) ;
#8842=ORIENTED_EDGE ( 'NONE', *, *, #5864, .T. ) ;
#8851=FACE_OUTER_BOUND ( 'NONE', #32897, .T. ) ;
#8856=CARTESIAN_POINT ( 'NONE',  ( -29.07867591359219617, -26.64985754041175525, 6.800000000000000711 ) ) ;
#8863=LINE ( 'NONE', #28213, #19870 ) ;
#8865=DIRECTION ( 'NONE',  ( 0.000000000000000000, 0.000000000000000000, 1.000000000000000000 ) ) ;
#8868=CIRCLE ( 'NONE', #23374, 0.1000000000000028644 ) ;
#8869=ORIENTED_EDGE ( 'NONE', *, *, #6850, .T. ) ;
#8870=CIRCLE ( 'NONE', #388, 0.1000000000000028644 ) ;
#8878=EDGE_LOOP ( 'NONE', ( #3088, #34509, #27256, #19959 ) ) ;
#8886=DIRECTION ( 'NONE',  ( 0.000000000000000000, 0.000000000000000000, 1.000000000000000000 ) ) ;
#8891=DIRECTION ( 'NONE',  ( 1.000000000000000000, 0.000000000000000000, 0.000000000000000000 ) ) ;
#8903=AXIS2_PLACEMENT_3D ( 'NONE', #34781, #5731, #3084 ) ;
#8904=CARTESIAN_POINT ( 'NONE',  ( -26.24874870218063450, -25.49307895267003587, 6.700000000000000178 ) ) ;
#8905=VECTOR ( 'NONE', #13336, 1000.000000000000000 ) ;
#8906=CARTESIAN_POINT ( 'NONE',  ( -14.97867591359219119, -24.55319635012989110, 6.800000000000000711 ) ) ;
#8918=ORIENTED_EDGE ( 'NONE', *, *, #16229, .F. ) ;
#8919=ORIENTED_EDGE ( 'NONE', *, *, #10458, .T. ) ;
#8921=EDGE_CURVE ( 'NONE', #38495, #1346, #18068, .T. ) ;
#8926=LINE ( 'NONE', #21300, #22866 ) ;
#8930=CARTESIAN_POINT ( 'NONE',  ( -14.44874870218064089, -26.64985754041175525, 6.700000000000000178 ) ) ;
#8931=VERTEX_POINT ( 'NONE', #27549 ) ;
#8935=ORIENTED_EDGE ( 'NONE', *, *, #14435, .F. ) ;
#8936=ORIENTED_EDGE ( 'NONE', *, *, #25950, .F. ) ;
#8956=CARTESIAN_POINT ( 'NONE',  ( -14.44874870218064089, -26.64985754041175525, 6.800000000000000711 ) ) ;
#8961=CIRCLE ( 'NONE', #4387, 2.000000000000000000 ) ;
#8965=AXIS2_PLACEMENT_3D ( 'NONE', #39744, #18318, #6552 ) ;
#8969=EDGE_CURVE ( 'NONE', #5530, #33055, #14991, .T. ) ;
#8970=DIRECTION ( 'NONE',  ( 1.000000000000000000, 0.000000000000000000, 0.000000000000000000 ) ) ;
#8974=EDGE_LOOP ( 'NONE', ( #2386, #20118, #15802, #36932 ) ) ;
#8977=EDGE_LOOP ( 'NONE', ( #12312, #38255, #33167, #35120 ) ) ;
#8986=VERTEX_POINT ( 'NONE', #9215 ) ;
#8996=ADVANCED_FACE ( 'NONE', ( #31063 ), #6355, .F. ) ;
#8997=VECTOR ( 'NONE', #26192, 1000.000000000000000 ) ;
#9011=CARTESIAN_POINT ( 'NONE',  ( -24.44874870218064089, -26.64985754041175525, 6.800000000000000711 ) ) ;
#9016=ORIENTED_EDGE ( 'NONE', *, *, #10230, .F. ) ;
#9030=DIRECTION ( 'NONE',  ( 1.000000000000000000, 0.000000000000000000, -0.000000000000000000 ) ) ;
#9031=ORIENTED_EDGE ( 'NONE', *, *, #9858, .T. ) ;
#9032=ORIENTED_EDGE ( 'NONE', *, *, #37591, .F. ) ;
#9035=ORIENTED_EDGE ( 'NONE', *, *, #11696, .T. ) ;
#9043=DIRECTION ( 'NONE',  ( 1.000000000000000000, 0.000000000000000000, 0.000000000000000000 ) ) ;
#9044=LINE ( 'NONE', #22248, #35635 ) ;
#9047=ADVANCED_FACE ( 'NONE', ( #15190 ), #40302, .F. ) ;
#9049=ORIENTED_EDGE ( 'NONE', *, *, #38297, .F. ) ;
#9053=VERTEX_POINT ( 'NONE', #34784 ) ;
#9063=ADVANCED_FACE ( 'NONE', ( #4088 ), #3897, .F. ) ;
#9069=CARTESIAN_POINT ( 'NONE',  ( -15.07867591359219439, -26.64985754041175525, 6.700000000000000178 ) ) ;
#9072=ORIENTED_EDGE ( 'NONE', *, *, #14164, .T. ) ;
#9074=CIRCLE ( 'NONE', #1207, 0.1000000000000028644 ) ;
#9076=ORIENTED_EDGE ( 'NONE', *, *, #16362, .F. ) ;
#9079=VERTEX_POINT ( 'NONE', #16215 ) ;
#9083=ORIENTED_EDGE ( 'NONE', *, *, #39130, .F. ) ;
#9084=FACE_OUTER_BOUND ( 'NONE', #2168, .T. ) ;
#9090=FACE_OUTER_BOUND ( 'NONE', #3968, .T. ) ;
#9097=DIRECTION ( 'NONE',  ( -0.000000000000000000, -1.000000000000000000, -0.000000000000000000 ) ) ;
#9101=VERTEX_POINT ( 'NONE', #993 ) ;
#9108=AXIS2_PLACEMENT_3D ( 'NONE', #37156, #21931, #2807 ) ;
#9115=EDGE_CURVE ( 'NONE', #18951, #4028, #38637, .T. ) ;
#9116=DIRECTION ( 'NONE',  ( 0.000000000000000000, 0.000000000000000000, 1.000000000000000000 ) ) ;
#9123=DIRECTION ( 'NONE',  ( 1.000000000000000000, 0.000000000000000000, 0.000000000000000000 ) ) ;
#9125=CARTESIAN_POINT ( 'NONE',  ( -18.44874870218064089, -26.64985754041175525, 6.700000000000000178 ) ) ;
#9132=LINE ( 'NONE', #28071, #11971 ) ;
#9134=EDGE_LOOP ( 'NONE', ( #16550, #7961, #39049, #21917 ) ) ;
#9136=DIRECTION ( 'NONE',  ( 0.000000000000000000, 1.000000000000000000, 0.000000000000000000 ) ) ;
#9140=ORIENTED_EDGE ( 'NONE', *, *, #20394, .T. ) ;
#9150=EDGE_CURVE ( 'NONE', #17955, #6604, #24343, .T. ) ;
#9179=AXIS2_PLACEMENT_3D ( 'NONE', #30636, #30005, #33722 ) ;
#9190=ORIENTED_EDGE ( 'NONE', *, *, #40021, .T. ) ;
#9207=DIRECTION ( 'NONE',  ( -0.000000000000000000, -0.000000000000000000, -1.000000000000000000 ) ) ;
#9215=CARTESIAN_POINT ( 'NONE',  ( -12.87867591359218977, -24.55319635012989110, 6.800000000000000711 ) ) ;
#9219=PLANE ( 'NONE',  #21381 ) ;
#9223=ORIENTED_EDGE ( 'NONE', *, *, #4492, .T. ) ;
#9228=DIRECTION ( 'NONE',  ( -0.000000000000000000, -1.000000000000000000, -0.000000000000000000 ) ) ;
#9230=AXIS2_PLACEMENT_3D ( 'NONE', #33191, #4977, #17505 ) ;
#9234=VERTEX_POINT ( 'NONE', #31017 ) ;
#9238=ORIENTED_EDGE ( 'NONE', *, *, #20266, .T. ) ;
#9241=VERTEX_POINT ( 'NONE', #33699 ) ;
#9244=FACE_OUTER_BOUND ( 'NONE', #38250, .T. ) ;
#9246=CARTESIAN_POINT ( 'NONE',  ( -42.83131703149249603, -32.06993018339340296, 6.800000000000000711 ) ) ;
#9247=LINE ( 'NONE', #15639, #17196 ) ;
#9254=ADVANCED_FACE ( 'NONE', ( #2826 ), #27506, .F. ) ;
#9256=DIRECTION ( 'NONE',  ( 0.000000000000000000, 0.000000000000000000, 1.000000000000000000 ) ) ;
#9267=CIRCLE ( 'NONE', #35601, 0.1000000000000028644 ) ;
#9275=ORIENTED_EDGE ( 'NONE', *, *, #15019, .T. ) ;
#9278=ORIENTED_EDGE ( 'NONE', *, *, #15718, .F. ) ;
#9282=FACE_BOUND ( 'NONE', #21815, .T. ) ;
#9283=CARTESIAN_POINT ( 'NONE',  ( -28.97867591359219475, -26.64985754041175525, 6.800000000000000711 ) ) ;
#9287=CARTESIAN_POINT ( 'NONE',  ( -22.24874870218063450, -26.64985754041175525, 6.700000000000000178 ) ) ;
#9288=EDGE_CURVE ( 'NONE', #33732, #23016, #32908, .T. ) ;
#9294=DIRECTION ( 'NONE',  ( 0.000000000000000000, 1.000000000000000000, 0.000000000000000000 ) ) ;
#9299=DIRECTION ( 'NONE',  ( -0.000000000000000000, -1.000000000000000000, -0.000000000000000000 ) ) ;
#9311=DIRECTION ( 'NONE',  ( 0.000000000000000000, 0.000000000000000000, 1.000000000000000000 ) ) ;
#9321=CARTESIAN_POINT ( 'NONE',  ( -6.448748702180637338, -26.64985754041175525, 6.800000000000000711 ) ) ;
#9333=EDGE_CURVE ( 'NONE', #1149, #12703, #40057, .T. ) ;
#9341=FACE_OUTER_BOUND ( 'NONE', #28842, .T. ) ;
#9351=FACE_OUTER_BOUND ( 'NONE', #19539, .T. ) ;
#9353=DIRECTION ( 'NONE',  ( -0.000000000000000000, -0.000000000000000000, 1.000000000000000000 ) ) ;
#9354=VERTEX_POINT ( 'NONE', #19060 ) ;
#9364=CARTESIAN_POINT ( 'NONE',  ( -27.07867591359219972, -24.55319635012989110, 6.700000000000000178 ) ) ;
#9366=CARTESIAN_POINT ( 'NONE',  ( 5.751251297819365504, -26.64985754041175525, 6.700000000000000178 ) ) ;
#9368=EDGE_CURVE ( 'NONE', #10291, #36291, #19669, .T. ) ;
#9373=ORIENTED_EDGE ( 'NONE', *, *, #34809, .F. ) ;
#9377=ADVANCED_FACE ( 'NONE', ( #19863 ), #31623, .F. ) ;
#9382=ORIENTED_EDGE ( 'NONE', *, *, #16102, .F. ) ;
#9386=ORIENTED_EDGE ( 'NONE', *, *, #16134, .F. ) ;
#9391=FACE_OUTER_BOUND ( 'NONE', #19485, .T. ) ;
#9395=VERTEX_POINT ( 'NONE', #34734 ) ;
#9396=ORIENTED_EDGE ( 'NONE', *, *, #22057, .F. ) ;
#9398=LINE ( 'NONE', #27936, #5199 ) ;
#9409=CARTESIAN_POINT ( 'NONE',  ( -20.24874870218063805, -26.64985754041175525, 6.700000000000000178 ) ) ;
#9410=VERTEX_POINT ( 'NONE', #28732 ) ;
#9411=DIRECTION ( 'NONE',  ( 1.000000000000000000, 0.000000000000000000, -0.000000000000000000 ) ) ;
#9412=DIRECTION ( 'NONE',  ( 1.000000000000000000, -0.000000000000000000, 0.000000000000000000 ) ) ;
#9425=DIRECTION ( 'NONE',  ( -0.000000000000000000, -1.000000000000000000, -0.000000000000000000 ) ) ;
#9428=EDGE_CURVE ( 'NONE', #36848, #2698, #38586, .T. ) ;
#9431=ADVANCED_FACE ( 'NONE', ( #25847 ), #22369, .T. ) ;
#9432=ORIENTED_EDGE ( 'NONE', *, *, #7304, .T. ) ;
#9438=EDGE_LOOP ( 'NONE', ( #34567, #6371, #37261, #19880 ) ) ;
#9444=CARTESIAN_POINT ( 'NONE',  ( -12.24874870218063627, -26.64985754041175525, 6.700000000000000178 ) ) ;
#9446=LINE ( 'NONE', #25517, #28800 ) ;
#9447=CIRCLE ( 'NONE', #1588, 0.1000000000000028644 ) ;
#9454=ORIENTED_EDGE ( 'NONE', *, *, #35743, .T. ) ;
#9457=VERTEX_POINT ( 'NONE', #13275 ) ;
#9461=ORIENTED_EDGE ( 'NONE', *, *, #1726, .F. ) ;
#9471=ORIENTED_EDGE ( 'NONE', *, *, #2873, .T. ) ;
#9476=EDGE_LOOP ( 'NONE', ( #9031, #13337, #40354, #22529 ) ) ;
#9480=VERTEX_POINT ( 'NONE', #547 ) ;
#9485=DIRECTION ( 'NONE',  ( 0.000000000000000000, 0.000000000000000000, 1.000000000000000000 ) ) ;
#9487=VERTEX_POINT ( 'NONE', #16559 ) ;
#9488=FACE_BOUND ( 'NONE', #39871, .T. ) ;
#9495=AXIS2_PLACEMENT_3D ( 'NONE', #19450, #19246, #18833 ) ;
#9508=CARTESIAN_POINT ( 'NONE',  ( -24.87867591359218977, -24.55319635012989110, 6.800000000000000711 ) ) ;
#9514=EDGE_CURVE ( 'NONE', #9410, #3866, #35338, .T. ) ;
#9515=DIRECTION ( 'NONE',  ( 0.000000000000000000, 0.000000000000000000, 1.000000000000000000 ) ) ;
#9516=FACE_OUTER_BOUND ( 'NONE', #10797, .T. ) ;
#9520=LINE ( 'NONE', #6455, #25620 ) ;
#9528=ADVANCED_FACE ( 'NONE', ( #10392 ), #28528, .F. ) ;
#9532=DIRECTION ( 'NONE',  ( -0.000000000000000000, -0.000000000000000000, 1.000000000000000000 ) ) ;
#9534=ORIENTED_EDGE ( 'NONE', *, *, #34294, .F. ) ;
#9535=EDGE_LOOP ( 'NONE', ( #25708, #22393, #23264, #37698 ) ) ;
#9536=CARTESIAN_POINT ( 'NONE',  ( -53.21549048184568420, -38.28842912540938670, 4.000000000000000000 ) ) ;
#9539=ORIENTED_EDGE ( 'NONE', *, *, #36865, .F. ) ;
#9540=DIRECTION ( 'NONE',  ( -0.000000000000000000, -1.000000000000000000, -0.000000000000000000 ) ) ;
#9541=DIRECTION ( 'NONE',  ( 0.000000000000000000, 1.000000000000000000, 0.000000000000000000 ) ) ;
#9547=ORIENTED_EDGE ( 'NONE', *, *, #7574, .T. ) ;
#9559=AXIS2_PLACEMENT_3D ( 'NONE', #13977, #19955, #32737 ) ;
#9560=AXIS2_PLACEMENT_3D ( 'NONE', #21767, #34350, #34147 ) ;
#9563=EDGE_LOOP ( 'NONE', ( #12441, #23352, #6780, #35383 ) ) ;
#9570=VECTOR ( 'NONE', #20305, 1000.000000000000000 ) ;
#9577=DIRECTION ( 'NONE',  ( -0.000000000000000000, -0.000000000000000000, 1.000000000000000000 ) ) ;
#9581=EDGE_CURVE ( 'NONE', #25156, #25120, #11384, .T. ) ;
#9585=LINE ( 'NONE', #19673, #26871 ) ;
#9592=EDGE_CURVE ( 'NONE', #33929, #8738, #14077, .T. ) ;
#9600=DIRECTION ( 'NONE',  ( 0.000000000000000000, 0.000000000000000000, 1.000000000000000000 ) ) ;
#9629=ADVANCED_FACE ( 'NONE', ( #23950 ), #10781, .F. ) ;
#9635=AXIS2_PLACEMENT_3D ( 'NONE', #16683, #13613, #10516 ) ;
#9649=ORIENTED_EDGE ( 'NONE', *, *, #7946, .F. ) ;
#9655=VERTEX_POINT ( 'NONE', #20067 ) ;
#9660=CARTESIAN_POINT ( 'NONE',  ( -22.97867591359219119, -26.64985754041175525, 6.800000000000000711 ) ) ;
#9661=DIRECTION ( 'NONE',  ( 0.000000000000000000, 0.000000000000000000, 1.000000000000000000 ) ) ;
#9666=EDGE_LOOP ( 'NONE', ( #38219, #93, #11869, #32160 ) ) ;
#9676=ADVANCED_FACE ( 'NONE', ( #24576 ), #40213, .F. ) ;
#9679=AXIS2_PLACEMENT_3D ( 'NONE', #24924, #9256, #34413 ) ;
#9685=CARTESIAN_POINT ( 'NONE',  ( -1.078675913592196167, -24.55319635012989110, 6.800000000000000711 ) ) ;
#9686=VERTEX_POINT ( 'NONE', #12425 ) ;
#9691=DIRECTION ( 'NONE',  ( 1.000000000000000000, 0.000000000000000000, -0.000000000000000000 ) ) ;
#9709=PLANE ( 'NONE',  #29834 ) ;
#9713=LINE ( 'NONE', #18771, #22387 ) ;
#9733=EDGE_CURVE ( 'NONE', #6110, #38497, #36724, .T. ) ;
#9734=CARTESIAN_POINT ( 'NONE',  ( -36.87867591359218977, -24.55319635012989110, 6.700000000000000178 ) ) ;
#9739=DIRECTION ( 'NONE',  ( -0.000000000000000000, -0.000000000000000000, 1.000000000000000000 ) ) ;
#9740=VECTOR ( 'NONE', #19696, 1000.000000000000000 ) ;
#9743=CARTESIAN_POINT ( 'NONE',  ( -36.24874870218063450, -26.64985754041175525, 6.700000000000000178 ) ) ;
#9750=VERTEX_POINT ( 'NONE', #8504 ) ;
#9754=DIRECTION ( 'NONE',  ( 0.000000000000000000, 0.000000000000000000, 1.000000000000000000 ) ) ;
#9760=EDGE_LOOP ( 'NONE', ( #23476, #12729, #13998, #5770 ) ) ;
#9777=DIRECTION ( 'NONE',  ( 0.000000000000000000, 0.000000000000000000, 1.000000000000000000 ) ) ;
#9779=EDGE_CURVE ( 'NONE', #11094, #27559, #21088, .T. ) ;
#9784=CARTESIAN_POINT ( 'NONE',  ( -16.97867591359219475, -26.64985754041175525, 6.800000000000000711 ) ) ;
#9785=CARTESIAN_POINT ( 'NONE',  ( -36.97867591359219119, -24.55319635012989110, 6.800000000000000711 ) ) ;
#9790=AXIS2_PLACEMENT_3D ( 'NONE', #29266, #35854, #4365 ) ;
#9799=EDGE_CURVE ( 'NONE', #33660, #30400, #30282, .T. ) ;
#9804=DIRECTION ( 'NONE',  ( -0.000000000000000000, -0.000000000000000000, 1.000000000000000000 ) ) ;
#9805=UNCERTAINTY_MEASURE_WITH_UNIT (LENGTH_MEASURE( 1.000000000000000082E-05 ), #32556, 'distance_accuracy_value', 'NONE');
#9810=LINE ( 'NONE', #40688, #18755 ) ;
#9812=LINE ( 'NONE', #19690, #38771 ) ;
#9813=ORIENTED_EDGE ( 'NONE', *, *, #10460, .T. ) ;
#9814=ADVANCED_FACE ( 'NONE', ( #33861 ), #18183, .F. ) ;
#9816=CIRCLE ( 'NONE', #13757, 0.1000000000000028644 ) ;
#9823=ORIENTED_EDGE ( 'NONE', *, *, #16324, .T. ) ;
#9824=CARTESIAN_POINT ( 'NONE',  ( -40.24874870218063450, -25.49307895267003587, 6.700000000000000178 ) ) ;
#9836=VECTOR ( 'NONE', #25586, 1000.000000000000000 ) ;
#9843=EDGE_CURVE ( 'NONE', #12335, #6115, #3795, .T. ) ;
#9846=ORIENTED_EDGE ( 'NONE', *, *, #36271, .F. ) ;
#9848=CARTESIAN_POINT ( 'NONE',  ( -27.07867591359219972, -26.64985754041175525, 6.800000000000000711 ) ) ;
#9850=CARTESIAN_POINT ( 'NONE',  ( -2.878675913592191993, -26.64985754041175525, 6.700000000000000178 ) ) ;
#9851=ORIENTED_EDGE ( 'NONE', *, *, #26830, .F. ) ;
#9858=EDGE_CURVE ( 'NONE', #21608, #6003, #29636, .T. ) ;
#9864=EDGE_CURVE ( 'NONE', #13694, #2784, #21903, .T. ) ;
#9866=CIRCLE ( 'NONE', #36804, 0.1000000000000028644 ) ;
#9874=CARTESIAN_POINT ( 'NONE',  ( -36.44874870218064444, -26.64985754041175525, 6.800000000000000711 ) ) ;
#9875=ORIENTED_EDGE ( 'NONE', *, *, #35862, .F. ) ;
#9882=ORIENTED_EDGE ( 'NONE', *, *, #3669, .F. ) ;
#9891=DIRECTION ( 'NONE',  ( 0.000000000000000000, 0.000000000000000000, 1.000000000000000000 ) ) ;
#9893=ORIENTED_EDGE ( 'NONE', *, *, #27699, .F. ) ;
#9894=EDGE_LOOP ( 'NONE', ( #20988, #34417, #19653, #37205 ) ) ;
#9901=CIRCLE ( 'NONE', #20408, 0.1000000000000028644 ) ;
#9902=PLANE ( 'NONE',  #39710 ) ;
#9904=EDGE_LOOP ( 'NONE', ( #23926, #11041, #29009, #8401 ) ) ;
#9905=FACE_BOUND ( 'NONE', #8013, .T. ) ;
#9909=ADVANCED_FACE ( 'NONE', ( #23515 ), #26601, .F. ) ;
#9946=AXIS2_PLACEMENT_3D ( 'NONE', #13375, #1448, #23068 ) ;
#9948=DIRECTION ( 'NONE',  ( 0.000000000000000000, 1.000000000000000000, 0.000000000000000000 ) ) ;
#9956=ADVANCED_FACE ( 'NONE', ( #29884 ), #29291, .F. ) ;
#9960=ADVANCED_FACE ( 'NONE', ( #13638 ), #32988, .F. ) ;
#9965=CARTESIAN_POINT ( 'NONE',  ( -0.4487487021806388365, -26.64985754041175525, 6.700000000000000178 ) ) ;
#9976=CARTESIAN_POINT ( 'NONE',  ( 3.551251297819357777, -25.49307895267003587, 6.700000000000000178 ) ) ;
#9977=ORIENTED_EDGE ( 'NONE', *, *, #2580, .T. ) ;
#9979=LINE ( 'NONE', #35922, #6559 ) ;
#9986=DIRECTION ( 'NONE',  ( 0.000000000000000000, 0.000000000000000000, 1.000000000000000000 ) ) ;
#9987=DIRECTION ( 'NONE',  ( -0.000000000000000000, -0.000000000000000000, 1.000000000000000000 ) ) ;
#9989=CIRCLE ( 'NONE', #33006, 0.1000000000000028644 ) ;
#9992=ORIENTED_EDGE ( 'NONE', *, *, #29445, .T. ) ;
#9996=ORIENTED_EDGE ( 'NONE', *, *, #15587, .F. ) ;
#10001=LINE ( 'NONE', #31440, #13654 ) ;
#10003=ORIENTED_EDGE ( 'NONE', *, *, #21855, .F. ) ;
#10008=VERTEX_POINT ( 'NONE', #4583 ) ;
#10009=DIRECTION ( 'NONE',  ( -0.000000000000000000, -0.000000000000000000, 1.000000000000000000 ) ) ;
#10011=DIRECTION ( 'NONE',  ( 0.000000000000000000, 0.000000000000000000, -1.000000000000000000 ) ) ;
#10014=ORIENTED_EDGE ( 'NONE', *, *, #38061, .F. ) ;
#10029=EDGE_CURVE ( 'NONE', #23121, #37478, #23312, .T. ) ;
#10035=ORIENTED_EDGE ( 'NONE', *, *, #28665, .T. ) ;
#10038=VECTOR ( 'NONE', #39625, 1000.000000000000000 ) ;
#10039=EDGE_CURVE ( 'NONE', #28543, #2729, #27664, .T. ) ;
#10041=FACE_OUTER_BOUND ( 'NONE', #11554, .T. ) ;
#10049=FACE_OUTER_BOUND ( 'NONE', #34835, .T. ) ;
#10050=ORIENTED_EDGE ( 'NONE', *, *, #35862, .T. ) ;
#10057=ORIENTED_EDGE ( 'NONE', *, *, #16606, .F. ) ;
#10070=ORIENTED_EDGE ( 'NONE', *, *, #17372, .F. ) ;
#10071=DIRECTION ( 'NONE',  ( 0.000000000000000000, 0.000000000000000000, 1.000000000000000000 ) ) ;
#10084=EDGE_CURVE ( 'NONE', #13148, #273, #17110, .T. ) ;
#10087=ADVANCED_FACE ( 'NONE', ( #10731 ), #11133, .T. ) ;
#10089=AXIS2_PLACEMENT_3D ( 'NONE', #26451, #24159, #4822 ) ;
#10095=DIRECTION ( 'NONE',  ( 0.000000000000000000, 0.000000000000000000, 1.000000000000000000 ) ) ;
#10099=VERTEX_POINT ( 'NONE', #27606 ) ;
#10100=FACE_BOUND ( 'NONE', #39696, .T. ) ;
#10101=ORIENTED_EDGE ( 'NONE', *, *, #40018, .F. ) ;
#10108=DIRECTION ( 'NONE',  ( 0.000000000000000000, 0.000000000000000000, -1.000000000000000000 ) ) ;
#10122=DIRECTION ( 'NONE',  ( 1.000000000000000000, -0.000000000000000000, 0.000000000000000000 ) ) ;
#10127=VECTOR ( 'NONE', #29860, 1000.000000000000000 ) ;
#10135=ORIENTED_EDGE ( 'NONE', *, *, #12129, .F. ) ;
#10136=CARTESIAN_POINT ( 'NONE',  ( -30.44874870218064089, -26.64985754041175525, 6.700000000000000178 ) ) ;
#10139=VERTEX_POINT ( 'NONE', #39963 ) ;
#10140=DIRECTION ( 'NONE',  ( -0.000000000000000000, -0.000000000000000000, 1.000000000000000000 ) ) ;
#10149=VECTOR ( 'NONE', #30288, 1000.000000000000000 ) ;
#10153=ORIENTED_EDGE ( 'NONE', *, *, #20133, .F. ) ;
#10170=CIRCLE ( 'NONE', #15434, 0.1000000000000028644 ) ;
#10181=CARTESIAN_POINT ( 'NONE',  ( -8.878675913592189772, -24.55319635012989110, 6.800000000000000711 ) ) ;
#10182=ADVANCED_FACE ( 'NONE', ( #2933 ), #27199, .F. ) ;
#10185=DIRECTION ( 'NONE',  ( 0.000000000000000000, 0.000000000000000000, 1.000000000000000000 ) ) ;
#10188=EDGE_CURVE ( 'NONE', #9079, #744, #16468, .T. ) ;
#10190=ORIENTED_EDGE ( 'NONE', *, *, #29665, .F. ) ;
#10199=FACE_OUTER_BOUND ( 'NONE', #18199, .T. ) ;
#10203=VECTOR ( 'NONE', #29206, 1000.000000000000000 ) ;
#10209=AXIS2_PLACEMENT_3D ( 'NONE', #13746, #23215, #35779 ) ;
#10217=VERTEX_POINT ( 'NONE', #23896 ) ;
#10219=VERTEX_POINT ( 'NONE', #20814 ) ;
#10221=DIRECTION ( 'NONE',  ( 0.000000000000000000, 0.000000000000000000, 1.000000000000000000 ) ) ;
#10230=EDGE_CURVE ( 'NONE', #30840, #33369, #33597, .T. ) ;
#10231=VECTOR ( 'NONE', #20920, 1000.000000000000000 ) ;
#10242=DIRECTION ( 'NONE',  ( -0.000000000000000000, -0.000000000000000000, 1.000000000000000000 ) ) ;
#10249=LINE ( 'NONE', #20315, #12204 ) ;
#10252=VERTEX_POINT ( 'NONE', #3743 ) ;
#10254=DIRECTION ( 'NONE',  ( -1.000000000000000000, 0.000000000000000000, 0.000000000000000000 ) ) ;
#10257=ORIENTED_EDGE ( 'NONE', *, *, #27330, .T. ) ;
#10270=EDGE_LOOP ( 'NONE', ( #32656, #3801, #442, #2743 ) ) ;
#10273=VERTEX_POINT ( 'NONE', #31726 ) ;
#10277=ORIENTED_EDGE ( 'NONE', *, *, #14671, .F. ) ;
#10283=ADVANCED_FACE ( 'NONE', ( #16068 ), #28839, .T. ) ;
#10289=CARTESIAN_POINT ( 'NONE',  ( -20.44874870218064444, -26.64985754041175525, 6.700000000000000178 ) ) ;
#10291=VERTEX_POINT ( 'NONE', #3147 ) ;
#10292=ORIENTED_EDGE ( 'NONE', *, *, #19440, .F. ) ;
#10295=AXIS2_PLACEMENT_3D ( 'NONE', #17128, #26227, #7472 ) ;
#10298=AXIS2_PLACEMENT_3D ( 'NONE', #33792, #24507, #2296 ) ;
#10304=EDGE_CURVE ( 'NONE', #39924, #39141, #5301, .T. ) ;
#10309=VERTEX_POINT ( 'NONE', #21848 ) ;
#10311=DIRECTION ( 'NONE',  ( -0.000000000000000000, -0.000000000000000000, 1.000000000000000000 ) ) ;
#10313=DIRECTION ( 'NONE',  ( 0.000000000000000000, 0.000000000000000000, -1.000000000000000000 ) ) ;
#10314=ADVANCED_FACE ( 'NONE', ( #22467 ), #15660, .T. ) ;
#10319=DIRECTION ( 'NONE',  ( 0.000000000000000000, 0.000000000000000000, 1.000000000000000000 ) ) ;
#10344=DIRECTION ( 'NONE',  ( -0.000000000000000000, -0.000000000000000000, 1.000000000000000000 ) ) ;
#10347=DIRECTION ( 'NONE',  ( 0.000000000000000000, 1.000000000000000000, 0.000000000000000000 ) ) ;
#10349=ADVANCED_FACE ( 'NONE', ( #439 ), #6612, .F. ) ;
#10352=CYLINDRICAL_SURFACE ( 'NONE', #27865, 0.1000000000000028644 ) ;
#10360=EDGE_LOOP ( 'NONE', ( #12598, #340, #15055, #32572 ) ) ;
#10365=VERTEX_POINT ( 'NONE', #19575 ) ;
#10369=EDGE_CURVE ( 'NONE', #37105, #19656, #26359, .T. ) ;
#10373=CARTESIAN_POINT ( 'NONE',  ( -1.078675913592196167, -26.64985754041175525, 6.700000000000000178 ) ) ;
#10376=AXIS2_PLACEMENT_3D ( 'NONE', #20737, #24025, #18050 ) ;
#10388=DIRECTION ( 'NONE',  ( 0.000000000000000000, 0.000000000000000000, 1.000000000000000000 ) ) ;
#10390=CARTESIAN_POINT ( 'NONE',  ( -33.07867591359219972, -26.64985754041175525, 6.700000000000000178 ) ) ;
#10392=FACE_OUTER_BOUND ( 'NONE', #16969, .T. ) ;
#10397=ORIENTED_EDGE ( 'NONE', *, *, #17999, .T. ) ;
#10404=EDGE_CURVE ( 'NONE', #21932, #21394, #36219, .T. ) ;
#10408=DIRECTION ( 'NONE',  ( 0.000000000000000000, 0.000000000000000000, 1.000000000000000000 ) ) ;
#10410=EDGE_CURVE ( 'NONE', #13769, #28407, #17260, .T. ) ;
#10416=CIRCLE ( 'NONE', #570, 0.1000000000000028644 ) ;
#10418=EDGE_CURVE ( 'NONE', #28407, #3677, #14511, .T. ) ;
#10419=DIRECTION ( 'NONE',  ( 1.000000000000000000, 0.000000000000000000, 0.000000000000000000 ) ) ;
#10420=LINE ( 'NONE', #16393, #9740 ) ;
#10425=FACE_OUTER_BOUND ( 'NONE', #11359, .T. ) ;
#10428=AXIS2_PLACEMENT_3D ( 'NONE', #1478, #39123, #16346 ) ;
#10446=ORIENTED_EDGE ( 'NONE', *, *, #10418, .F. ) ;
#10447=CARTESIAN_POINT ( 'NONE',  ( 2.921324086407800280, -26.64985754041175525, 6.800000000000000711 ) ) ;
#10456=ORIENTED_EDGE ( 'NONE', *, *, #3427, .F. ) ;
#10457=EDGE_CURVE ( 'NONE', #13597, #33969, #32746, .T. ) ;
#10458=EDGE_CURVE ( 'NONE', #39035, #25329, #846, .T. ) ;
#10460=EDGE_CURVE ( 'NONE', #30200, #34241, #34960, .T. ) ;
#10463=DIRECTION ( 'NONE',  ( 1.000000000000000000, 0.000000000000000000, 0.000000000000000000 ) ) ;
#10480=VECTOR ( 'NONE', #21013, 1000.000000000000000 ) ;
#10487=DIRECTION ( 'NONE',  ( 1.000000000000000000, 0.000000000000000000, 0.000000000000000000 ) ) ;
#10500=ORIENTED_EDGE ( 'NONE', *, *, #17745, .T. ) ;
#10506=AXIS2_PLACEMENT_3D ( 'NONE', #6908, #25241, #38379 ) ;
#10507=PLANE ( 'NONE',  #11417 ) ;
#10516=DIRECTION ( 'NONE',  ( 1.000000000000000000, 0.000000000000000000, 0.000000000000000000 ) ) ;
#10526=CARTESIAN_POINT ( 'NONE',  ( 11.65737507970504439, -27.06993018339339940, 6.000000000000000000 ) ) ;
#10531=DIRECTION ( 'NONE',  ( 0.000000000000000000, 0.000000000000000000, 1.000000000000000000 ) ) ;
#10536=CIRCLE ( 'NONE', #33579, 0.1000000000000028644 ) ;
#10543=ADVANCED_FACE ( 'NONE', ( #26754 ), #20358, .T. ) ;
#10551=DIRECTION ( 'NONE',  ( 0.000000000000000000, 0.000000000000000000, -1.000000000000000000 ) ) ;
#10554=AXIS2_PLACEMENT_3D ( 'NONE', #22058, #34633, #9691 ) ;
#10559=EDGE_CURVE ( 'NONE', #13946, #8281, #17161, .T. ) ;
#10568=VECTOR ( 'NONE', #27239, 1000.000000000000000 ) ;
#10571=ORIENTED_EDGE ( 'NONE', *, *, #24100, .T. ) ;
#10577=EDGE_CURVE ( 'NONE', #9234, #25156, #7303, .T. ) ;
#10583=DIRECTION ( 'NONE',  ( 1.000000000000000000, -0.000000000000000000, 0.000000000000000000 ) ) ;
#10596=DIRECTION ( 'NONE',  ( -0.000000000000000000, -0.000000000000000000, 1.000000000000000000 ) ) ;
#10603=ORIENTED_EDGE ( 'NONE', *, *, #26458, .F. ) ;
#10608=DIRECTION ( 'NONE',  ( -0.000000000000000000, -0.000000000000000000, 1.000000000000000000 ) ) ;
#10634=DIRECTION ( 'NONE',  ( 0.000000000000000000, 0.000000000000000000, 1.000000000000000000 ) ) ;
#10637=EDGE_CURVE ( 'NONE', #38489, #36027, #8275, .T. ) ;
#10646=CARTESIAN_POINT ( 'NONE',  ( -17.07867591359219617, -26.64985754041175525, 6.800000000000000711 ) ) ;
#10651=DIRECTION ( 'NONE',  ( -0.000000000000000000, -1.000000000000000000, -0.000000000000000000 ) ) ;
#10655=ORIENTED_EDGE ( 'NONE', *, *, #16606, .T. ) ;
#10658=CARTESIAN_POINT ( 'NONE',  ( -34.97867591359219830, -24.55319635012989110, 6.700000000000000178 ) ) ;
#10695=ORIENTED_EDGE ( 'NONE', *, *, #13113, .T. ) ;
#10700=VERTEX_POINT ( 'NONE', #22998 ) ;
#10709=AXIS2_PLACEMENT_3D ( 'NONE', #27463, #15722, #2785 ) ;
#10711=CARTESIAN_POINT ( 'NONE',  ( -12.87867591359218977, -26.64985754041175525, 6.700000000000000178 ) ) ;
#10719=DIRECTION ( 'NONE',  ( -0.000000000000000000, -0.000000000000000000, 1.000000000000000000 ) ) ;
#10721=DIRECTION ( 'NONE',  ( -0.000000000000000000, -0.000000000000000000, 1.000000000000000000 ) ) ;
#10723=VECTOR ( 'NONE', #18222, 1000.000000000000000 ) ;
#10729=DIRECTION ( 'NONE',  ( 1.000000000000000000, 0.000000000000000000, 0.000000000000000000 ) ) ;
#10731=FACE_OUTER_BOUND ( 'NONE', #28723, .T. ) ;
#10733=ORIENTED_EDGE ( 'NONE', *, *, #15724, .F. ) ;
#10740=LINE ( 'NONE', #22924, #23949 ) ;
#10741=CARTESIAN_POINT ( 'NONE',  ( -4.248748702180636272, -26.64985754041175525, 6.800000000000000711 ) ) ;
#10742=DIRECTION ( 'NONE',  ( 0.000000000000000000, 1.000000000000000000, 0.000000000000000000 ) ) ;
#10743=DIRECTION ( 'NONE',  ( -0.000000000000000000, -0.000000000000000000, 1.000000000000000000 ) ) ;
#10746=ORIENTED_EDGE ( 'NONE', *, *, #19521, .F. ) ;
#10750=CIRCLE ( 'NONE', #8124, 0.1000000000000028644 ) ;
#10752=LINE ( 'NONE', #14451, #27834 ) ;
#10764=CARTESIAN_POINT ( 'NONE',  ( 5.121324086407808451, -24.55319635012989110, 6.700000000000000178 ) ) ;
#10768=EDGE_LOOP ( 'NONE', ( #18484, #25661, #25565, #8171 ) ) ;
#10772=FACE_OUTER_BOUND ( 'NONE', #2757, .T. ) ;
#10780=DIRECTION ( 'NONE',  ( -1.000000000000000000, 0.000000000000000000, 0.000000000000000000 ) ) ;
#10781=CYLINDRICAL_SURFACE ( 'NONE', #32937, 0.1000000000000028644 ) ;
#10783=AXIS2_PLACEMENT_3D ( 'NONE', #27233, #2353, #34059 ) ;
#10794=CARTESIAN_POINT ( 'NONE',  ( -6.348748702180634140, -25.49307895267003587, 6.700000000000000178 ) ) ;
#10797=EDGE_LOOP ( 'NONE', ( #9190, #849, #32815, #27219 ) ) ;
#10798=VERTEX_POINT ( 'NONE', #25377 ) ;
#10820=DIRECTION ( 'NONE',  ( -0.000000000000000000, -0.000000000000000000, 1.000000000000000000 ) ) ;
#10824=CARTESIAN_POINT ( 'NONE',  ( -9.078675913592196167, -26.64985754041175525, 6.800000000000000711 ) ) ;
#10825=PLANE ( 'NONE',  #915 ) ;
#10830=EDGE_CURVE ( 'NONE', #13769, #25932, #2555, .T. ) ;
#10837=VECTOR ( 'NONE', #14633, 1000.000000000000000 ) ;
#10846=CIRCLE ( 'NONE', #33899, 0.1000000000000028644 ) ;
#10850=CARTESIAN_POINT ( 'NONE',  ( -18.24874870218063450, -26.64985754041175525, 6.700000000000000178 ) ) ;
#10853=ORIENTED_EDGE ( 'NONE', *, *, #29445, .F. ) ;
#10863=EDGE_CURVE ( 'NONE', #7577, #38171, #27638, .T. ) ;
#10874=ORIENTED_EDGE ( 'NONE', *, *, #11318, .T. ) ;
#10885=DIRECTION ( 'NONE',  ( 0.000000000000000000, 0.000000000000000000, 1.000000000000000000 ) ) ;
#10894=CIRCLE ( 'NONE', #32442, 0.1000000000000028644 ) ;
#10898=VERTEX_POINT ( 'NONE', #15488 ) ;
#10905=CIRCLE ( 'NONE', #38504, 0.1000000000000028644 ) ;
#10910=LINE ( 'NONE', #36443, #20637 ) ;
#10912=CYLINDRICAL_SURFACE ( 'NONE', #27701, 0.1000000000000028644 ) ;
#10915=DIRECTION ( 'NONE',  ( -0.000000000000000000, -0.000000000000000000, 1.000000000000000000 ) ) ;
#10916=EDGE_CURVE ( 'NONE', #22571, #4144, #40178, .T. ) ;
#10921=FACE_OUTER_BOUND ( 'NONE', #430, .T. ) ;
#10928=ORIENTED_EDGE ( 'NONE', *, *, #28275, .F. ) ;
#10929=LINE ( 'NONE', #38527, #25051 ) ;
#10937=ORIENTED_EDGE ( 'NONE', *, *, #1378, .F. ) ;
#10943=DIRECTION ( 'NONE',  ( -0.000000000000000000, -1.000000000000000000, -0.000000000000000000 ) ) ;
#10947=CYLINDRICAL_SURFACE ( 'NONE', #6310, 0.1000000000000028644 ) ;
#10973=DIRECTION ( 'NONE',  ( 0.000000000000000000, 0.000000000000000000, 1.000000000000000000 ) ) ;
#10975=ORIENTED_EDGE ( 'NONE', *, *, #3300, .F. ) ;
#10994=DIRECTION ( 'NONE',  ( -0.000000000000000000, -0.000000000000000000, 1.000000000000000000 ) ) ;
#10995=DIRECTION ( 'NONE',  ( 0.000000000000000000, 0.000000000000000000, -1.000000000000000000 ) ) ;
#11007=CIRCLE ( 'NONE', #28136, 0.1000000000000028644 ) ;
#11009=ORIENTED_EDGE ( 'NONE', *, *, #35490, .T. ) ;
#11019=DIRECTION ( 'NONE',  ( 1.000000000000000000, 0.000000000000000000, 0.000000000000000000 ) ) ;
#11028=EDGE_CURVE ( 'NONE', #5443, #8785, #22287, .T. ) ;
#11041=ORIENTED_EDGE ( 'NONE', *, *, #10029, .T. ) ;
#11047=CARTESIAN_POINT ( 'NONE',  ( -12.34874870218063947, -26.64985754041175525, 6.800000000000000711 ) ) ;
#11058=FACE_OUTER_BOUND ( 'NONE', #30254, .T. ) ;
#11059=DIRECTION ( 'NONE',  ( -1.000000000000000000, 0.000000000000000000, 0.000000000000000000 ) ) ;
#11076=DIRECTION ( 'NONE',  ( 1.000000000000000000, 0.000000000000000000, 0.000000000000000000 ) ) ;
#11078=CARTESIAN_POINT ( 'NONE',  ( -52.01549048184568846, -30.38627270959228710, 4.800000000000000711 ) ) ;
#11083=AXIS2_PLACEMENT_3D ( 'NONE', #36393, #14754, #26727 ) ;
#11091=LINE ( 'NONE', #7815, #14546 ) ;
#11094=VERTEX_POINT ( 'NONE', #19902 ) ;
#11095=CARTESIAN_POINT ( 'NONE',  ( -38.24874870218063450, -25.49307895267003587, 6.700000000000000178 ) ) ;
#11099=FACE_OUTER_BOUND ( 'NONE', #31647, .T. ) ;
#11100=ORIENTED_EDGE ( 'NONE', *, *, #26415, .F. ) ;
#11103=DIRECTION ( 'NONE',  ( -0.000000000000000000, -1.000000000000000000, -0.000000000000000000 ) ) ;
#11106=ORIENTED_EDGE ( 'NONE', *, *, #26104, .F. ) ;
#11113=DIRECTION ( 'NONE',  ( 0.000000000000000000, 0.000000000000000000, -1.000000000000000000 ) ) ;
#11116=AXIS2_PLACEMENT_3D ( 'NONE', #10658, #7182, #29215 ) ;
#11127=DIRECTION ( 'NONE',  ( 0.000000000000000000, 0.000000000000000000, 1.000000000000000000 ) ) ;
#11129=CARTESIAN_POINT ( 'NONE',  ( -30.87867591359218977, -26.64985754041175525, 6.800000000000000711 ) ) ;
#11133=PLANE ( 'NONE',  #9230 ) ;
#11134=EDGE_CURVE ( 'NONE', #25426, #8794, #16999, .T. ) ;
#11135=ORIENTED_EDGE ( 'NONE', *, *, #13323, .T. ) ;
#11139=EDGE_CURVE ( 'NONE', #35057, #20163, #14337, .T. ) ;
#11148=LINE ( 'NONE', #8258, #30418 ) ;
#11172=DIRECTION ( 'NONE',  ( 1.000000000000000000, 0.000000000000000000, 0.000000000000000000 ) ) ;
#11180=DIRECTION ( 'NONE',  ( 0.000000000000000000, 0.000000000000000000, 1.000000000000000000 ) ) ;
#11181=DIRECTION ( 'NONE',  ( 0.000000000000000000, 0.000000000000000000, -1.000000000000000000 ) ) ;
#11184=CARTESIAN_POINT ( 'NONE',  ( -28.87867591359218977, -26.64985754041175525, 6.700000000000000178 ) ) ;
#11187=EDGE_CURVE ( 'NONE', #25932, #3811, #3033, .T. ) ;
#11188=ORIENTED_EDGE ( 'NONE', *, *, #22059, .T. ) ;
#11191=CARTESIAN_POINT ( 'NONE',  ( -2.248748702180634940, -26.64985754041175525, 6.800000000000000711 ) ) ;
#11194=CARTESIAN_POINT ( 'NONE',  ( -21.07867591359219617, -26.64985754041175525, 6.700000000000000178 ) ) ;
#11197=DIRECTION ( 'NONE',  ( -0.000000000000000000, -0.000000000000000000, 1.000000000000000000 ) ) ;
#11209=CARTESIAN_POINT ( 'NONE',  ( -34.44874870218064444, -26.64985754041175525, 6.800000000000000711 ) ) ;
#11218=DIRECTION ( 'NONE',  ( 1.000000000000000000, 0.000000000000000000, 0.000000000000000000 ) ) ;
#11219=CARTESIAN_POINT ( 'NONE',  ( -38.87867591359218977, -26.64985754041175525, 6.700000000000000178 ) ) ;
#11221=VECTOR ( 'NONE', #5160, 1000.000000000000000 ) ;
#11226=CARTESIAN_POINT ( 'NONE',  ( -27.07867591359219972, -26.64985754041175525, 6.800000000000000711 ) ) ;
#11230=ORIENTED_EDGE ( 'NONE', *, *, #8115, .F. ) ;
#11231=DIRECTION ( 'NONE',  ( 1.000000000000000000, -0.000000000000000000, 0.000000000000000000 ) ) ;
#11236=CYLINDRICAL_SURFACE ( 'NONE', #24131, 0.1000000000000028644 ) ;
#11241=ORIENTED_EDGE ( 'NONE', *, *, #5011, .F. ) ;
#11252=LINE ( 'NONE', #20736, #20978 ) ;
#11257=ORIENTED_EDGE ( 'NONE', *, *, #39213, .T. ) ;
#11268=ORIENTED_EDGE ( 'NONE', *, *, #6491, .F. ) ;
#11270=EDGE_CURVE ( 'NONE', #24116, #30761, #5472, .T. ) ;
#11278=ORIENTED_EDGE ( 'NONE', *, *, #27568, .F. ) ;
#11287=VECTOR ( 'NONE', #10347, 1000.000000000000000 ) ;
#11288=ORIENTED_EDGE ( 'NONE', *, *, #1148, .T. ) ;
#11292=DIRECTION ( 'NONE',  ( -0.000000000000000000, -0.000000000000000000, 1.000000000000000000 ) ) ;
#11293=ORIENTED_EDGE ( 'NONE', *, *, #5581, .T. ) ;
#11299=ADVANCED_FACE ( 'NONE', ( #11826 ), #24409, .F. ) ;
#11302=PLANE ( 'NONE',  #3590 ) ;
#11304=CARTESIAN_POINT ( 'NONE',  ( -6.348748702180634140, -26.64985754041175525, 6.800000000000000711 ) ) ;
#11308=ORIENTED_EDGE ( 'NONE', *, *, #15419, .F. ) ;
#11309=CARTESIAN_POINT ( 'NONE',  ( -8.348748702180635917, -25.49307895267003587, 6.700000000000000178 ) ) ;
#11311=DIRECTION ( 'NONE',  ( 0.000000000000000000, -0.000000000000000000, 1.000000000000000000 ) ) ;
#11318=EDGE_CURVE ( 'NONE', #33929, #37233, #27692, .T. ) ;
#11326=PLANE ( 'NONE',  #3658 ) ;
#11332=ORIENTED_EDGE ( 'NONE', *, *, #40292, .F. ) ;
#11338=VERTEX_POINT ( 'NONE', #19460 ) ;
#11340=DIRECTION ( 'NONE',  ( 1.000000000000000000, 0.000000000000000000, 0.000000000000000000 ) ) ;
#11345=CARTESIAN_POINT ( 'NONE',  ( -12.24874870218063627, -26.64985754041175525, 6.800000000000000711 ) ) ;
#11351=FACE_OUTER_BOUND ( 'NONE', #656, .T. ) ;
#11358=ORIENTED_EDGE ( 'NONE', *, *, #19977, .T. ) ;
#11359=EDGE_LOOP ( 'NONE', ( #2070, #33150, #28746, #36826 ) ) ;
#11367=LINE ( 'NONE', #17957, #23381 ) ;
#11374=ORIENTED_EDGE ( 'NONE', *, *, #19392, .T. ) ;
#11376=DIRECTION ( 'NONE',  ( 1.000000000000000000, 0.000000000000000000, 0.000000000000000000 ) ) ;
#11384=LINE ( 'NONE', #23564, #22428 ) ;
#11388=AXIS2_PLACEMENT_3D ( 'NONE', #9784, #10388, #35724 ) ;
#11391=DIRECTION ( 'NONE',  ( -0.000000000000000000, -0.000000000000000000, 1.000000000000000000 ) ) ;
#11393=ORIENTED_EDGE ( 'NONE', *, *, #39302, .F. ) ;
#11398=DIRECTION ( 'NONE',  ( 1.000000000000000000, 0.000000000000000000, 0.000000000000000000 ) ) ;
#11399=CARTESIAN_POINT ( 'NONE',  ( -25.07867591359219617, -26.64985754041175525, 6.700000000000000178 ) ) ;
#11407=LINE ( 'NONE', #8734, #10038 ) ;
#11408=ADVANCED_FACE ( 'NONE', ( #30141 ), #32430, .F. ) ;
#11416=CIRCLE ( 'NONE', #12069, 0.1000000000000028644 ) ;
#11417=AXIS2_PLACEMENT_3D ( 'NONE', #23282, #16675, #22887 ) ;
#11418=EDGE_CURVE ( 'NONE', #34241, #6781, #4628, .T. ) ;
#11424=DIRECTION ( 'NONE',  ( -0.000000000000000000, -0.000000000000000000, 1.000000000000000000 ) ) ;
#11426=CIRCLE ( 'NONE', #39027, 0.1000000000000028644 ) ;
#11429=DIRECTION ( 'NONE',  ( -0.000000000000000000, -0.000000000000000000, 1.000000000000000000 ) ) ;
#11430=CIRCLE ( 'NONE', #7512, 0.1000000000000028644 ) ;
#11440=LINE ( 'NONE', #2640, #21991 ) ;
#11441=ORIENTED_EDGE ( 'NONE', *, *, #4528, .T. ) ;
#11456=DIRECTION ( 'NONE',  ( -1.000000000000000000, 0.000000000000000000, 0.000000000000000000 ) ) ;
#11457=LINE ( 'NONE', #20950, #22504 ) ;
#11458=CARTESIAN_POINT ( 'NONE',  ( -38.34874870218063592, -25.49307895267003587, 6.700000000000000178 ) ) ;
#11461=DIRECTION ( 'NONE',  ( 0.000000000000000000, 0.000000000000000000, 1.000000000000000000 ) ) ;
#11471=ORIENTED_EDGE ( 'NONE', *, *, #16119, .F. ) ;
#11481=VECTOR ( 'NONE', #38736, 1000.000000000000000 ) ;
#11488=ORIENTED_EDGE ( 'NONE', *, *, #29842, .F. ) ;
#11493=DIRECTION ( 'NONE',  ( 1.000000000000000000, 0.000000000000000000, 0.000000000000000000 ) ) ;
#11495=DIRECTION ( 'NONE',  ( -0.000000000000000000, -0.000000000000000000, 1.000000000000000000 ) ) ;
#11501=VERTEX_POINT ( 'NONE', #38788 ) ;
#11507=AXIS2_PLACEMENT_3D ( 'NONE', #38686, #29438, #4135 ) ;
#11510=FACE_OUTER_BOUND ( 'NONE', #30644, .T. ) ;
#11512=CARTESIAN_POINT ( 'NONE',  ( -5.078675913592192614, -24.55319635012989110, 6.700000000000000178 ) ) ;
#11517=CARTESIAN_POINT ( 'NONE',  ( -51.01549048184568846, -38.28842912540938670, 6.800000000000000711 ) ) ;
#11518=EDGE_CURVE ( 'NONE', #32758, #25288, #10416, .T. ) ;
#11537=ADVANCED_FACE ( 'NONE', ( #26845 ), #26049, .F. ) ;
#11539=VECTOR ( 'NONE', #8035, 1000.000000000000000 ) ;
#11544=CYLINDRICAL_SURFACE ( 'NONE', #6406, 0.1000000000000028644 ) ;
#11546=DIRECTION ( 'NONE',  ( 0.000000000000000000, 0.000000000000000000, -1.000000000000000000 ) ) ;
#11547=CARTESIAN_POINT ( 'NONE',  ( -13.07867591359219617, -24.55319635012989110, 6.700000000000000178 ) ) ;
#11548=VERTEX_POINT ( 'NONE', #4433 ) ;
#11554=EDGE_LOOP ( 'NONE', ( #3609, #34169, #25102, #4622 ) ) ;
#11569=CARTESIAN_POINT ( 'NONE',  ( -14.87867591359218977, -26.64985754041175525, 6.700000000000000178 ) ) ;
#11581=DIRECTION ( 'NONE',  ( 1.000000000000000000, 0.000000000000000000, -0.000000000000000000 ) ) ;
#11584=CARTESIAN_POINT ( 'NONE',  ( -20.87867591359218622, -26.64985754041175525, 6.800000000000000711 ) ) ;
#11585=DIRECTION ( 'NONE',  ( 0.000000000000000000, 0.000000000000000000, 1.000000000000000000 ) ) ;
#11593=DIRECTION ( 'NONE',  ( 0.000000000000000000, 0.000000000000000000, 1.000000000000000000 ) ) ;
#11597=AXIS2_PLACEMENT_3D ( 'NONE', #710, #22130, #28701 ) ;
#11605=CARTESIAN_POINT ( 'NONE',  ( 3.651251297819360531, -25.49307895267003587, 6.700000000000000178 ) ) ;
#11611=DIRECTION ( 'NONE',  ( -0.000000000000000000, -0.000000000000000000, 1.000000000000000000 ) ) ;
#11619=CARTESIAN_POINT ( 'NONE',  ( -34.97867591359219830, -26.64985754041175525, 6.700000000000000178 ) ) ;
#11620=CARTESIAN_POINT ( 'NONE',  ( -38.87867591359218977, -24.55319635012989110, 6.700000000000000178 ) ) ;
#11624=CYLINDRICAL_SURFACE ( 'NONE', #5661, 0.1000000000000028644 ) ;
#11627=AXIS2_PLACEMENT_3D ( 'NONE', #32231, #9777, #13070 ) ;
#11632=LINE ( 'NONE', #11226, #10231 ) ;
#11633=ORIENTED_EDGE ( 'NONE', *, *, #9799, .F. ) ;
#11637=DIRECTION ( 'NONE',  ( -0.000000000000000000, -0.000000000000000000, 1.000000000000000000 ) ) ;
#11643=DIRECTION ( 'NONE',  ( 1.000000000000000000, 0.000000000000000000, 0.000000000000000000 ) ) ;
#11646=ORIENTED_EDGE ( 'NONE', *, *, #38389, .F. ) ;
#11652=AXIS2_PLACEMENT_3D ( 'NONE', #5943, #24047, #15196 ) ;
#11661=CARTESIAN_POINT ( 'NONE',  ( -3.078675913592197944, -26.64985754041175525, 6.700000000000000178 ) ) ;
#11663=PLANE ( 'NONE',  #30087 ) ;
#11667=DIRECTION ( 'NONE',  ( -0.000000000000000000, -0.000000000000000000, 1.000000000000000000 ) ) ;
#11676=DIRECTION ( 'NONE',  ( 0.000000000000000000, 0.000000000000000000, -1.000000000000000000 ) ) ;
#11681=CARTESIAN_POINT ( 'NONE',  ( -38.44874870218063734, -26.64985754041175525, 6.700000000000000178 ) ) ;
#11683=DIRECTION ( 'NONE',  ( 0.000000000000000000, 0.000000000000000000, 1.000000000000000000 ) ) ;
#11691=FACE_OUTER_BOUND ( 'NONE', #24503, .T. ) ;
#11696=EDGE_CURVE ( 'NONE', #8305, #8931, #34069, .T. ) ;
#11699=EDGE_LOOP ( 'NONE', ( #38003, #30411, #28425, #32795 ) ) ;
#11707=ORIENTED_EDGE ( 'NONE', *, *, #29977, .T. ) ;
#11717=DIRECTION ( 'NONE',  ( 1.000000000000000000, 0.000000000000000000, 0.000000000000000000 ) ) ;
#11718=VECTOR ( 'NONE', #3646, 1000.000000000000000 ) ;
#11720=CARTESIAN_POINT ( 'NONE',  ( -53.21549048184568420, -30.38627270959228710, 6.000000000000000000 ) ) ;
#11727=DIRECTION ( 'NONE',  ( 1.000000000000000000, 0.000000000000000000, 0.000000000000000000 ) ) ;
#11729=CIRCLE ( 'NONE', #14350, 0.1000000000000028644 ) ;
#11735=ORIENTED_EDGE ( 'NONE', *, *, #3492, .T. ) ;
#11748=ORIENTED_EDGE ( 'NONE', *, *, #40236, .T. ) ;
#11749=FACE_OUTER_BOUND ( 'NONE', #2735, .T. ) ;
#11751=ORIENTED_EDGE ( 'NONE', *, *, #13383, .F. ) ;
#11756=ORIENTED_EDGE ( 'NONE', *, *, #31072, .T. ) ;
#11759=DIRECTION ( 'NONE',  ( 1.000000000000000000, 0.000000000000000000, 0.000000000000000000 ) ) ;
#11770=DIRECTION ( 'NONE',  ( 1.000000000000000000, 0.000000000000000000, 0.000000000000000000 ) ) ;
#11782=DIRECTION ( 'NONE',  ( 0.000000000000000000, 0.000000000000000000, 1.000000000000000000 ) ) ;
#11786=EDGE_CURVE ( 'NONE', #14653, #33732, #13279, .T. ) ;
#11792=ORIENTED_EDGE ( 'NONE', *, *, #28704, .T. ) ;
#11793=CARTESIAN_POINT ( 'NONE',  ( -37.07867591359219261, -26.64985754041175525, 6.700000000000000178 ) ) ;
#11795=EDGE_CURVE ( 'NONE', #1142, #28508, #15716, .T. ) ;
#11797=DIRECTION ( 'NONE',  ( 0.000000000000000000, 0.000000000000000000, -1.000000000000000000 ) ) ;
#11799=SHAPE_DEFINITION_REPRESENTATION ( #19319, #39533 ) ;
#11815=DIRECTION ( 'NONE',  ( 0.000000000000000000, 1.000000000000000000, 0.000000000000000000 ) ) ;
#11818=ORIENTED_EDGE ( 'NONE', *, *, #22804, .T. ) ;
#11821=LINE ( 'NONE', #15337, #7042 ) ;
#11826=FACE_OUTER_BOUND ( 'NONE', #16483, .T. ) ;
#11828=CARTESIAN_POINT ( 'NONE',  ( -54.01549048184568846, -38.28842912540938670, -4.152976064860135708 ) ) ;
#11833=CARTESIAN_POINT ( 'NONE',  ( -4.448748702180642667, -26.64985754041175525, 6.700000000000000178 ) ) ;
#11834=EDGE_CURVE ( 'NONE', #24757, #8717, #9585, .T. ) ;
#11836=DIRECTION ( 'NONE',  ( -0.000000000000000000, -1.000000000000000000, -0.000000000000000000 ) ) ;
#11837=CARTESIAN_POINT ( 'NONE',  ( -20.97867591359219475, -26.64985754041175525, 6.700000000000000178 ) ) ;
#11839=ORIENTED_EDGE ( 'NONE', *, *, #2406, .F. ) ;
#11841=VERTEX_POINT ( 'NONE', #16170 ) ;
#11847=VECTOR ( 'NONE', #27802, 1000.000000000000000 ) ;
#11848=EDGE_CURVE ( 'NONE', #35180, #11501, #28940, .T. ) ;
#11853=CARTESIAN_POINT ( 'NONE',  ( -31.07867591359219617, -26.64985754041175525, 6.700000000000000178 ) ) ;
#11855=ORIENTED_EDGE ( 'NONE', *, *, #10863, .F. ) ;
#11867=DIRECTION ( 'NONE',  ( 0.000000000000000000, 1.000000000000000000, 0.000000000000000000 ) ) ;
#11869=ORIENTED_EDGE ( 'NONE', *, *, #20208, .F. ) ;
#11870=CARTESIAN_POINT ( 'NONE',  ( -51.01549048184568846, -30.38627270959228710, 6.800000000000000711 ) ) ;
#11891=DIRECTION ( 'NONE',  ( 0.000000000000000000, 0.000000000000000000, 1.000000000000000000 ) ) ;
#11898=LINE ( 'NONE', #33974, #5717 ) ;
#11901=CARTESIAN_POINT ( 'NONE',  ( -4.878675913592187108, -26.64985754041175525, 6.700000000000000178 ) ) ;
#11904=ORIENTED_EDGE ( 'NONE', *, *, #9368, .T. ) ;
#11905=CARTESIAN_POINT ( 'NONE',  ( -8.878675913592189772, -24.55319635012989110, 6.700000000000000178 ) ) ;
#11907=DIRECTION ( 'NONE',  ( 0.000000000000000000, 0.000000000000000000, 1.000000000000000000 ) ) ;
#11908=VERTEX_POINT ( 'NONE', #22570 ) ;
#11914=EDGE_CURVE ( 'NONE', #160, #38778, #32437, .T. ) ;
#11916=ORIENTED_EDGE ( 'NONE', *, *, #27061, .T. ) ;
#11925=DIRECTION ( 'NONE',  ( 0.000000000000000000, 0.000000000000000000, 1.000000000000000000 ) ) ;
#11931=LINE ( 'NONE', #37059, #13566 ) ;
#11932=EDGE_CURVE ( 'NONE', #32407, #25870, #7307, .T. ) ;
#11936=CARTESIAN_POINT ( 'NONE',  ( 3.121324086407806231, -26.64985754041175525, 6.800000000000000711 ) ) ;
#11943=DIRECTION ( 'NONE',  ( -0.000000000000000000, -0.000000000000000000, 1.000000000000000000 ) ) ;
#11953=CARTESIAN_POINT ( 'NONE',  ( -38.97867591359219119, -26.64985754041175525, 6.700000000000000178 ) ) ;
#11956=DIRECTION ( 'NONE',  ( 1.000000000000000000, 0.000000000000000000, -0.000000000000000000 ) ) ;
#11963=ORIENTED_EDGE ( 'NONE', *, *, #34569, .F. ) ;
#11971=VECTOR ( 'NONE', #37939, 1000.000000000000000 ) ;
#11985=FACE_OUTER_BOUND ( 'NONE', #39100, .T. ) ;
#11994=DIRECTION ( 'NONE',  ( 0.000000000000000000, 1.000000000000000000, 0.000000000000000000 ) ) ;
#12008=CARTESIAN_POINT ( 'NONE',  ( -13.07867591359219617, -26.64985754041175525, 6.700000000000000178 ) ) ;
#12014=DIRECTION ( 'NONE',  ( 0.000000000000000000, 0.000000000000000000, 1.000000000000000000 ) ) ;
#12018=CARTESIAN_POINT ( 'NONE',  ( -7.078675913592194391, -24.55319635012989110, 6.800000000000000711 ) ) ;
#12037=PLANE ( 'NONE',  #34551 ) ;
#12039=AXIS2_PLACEMENT_3D ( 'NONE', #33460, #14073, #8294 ) ;
#12047=VECTOR ( 'NONE', #8516, 1000.000000000000000 ) ;
#12048=DIRECTION ( 'NONE',  ( -0.000000000000000000, -0.000000000000000000, 1.000000000000000000 ) ) ;
#12054=FACE_OUTER_BOUND ( 'NONE', #32062, .T. ) ;
#12058=DIRECTION ( 'NONE',  ( 1.000000000000000000, 0.000000000000000000, -0.000000000000000000 ) ) ;
#12066=VERTEX_POINT ( 'NONE', #36874 ) ;
#12068=EDGE_CURVE ( 'NONE', #7879, #21734, #28856, .T. ) ;
#12069=AXIS2_PLACEMENT_3D ( 'NONE', #33756, #40310, #5945 ) ;
#12071=VECTOR ( 'NONE', #4948, 1000.000000000000000 ) ;
#12073=CARTESIAN_POINT ( 'NONE',  ( -26.34874870218063947, -26.64985754041175525, 6.700000000000000178 ) ) ;
#12080=AXIS2_PLACEMENT_3D ( 'NONE', #15729, #28281, #6264 ) ;
#12092=CARTESIAN_POINT ( 'NONE',  ( -26.97867591359219475, -26.64985754041175525, 6.700000000000000178 ) ) ;
#12094=CARTESIAN_POINT ( 'NONE',  ( -28.34874870218063947, -25.49307895267003587, 6.800000000000000711 ) ) ;
#12095=PLANE ( 'NONE',  #19602 ) ;
#12105=CARTESIAN_POINT ( 'NONE',  ( -2.878675913592191993, -26.64985754041175525, 6.700000000000000178 ) ) ;
#12110=ORIENTED_EDGE ( 'NONE', *, *, #16718, .T. ) ;
#12114=ADVANCED_FACE ( 'NONE', ( #30503 ), #1908, .F. ) ;
#12122=CARTESIAN_POINT ( 'NONE',  ( -15.07867591359219439, -26.64985754041175525, 6.800000000000000711 ) ) ;
#12123=ORIENTED_EDGE ( 'NONE', *, *, #36221, .F. ) ;
#12124=DIRECTION ( 'NONE',  ( 0.000000000000000000, 0.000000000000000000, 1.000000000000000000 ) ) ;
#12129=EDGE_CURVE ( 'NONE', #8931, #7569, #23163, .T. ) ;
#12144=EDGE_LOOP ( 'NONE', ( #30053, #34620, #27704, #23254 ) ) ;
#12150=EDGE_LOOP ( 'NONE', ( #1013, #21347, #12642, #7209 ) ) ;
#12153=CARTESIAN_POINT ( 'NONE',  ( 3.651251297819360531, -26.64985754041175525, 6.700000000000000178 ) ) ;
#12154=DIRECTION ( 'NONE',  ( 0.000000000000000000, 0.000000000000000000, 1.000000000000000000 ) ) ;
#12155=ORIENTED_EDGE ( 'NONE', *, *, #19678, .T. ) ;
#12162=CIRCLE ( 'NONE', #31269, 0.1000000000000028644 ) ;
#12164=AXIS2_PLACEMENT_3D ( 'NONE', #14791, #2485, #1865 ) ;
#12168=DIRECTION ( 'NONE',  ( -0.000000000000000000, -1.000000000000000000, -0.000000000000000000 ) ) ;
#12170=ORIENTED_EDGE ( 'NONE', *, *, #3489, .T. ) ;
#12175=EDGE_CURVE ( 'NONE', #9750, #17561, #37392, .T. ) ;
#12180=ORIENTED_EDGE ( 'NONE', *, *, #4839, .T. ) ;
#12197=CARTESIAN_POINT ( 'NONE',  ( 1.751251297819361730, -26.64985754041175525, 6.800000000000000711 ) ) ;
#12201=VERTEX_POINT ( 'NONE', #9069 ) ;
#12204=VECTOR ( 'NONE', #22828, 1000.000000000000000 ) ;
#12207=DIRECTION ( 'NONE',  ( 0.000000000000000000, 0.000000000000000000, -1.000000000000000000 ) ) ;
#12209=CARTESIAN_POINT ( 'NONE',  ( -20.44874870218064444, -26.64985754041175525, 6.700000000000000178 ) ) ;
#12211=LINE ( 'NONE', #25999, #11481 ) ;
#12214=DIRECTION ( 'NONE',  ( -0.000000000000000000, -0.000000000000000000, 1.000000000000000000 ) ) ;
#12217=CARTESIAN_POINT ( 'NONE',  ( -30.97867591359219119, -26.64985754041175525, 6.700000000000000178 ) ) ;
#12218=EDGE_LOOP ( 'NONE', ( #11748, #13280, #26442, #38304 ) ) ;
#12221=ORIENTED_EDGE ( 'NONE', *, *, #39276, .F. ) ;
#12227=ORIENTED_EDGE ( 'NONE', *, *, #26487, .T. ) ;
#12232=CIRCLE ( 'NONE', #6980, 0.1000000000000028644 ) ;
#12234=ORIENTED_EDGE ( 'NONE', *, *, #19771, .T. ) ;
#12239=VECTOR ( 'NONE', #33446, 1000.000000000000000 ) ;
#12240=FACE_OUTER_BOUND ( 'NONE', #5495, .T. ) ;
#12255=DIRECTION ( 'NONE',  ( 0.000000000000000000, 0.000000000000000000, 1.000000000000000000 ) ) ;
#12256=CARTESIAN_POINT ( 'NONE',  ( -22.44874870218064089, -26.64985754041175525, 6.700000000000000178 ) ) ;
#12261=EDGE_LOOP ( 'NONE', ( #16256, #37034, #20679, #24149 ) ) ;
#12267=PLANE ( 'NONE',  #17441 ) ;
#12275=CARTESIAN_POINT ( 'NONE',  ( -33.07867591359219972, -24.55319635012989110, 6.700000000000000178 ) ) ;
#12276=UNCERTAINTY_MEASURE_WITH_UNIT (LENGTH_MEASURE( 1.000000000000000082E-05 ), #15675, 'distance_accuracy_value', 'NONE');
#12282=DIRECTION ( 'NONE',  ( 1.000000000000000000, 0.000000000000000000, 0.000000000000000000 ) ) ;
#12288=DIRECTION ( 'NONE',  ( -0.000000000000000000, -0.000000000000000000, 1.000000000000000000 ) ) ;
#12294=ORIENTED_EDGE ( 'NONE', *, *, #23161, .F. ) ;
#12295=FACE_OUTER_BOUND ( 'NONE', #20875, .T. ) ;
#12302=DIRECTION ( 'NONE',  ( 1.000000000000000000, 0.000000000000000000, 0.000000000000000000 ) ) ;
#12303=ORIENTED_EDGE ( 'NONE', *, *, #12933, .T. ) ;
#12310=DIRECTION ( 'NONE',  ( 1.000000000000000000, 0.000000000000000000, -0.000000000000000000 ) ) ;
#12312=ORIENTED_EDGE ( 'NONE', *, *, #27516, .T. ) ;
#12316=ORIENTED_EDGE ( 'NONE', *, *, #8302, .T. ) ;
#12329=EDGE_CURVE ( 'NONE', #2870, #37024, #33029, .T. ) ;
#12331=DIRECTION ( 'NONE',  ( -0.000000000000000000, -0.000000000000000000, 1.000000000000000000 ) ) ;
#12332=VERTEX_POINT ( 'NONE', #4819 ) ;
#12335=VERTEX_POINT ( 'NONE', #29926 ) ;
#12338=AXIS2_PLACEMENT_3D ( 'NONE', #24191, #5257, #33065 ) ;
#12352=DIRECTION ( 'NONE',  ( -0.000000000000000000, -0.000000000000000000, 1.000000000000000000 ) ) ;
#12355=ORIENTED_EDGE ( 'NONE', *, *, #35636, .F. ) ;
#12367=ORIENTED_EDGE ( 'NONE', *, *, #32984, .F. ) ;
#12371=ORIENTED_EDGE ( 'NONE', *, *, #23183, .F. ) ;
#12381=LINE ( 'NONE', #24323, #38446 ) ;
#12383=DIRECTION ( 'NONE',  ( -0.000000000000000000, -0.000000000000000000, 1.000000000000000000 ) ) ;
#12384=PLANE ( 'NONE',  #27146 ) ;
#12388=VECTOR ( 'NONE', #8292, 1000.000000000000000 ) ;
#12393=APPLICATION_CONTEXT ( 'automotive_design' ) ;
#12395=CARTESIAN_POINT ( 'NONE',  ( -22.97867591359219119, -24.55319635012989110, 6.800000000000000711 ) ) ;
#12411=DIRECTION ( 'NONE',  ( 1.000000000000000000, 0.000000000000000000, 0.000000000000000000 ) ) ;
#12416=LINE ( 'NONE', #34472, #36476 ) ;
#12419=CARTESIAN_POINT ( 'NONE',  ( -14.87867591359218977, -26.64985754041175525, 6.700000000000000178 ) ) ;
#12422=EDGE_CURVE ( 'NONE', #3833, #26349, #26609, .T. ) ;
#12425=CARTESIAN_POINT ( 'NONE',  ( -24.44874870218064089, -26.64985754041175525, 6.700000000000000178 ) ) ;
#12428=ORIENTED_EDGE ( 'NONE', *, *, #32159, .F. ) ;
#12437=ORIENTED_EDGE ( 'NONE', *, *, #17829, .T. ) ;
#12439=DIRECTION ( 'NONE',  ( 1.000000000000000000, 0.000000000000000000, 0.000000000000000000 ) ) ;
#12441=ORIENTED_EDGE ( 'NONE', *, *, #2886, .T. ) ;
#12444=CARTESIAN_POINT ( 'NONE',  ( -34.24874870218063450, -25.49307895267003587, 6.700000000000000178 ) ) ;
#12456=ORIENTED_EDGE ( 'NONE', *, *, #33575, .T. ) ;
#12462=CARTESIAN_POINT ( 'NONE',  ( -0.8786759135921904385, -24.55319635012989110, 6.700000000000000178 ) ) ;
#12464=DIRECTION ( 'NONE',  ( 1.000000000000000000, 0.000000000000000000, 0.000000000000000000 ) ) ;
#12468=EDGE_CURVE ( 'NONE', #13597, #33127, #24155, .T. ) ;
#12472=EDGE_CURVE ( 'NONE', #10309, #13597, #324, .T. ) ;
#12474=ORIENTED_EDGE ( 'NONE', *, *, #32427, .T. ) ;
#12481=FACE_OUTER_BOUND ( 'NONE', #28647, .T. ) ;
#12489=ORIENTED_EDGE ( 'NONE', *, *, #19307, .T. ) ;
#12490=VECTOR ( 'NONE', #13254, 1000.000000000000000 ) ;
#12491=ORIENTED_EDGE ( 'NONE', *, *, #25453, .F. ) ;
#12505=DIRECTION ( 'NONE',  ( 0.000000000000000000, 0.000000000000000000, 1.000000000000000000 ) ) ;
#12515=EDGE_CURVE ( 'NONE', #38606, #5089, #22516, .T. ) ;
#12516=DIRECTION ( 'NONE',  ( -0.000000000000000000, -1.000000000000000000, -0.000000000000000000 ) ) ;
#12536=ADVANCED_FACE ( 'NONE', ( #28263 ), #13025, .F. ) ;
#12548=ORIENTED_EDGE ( 'NONE', *, *, #38740, .F. ) ;
#12557=ORIENTED_EDGE ( 'NONE', *, *, #23536, .F. ) ;
#12567=DIRECTION ( 'NONE',  ( -0.000000000000000000, -0.000000000000000000, 1.000000000000000000 ) ) ;
#12571=ORIENTED_EDGE ( 'NONE', *, *, #19360, .F. ) ;
#12573=CARTESIAN_POINT ( 'NONE',  ( -20.34874870218063947, -25.49307895267003587, 6.800000000000000711 ) ) ;
#12582=FACE_BOUND ( 'NONE', #15518, .T. ) ;
#12598=ORIENTED_EDGE ( 'NONE', *, *, #36526, .T. ) ;
#12599=ORIENTED_EDGE ( 'NONE', *, *, #20409, .F. ) ;
#12601=LINE ( 'NONE', #15894, #30655 ) ;
#12602=VECTOR ( 'NONE', #37253, 1000.000000000000000 ) ;
#12611=CARTESIAN_POINT ( 'NONE',  ( -25.07867591359219617, -26.64985754041175525, 6.700000000000000178 ) ) ;
#12613=DIRECTION ( 'NONE',  ( 1.000000000000000000, 0.000000000000000000, 0.000000000000000000 ) ) ;
#12615=ADVANCED_FACE ( 'NONE', ( #25590 ), #15299, .F. ) ;
#12617=CARTESIAN_POINT ( 'NONE',  ( 6.921324086407803833, -26.64985754041175525, 6.700000000000000178 ) ) ;
#12624=FACE_OUTER_BOUND ( 'NONE', #9666, .T. ) ;
#12626=DIRECTION ( 'NONE',  ( 1.000000000000000000, 0.000000000000000000, -0.000000000000000000 ) ) ;
#12630=EDGE_CURVE ( 'NONE', #6110, #8281, #12416, .T. ) ;
#12631=LINE ( 'NONE', #25201, #13416 ) ;
#12637=EDGE_LOOP ( 'NONE', ( #30860, #1977, #32030, #16234 ) ) ;
#12640=VERTEX_POINT ( 'NONE', #18795 ) ;
#12641=EDGE_CURVE ( 'NONE', #30400, #18363, #31369, .T. ) ;
#12642=ORIENTED_EDGE ( 'NONE', *, *, #13323, .F. ) ;
#12648=ADVANCED_FACE ( 'NONE', ( #7852 ), #35677, .T. ) ;
#12666=CARTESIAN_POINT ( 'NONE',  ( -42.83131703149249603, -32.06993018339340296, 6.800000000000000711 ) ) ;
#12675=EDGE_CURVE ( 'NONE', #17561, #2391, #1298, .T. ) ;
#12683=EDGE_CURVE ( 'NONE', #39450, #32407, #35823, .T. ) ;
#12686=DIRECTION ( 'NONE',  ( -0.000000000000000000, 0.000000000000000000, 1.000000000000000000 ) ) ;
#12688=EDGE_LOOP ( 'NONE', ( #14952, #14458, #32153, #8188 ) ) ;
#12692=VECTOR ( 'NONE', #37963, 1000.000000000000000 ) ;
#12699=DIRECTION ( 'NONE',  ( -0.000000000000000000, -1.000000000000000000, -0.000000000000000000 ) ) ;
#12703=VERTEX_POINT ( 'NONE', #13228 ) ;
#12705=VERTEX_POINT ( 'NONE', #32789 ) ;
#12706=CARTESIAN_POINT ( 'NONE',  ( 7.021324086407807030, -26.64985754041175525, 6.700000000000000178 ) ) ;
#12709=DIRECTION ( 'NONE',  ( -0.000000000000000000, -0.000000000000000000, 1.000000000000000000 ) ) ;
#12717=AXIS2_PLACEMENT_3D ( 'NONE', #15588, #34153, #28141 ) ;
#12725=EDGE_LOOP ( 'NONE', ( #2810, #29199, #5005, #32306 ) ) ;
#12729=ORIENTED_EDGE ( 'NONE', *, *, #9428, .T. ) ;
#12742=EDGE_CURVE ( 'NONE', #25329, #38606, #14771, .T. ) ;
#12743=VECTOR ( 'NONE', #24799, 1000.000000000000000 ) ;
#12752=ORIENTED_EDGE ( 'NONE', *, *, #39407, .T. ) ;
#12762=VECTOR ( 'NONE', #32424, 1000.000000000000000 ) ;
#12765=CARTESIAN_POINT ( 'NONE',  ( -36.87867591359218977, -26.64985754041175525, 6.700000000000000178 ) ) ;
#12771=CARTESIAN_POINT ( 'NONE',  ( 1.021324086407808585, -26.64985754041175525, 6.700000000000000178 ) ) ;
#12773=VECTOR ( 'NONE', #10311, 1000.000000000000000 ) ;
#12778=ORIENTED_EDGE ( 'NONE', *, *, #9592, .F. ) ;
#12783=FACE_OUTER_BOUND ( 'NONE', #14182, .T. ) ;
#12795=CARTESIAN_POINT ( 'NONE',  ( -37.07867591359219261, -26.64985754041175525, 6.700000000000000178 ) ) ;
#12801=ORIENTED_EDGE ( 'NONE', *, *, #16275, .T. ) ;
#12802=VECTOR ( 'NONE', #15785, 1000.000000000000000 ) ;
#12803=DIRECTION ( 'NONE',  ( -0.000000000000000000, -1.000000000000000000, -0.000000000000000000 ) ) ;
#12809=CARTESIAN_POINT ( 'NONE',  ( -5.078675913592192614, -26.64985754041175525, 6.700000000000000178 ) ) ;
#12812=DIRECTION ( 'NONE',  ( 0.000000000000000000, 0.000000000000000000, 1.000000000000000000 ) ) ;
#12816=DIRECTION ( 'NONE',  ( 1.000000000000000000, -0.000000000000000000, 0.000000000000000000 ) ) ;
#12819=LINE ( 'NONE', #22318, #39771 ) ;
#12820=EDGE_CURVE ( 'NONE', #301, #10798, #8838, .T. ) ;
#12821=LINE ( 'NONE', #6463, #25449 ) ;
#12823=CARTESIAN_POINT ( 'NONE',  ( 3.021324086407803478, -24.55319635012989110, 6.800000000000000711 ) ) ;
#12824=AXIS2_PLACEMENT_3D ( 'NONE', #37614, #24247, #12302 ) ;
#12826=VERTEX_POINT ( 'NONE', #13633 ) ;
#12831=AXIS2_PLACEMENT_3D ( 'NONE', #17177, #17994, #33674 ) ;
#12833=ORIENTED_EDGE ( 'NONE', *, *, #351, .F. ) ;
#12834=LINE ( 'NONE', #31788, #16684 ) ;
#12835=CARTESIAN_POINT ( 'NONE',  ( -12.97867591359219297, -26.64985754041175525, 6.800000000000000711 ) ) ;
#12840=ORIENTED_EDGE ( 'NONE', *, *, #33683, .T. ) ;
#12842=PLANE ( 'NONE',  #13592 ) ;
#12843=VERTEX_POINT ( 'NONE', #14829 ) ;
#12845=EDGE_CURVE ( 'NONE', #16562, #6115, #39958, .T. ) ;
#12846=ORIENTED_EDGE ( 'NONE', *, *, #407, .F. ) ;
#12853=VECTOR ( 'NONE', #13550, 1000.000000000000000 ) ;
#12861=CARTESIAN_POINT ( 'NONE',  ( -11.07867591359219794, -26.64985754041175525, 6.800000000000000711 ) ) ;
#12865=ORIENTED_EDGE ( 'NONE', *, *, #23790, .F. ) ;
#12874=LINE ( 'NONE', #6712, #3332 ) ;
#12875=DIRECTION ( 'NONE',  ( -0.000000000000000000, -0.000000000000000000, 1.000000000000000000 ) ) ;
#12879=DIRECTION ( 'NONE',  ( -0.000000000000000000, -1.000000000000000000, -0.000000000000000000 ) ) ;
#12881=ADVANCED_FACE ( 'NONE', ( #40156 ), #27194, .F. ) ;
#12883=EDGE_CURVE ( 'NONE', #4585, #22121, #8043, .T. ) ;
#12886=CARTESIAN_POINT ( 'NONE',  ( -28.24874870218063805, -26.64985754041175525, 6.800000000000000711 ) ) ;
#12889=LINE ( 'NONE', #25256, #37913 ) ;
#12890=ORIENTED_EDGE ( 'NONE', *, *, #38711, .T. ) ;
#12893=CARTESIAN_POINT ( 'NONE',  ( 11.65737507970504439, -23.60493063168009442, 6.800000000000000711 ) ) ;
#12901=ORIENTED_EDGE ( 'NONE', *, *, #26104, .T. ) ;
#12918=DIRECTION ( 'NONE',  ( 0.000000000000000000, 0.000000000000000000, 1.000000000000000000 ) ) ;
#12921=LINE ( 'NONE', #25487, #34101 ) ;
#12922=VECTOR ( 'NONE', #37189, 1000.000000000000000 ) ;
#12925=VECTOR ( 'NONE', #1195, 1000.000000000000000 ) ;
#12927=ADVANCED_FACE ( 'NONE', ( #17499 ), #11326, .F. ) ;
#12930=FACE_OUTER_BOUND ( 'NONE', #5751, .T. ) ;
#12933=EDGE_CURVE ( 'NONE', #1854, #25414, #33404, .T. ) ;
#12941=ORIENTED_EDGE ( 'NONE', *, *, #13147, .T. ) ;
#12947=AXIS2_PLACEMENT_3D ( 'NONE', #32008, #38353, #12439 ) ;
#12954=CARTESIAN_POINT ( 'NONE',  ( -3.078675913592197944, -26.64985754041175525, 6.800000000000000711 ) ) ;
#12957=CARTESIAN_POINT ( 'NONE',  ( -32.24874870218063450, -25.49307895267003587, 6.700000000000000178 ) ) ;
#12961=ORIENTED_EDGE ( 'NONE', *, *, #31350, .T. ) ;
#12963=ORIENTED_EDGE ( 'NONE', *, *, #25818, .T. ) ;
#12978=ORIENTED_EDGE ( 'NONE', *, *, #4155, .T. ) ;
#12979=VECTOR ( 'NONE', #10743, 1000.000000000000000 ) ;
#12982=DIRECTION ( 'NONE',  ( 0.000000000000000000, 0.000000000000000000, 1.000000000000000000 ) ) ;
#12983=EDGE_CURVE ( 'NONE', #30200, #27310, #28007, .T. ) ;
#12986=ORIENTED_EDGE ( 'NONE', *, *, #3855, .T. ) ;
#12988=DIRECTION ( 'NONE',  ( 1.000000000000000000, 0.000000000000000000, 0.000000000000000000 ) ) ;
#12994=FACE_BOUND ( 'NONE', #28579, .T. ) ;
#12996=VERTEX_POINT ( 'NONE', #40550 ) ;
#12999=VECTOR ( 'NONE', #24457, 1000.000000000000000 ) ;
#13001=EDGE_LOOP ( 'NONE', ( #33023, #457, #9851, #28548 ) ) ;
#13011=VERTEX_POINT ( 'NONE', #31518 ) ;
#13013=DIRECTION ( 'NONE',  ( 1.000000000000000000, 0.000000000000000000, 0.000000000000000000 ) ) ;
#13023=LINE ( 'NONE', #18577, #5825 ) ;
#13025=PLANE ( 'NONE',  #27272 ) ;
#13027=VECTOR ( 'NONE', #31049, 1000.000000000000000 ) ;
#13034=FACE_OUTER_BOUND ( 'NONE', #37630, .T. ) ;
#13038=AXIS2_PLACEMENT_3D ( 'NONE', #35722, #1349, #36122 ) ;
#13039=ORIENTED_EDGE ( 'NONE', *, *, #29011, .T. ) ;
#13040=DIRECTION ( 'NONE',  ( 0.000000000000000000, 1.000000000000000000, 0.000000000000000000 ) ) ;
#13045=ORIENTED_EDGE ( 'NONE', *, *, #22748, .T. ) ;
#13046=CARTESIAN_POINT ( 'NONE',  ( -10.97867591359219475, -26.64985754041175525, 6.700000000000000178 ) ) ;
#13050=ORIENTED_EDGE ( 'NONE', *, *, #36358, .T. ) ;
#13070=DIRECTION ( 'NONE',  ( 1.000000000000000000, 0.000000000000000000, 0.000000000000000000 ) ) ;
#13072=CYLINDRICAL_SURFACE ( 'NONE', #5219, 0.1000000000000028644 ) ;
#13078=PLANE ( 'NONE',  #35195 ) ;
#13086=ORIENTED_EDGE ( 'NONE', *, *, #15951, .F. ) ;
#13096=VECTOR ( 'NONE', #38732, 1000.000000000000000 ) ;
#13097=EDGE_CURVE ( 'NONE', #15366, #18497, #33232, .T. ) ;
#13098=EDGE_LOOP ( 'NONE', ( #17647, #38272, #35398, #9823 ) ) ;
#13101=EDGE_LOOP ( 'NONE', ( #22190, #38287, #27299, #27416 ) ) ;
#13104=DIRECTION ( 'NONE',  ( 1.000000000000000000, 0.000000000000000000, 0.000000000000000000 ) ) ;
#13108=VERTEX_POINT ( 'NONE', #1046 ) ;
#13109=FACE_OUTER_BOUND ( 'NONE', #13001, .T. ) ;
#13111=CARTESIAN_POINT ( 'NONE',  ( -22.87867591359218977, -26.64985754041175525, 6.700000000000000178 ) ) ;
#13113=EDGE_CURVE ( 'NONE', #26273, #6408, #20155, .T. ) ;
#13116=ORIENTED_EDGE ( 'NONE', *, *, #36358, .F. ) ;
#13118=ADVANCED_FACE ( 'NONE', ( #26154 ), #840, .F. ) ;
#13119=PLANE ( 'NONE',  #6288 ) ;
#13128=DIRECTION ( 'NONE',  ( 1.000000000000000000, 0.000000000000000000, 0.000000000000000000 ) ) ;
#13133=DIRECTION ( 'NONE',  ( -0.000000000000000000, -0.000000000000000000, 1.000000000000000000 ) ) ;
#13137=ADVANCED_FACE ( 'NONE', ( #23063 ), #1445, .F. ) ;
#13143=LINE ( 'NONE', #16023, #13226 ) ;
#13145=ORIENTED_EDGE ( 'NONE', *, *, #34676, .T. ) ;
#13147=EDGE_CURVE ( 'NONE', #8480, #26273, #25743, .T. ) ;
#13148=VERTEX_POINT ( 'NONE', #1251 ) ;
#13154=ORIENTED_EDGE ( 'NONE', *, *, #13641, .F. ) ;
#13155=ORIENTED_EDGE ( 'NONE', *, *, #6289, .T. ) ;
#13157=AXIS2_PLACEMENT_3D ( 'NONE', #26543, #20153, #11676 ) ;
#13159=DIRECTION ( 'NONE',  ( 0.000000000000000000, 0.000000000000000000, 1.000000000000000000 ) ) ;
#13162=CARTESIAN_POINT ( 'NONE',  ( -14.44874870218064089, -25.49307895267003587, 6.700000000000000178 ) ) ;
#13183=VECTOR ( 'NONE', #37616, 1000.000000000000000 ) ;
#13184=DIRECTION ( 'NONE',  ( 1.000000000000000000, 0.000000000000000000, 0.000000000000000000 ) ) ;
#13187=ORIENTED_EDGE ( 'NONE', *, *, #29714, .T. ) ;
#13193=ORIENTED_EDGE ( 'NONE', *, *, #5823, .F. ) ;
#13194=AXIS2_PLACEMENT_3D ( 'NONE', #26053, #10780, #38981 ) ;
#13197=FACE_BOUND ( 'NONE', #17887, .T. ) ;
#13202=ORIENTED_EDGE ( 'NONE', *, *, #16229, .T. ) ;
#13203=ORIENTED_EDGE ( 'NONE', *, *, #10230, .T. ) ;
#13205=LINE ( 'NONE', #25773, #12773 ) ;
#13210=CARTESIAN_POINT ( 'NONE',  ( -2.448748702180640446, -26.64985754041175525, 6.700000000000000178 ) ) ;
#13224=DIRECTION ( 'NONE',  ( 0.000000000000000000, 1.000000000000000000, 0.000000000000000000 ) ) ;
#13226=VECTOR ( 'NONE', #37229, 1000.000000000000000 ) ;
#13228=CARTESIAN_POINT ( 'NONE',  ( -22.44874870218064089, -26.64985754041175525, 6.700000000000000178 ) ) ;
#13230=DIRECTION ( 'NONE',  ( 0.000000000000000000, 0.000000000000000000, 1.000000000000000000 ) ) ;
#13236=FACE_OUTER_BOUND ( 'NONE', #20851, .T. ) ;
#13245=VERTEX_POINT ( 'NONE', #7993 ) ;
#13250=CARTESIAN_POINT ( 'NONE',  ( -28.97867591359219475, -26.64985754041175525, 6.700000000000000178 ) ) ;
#13251=ORIENTED_EDGE ( 'NONE', *, *, #32159, .T. ) ;
#13254=DIRECTION ( 'NONE',  ( -0.000000000000000000, -0.000000000000000000, 1.000000000000000000 ) ) ;
#13258=EDGE_CURVE ( 'NONE', #7577, #13694, #2054, .T. ) ;
#13264=CYLINDRICAL_SURFACE ( 'NONE', #9495, 0.1000000000000028644 ) ;
#13265=ORIENTED_EDGE ( 'NONE', *, *, #27974, .T. ) ;
#13274=DIRECTION ( 'NONE',  ( 0.000000000000000000, 0.000000000000000000, 1.000000000000000000 ) ) ;
#13275=CARTESIAN_POINT ( 'NONE',  ( -40.87867591359218977, -24.55319635012989110, 6.800000000000000711 ) ) ;
#13279=LINE ( 'NONE', #6912, #11718 ) ;
#13280=ORIENTED_EDGE ( 'NONE', *, *, #9514, .F. ) ;
#13311=DIRECTION ( 'NONE',  ( 0.000000000000000000, 0.000000000000000000, 1.000000000000000000 ) ) ;
#13323=EDGE_CURVE ( 'NONE', #34397, #24284, #39084, .T. ) ;
#13327=EDGE_LOOP ( 'NONE', ( #12180, #13386, #11308, #27989 ) ) ;
#13336=DIRECTION ( 'NONE',  ( -0.000000000000000000, -0.000000000000000000, 1.000000000000000000 ) ) ;
#13337=ORIENTED_EDGE ( 'NONE', *, *, #33534, .F. ) ;
#13352=DIRECTION ( 'NONE',  ( -0.000000000000000000, -0.000000000000000000, 1.000000000000000000 ) ) ;
#13358=ORIENTED_EDGE ( 'NONE', *, *, #30, .T. ) ;
#13364=VERTEX_POINT ( 'NONE', #20353 ) ;
#13366=DIRECTION ( 'NONE',  ( 0.000000000000000000, 1.000000000000000000, 0.000000000000000000 ) ) ;
#13375=CARTESIAN_POINT ( 'NONE',  ( 5.651251297819362307, -26.64985754041175525, 6.700000000000000178 ) ) ;
#13377=VECTOR ( 'NONE', #8065, 1000.000000000000000 ) ;
#13383=EDGE_CURVE ( 'NONE', #12703, #3524, #29922, .T. ) ;
#13386=ORIENTED_EDGE ( 'NONE', *, *, #20725, .F. ) ;
#13387=EDGE_CURVE ( 'NONE', #31945, #3169, #13500, .T. ) ;
#13388=ORIENTED_EDGE ( 'NONE', *, *, #22748, .F. ) ;
#13390=CYLINDRICAL_SURFACE ( 'NONE', #32702, 0.1000000000000028644 ) ;
#13393=FACE_BOUND ( 'NONE', #27930, .T. ) ;
#13396=VERTEX_POINT ( 'NONE', #39485 ) ;
#13404=CARTESIAN_POINT ( 'NONE',  ( -28.87867591359218977, -26.64985754041175525, 6.800000000000000711 ) ) ;
#13405=FACE_OUTER_BOUND ( 'NONE', #36198, .T. ) ;
#13412=DIRECTION ( 'NONE',  ( 1.000000000000000000, 0.000000000000000000, 0.000000000000000000 ) ) ;
#13416=VECTOR ( 'NONE', #31182, 1000.000000000000000 ) ;
#13421=AXIS2_PLACEMENT_3D ( 'NONE', #205, #18933, #18717 ) ;
#13422=DIRECTION ( 'NONE',  ( 1.000000000000000000, 0.000000000000000000, 0.000000000000000000 ) ) ;
#13425=DIRECTION ( 'NONE',  ( 1.000000000000000000, 0.000000000000000000, 0.000000000000000000 ) ) ;
#13426=EDGE_CURVE ( 'NONE', #1269, #10273, #14994, .T. ) ;
#13434=ADVANCED_FACE ( 'NONE', ( #28161 ), #18905, .F. ) ;
#13435=CARTESIAN_POINT ( 'NONE',  ( 11.65737507970504616, -30.94667987854474234, 6.000000000000000000 ) ) ;
#13436=ORIENTED_EDGE ( 'NONE', *, *, #26415, .T. ) ;
#13437=VECTOR ( 'NONE', #5624, 1000.000000000000000 ) ;
#13438=CARTESIAN_POINT ( 'NONE',  ( -36.34874870218064302, -25.49307895267003587, 6.700000000000000178 ) ) ;
#13439=ADVANCED_FACE ( 'NONE', ( #37019 ), #6147, .T. ) ;
#13445=ORIENTED_EDGE ( 'NONE', *, *, #16462, .T. ) ;
#13467=CARTESIAN_POINT ( 'NONE',  ( -2.878675913592191993, -26.64985754041175525, 6.700000000000000178 ) ) ;
#13473=DIRECTION ( 'NONE',  ( 1.000000000000000000, 1.273455763949465563E-16, 0.000000000000000000 ) ) ;
#13474=AXIS2_PLACEMENT_3D ( 'NONE', #37371, #5681, #34731 ) ;
#13481=DIRECTION ( 'NONE',  ( -0.000000000000000000, -0.000000000000000000, 1.000000000000000000 ) ) ;
#13485=VERTEX_POINT ( 'NONE', #22007 ) ;
#13491=DIRECTION ( 'NONE',  ( 0.000000000000000000, 0.000000000000000000, 1.000000000000000000 ) ) ;
#13492=ORIENTED_EDGE ( 'NONE', *, *, #19769, .F. ) ;
#13497=CARTESIAN_POINT ( 'NONE',  ( -0.4487487021806388365, -25.49307895267003587, 6.800000000000000711 ) ) ;
#13500=CIRCLE ( 'NONE', #36512, 0.1000000000000028644 ) ;
#13501=CIRCLE ( 'NONE', #39835, 0.1000000000000028644 ) ;
#13508=VECTOR ( 'NONE', #4094, 1000.000000000000000 ) ;
#13522=CARTESIAN_POINT ( 'NONE',  ( -0.8786759135921904385, -26.64985754041175525, 6.800000000000000711 ) ) ;
#13529=VECTOR ( 'NONE', #15187, 1000.000000000000000 ) ;
#13530=VECTOR ( 'NONE', #33423, 1000.000000000000000 ) ;
#13531=DIRECTION ( 'NONE',  ( 1.000000000000000000, 0.000000000000000000, 0.000000000000000000 ) ) ;
#13537=LINE ( 'NONE', #28992, #22727 ) ;
#13539=ADVANCED_FACE ( 'NONE', ( #34175 ), #9219, .F. ) ;
#13550=DIRECTION ( 'NONE',  ( -0.000000000000000000, -1.000000000000000000, -0.000000000000000000 ) ) ;
#13557=DIRECTION ( 'NONE',  ( 0.000000000000000000, 0.000000000000000000, 1.000000000000000000 ) ) ;
#13558=CARTESIAN_POINT ( 'NONE',  ( -4.248748702180636272, -26.64985754041175525, 6.700000000000000178 ) ) ;
#13559=CIRCLE ( 'NONE', #6352, 0.1000000000000028644 ) ;
#13566=VECTOR ( 'NONE', #34006, 1000.000000000000000 ) ;
#13570=CARTESIAN_POINT ( 'NONE',  ( -36.34874870218064302, -25.49307895267003587, 6.800000000000000711 ) ) ;
#13576=EDGE_CURVE ( 'NONE', #25891, #3311, #12162, .T. ) ;
#13580=CARTESIAN_POINT ( 'NONE',  ( -34.44874870218064444, -26.64985754041175525, 6.700000000000000178 ) ) ;
#13581=LINE ( 'NONE', #23262, #29875 ) ;
#13582=DIRECTION ( 'NONE',  ( 0.000000000000000000, 0.000000000000000000, 1.000000000000000000 ) ) ;
#13585=CARTESIAN_POINT ( 'NONE',  ( -28.97867591359219475, -24.55319635012989110, 6.700000000000000178 ) ) ;
#13589=ORIENTED_EDGE ( 'NONE', *, *, #793, .F. ) ;
#13592=AXIS2_PLACEMENT_3D ( 'NONE', #13046, #22539, #34495 ) ;
#13594=AXIS2_PLACEMENT_3D ( 'NONE', #4567, #16687, #35666 ) ;
#13596=CIRCLE ( 'NONE', #29383, 0.1000000000000028644 ) ;
#13597=VERTEX_POINT ( 'NONE', #2877 ) ;
#13606=CARTESIAN_POINT ( 'NONE',  ( -42.44874870218064444, -25.49307895267003587, 6.700000000000000178 ) ) ;
#13613=DIRECTION ( 'NONE',  ( 0.000000000000000000, 0.000000000000000000, 1.000000000000000000 ) ) ;
#13614=AXIS2_PLACEMENT_3D ( 'NONE', #3528, #16254, #28825 ) ;
#13615=FACE_OUTER_BOUND ( 'NONE', #16576, .T. ) ;
#13617=DIRECTION ( 'NONE',  ( 0.000000000000000000, 0.000000000000000000, 1.000000000000000000 ) ) ;
#13623=EDGE_CURVE ( 'NONE', #11094, #26805, #22817, .T. ) ;
#13625=CIRCLE ( 'NONE', #11627, 0.1000000000000028644 ) ;
#13627=VECTOR ( 'NONE', #29403, 1000.000000000000000 ) ;
#13633=CARTESIAN_POINT ( 'NONE',  ( -8.248748702180632719, -26.64985754041175525, 6.700000000000000178 ) ) ;
#13634=CARTESIAN_POINT ( 'NONE',  ( -39.07867591359219261, -24.55319635012989110, 6.800000000000000711 ) ) ;
#13638=FACE_OUTER_BOUND ( 'NONE', #16839, .T. ) ;
#13641=EDGE_CURVE ( 'NONE', #7892, #12826, #8868, .T. ) ;
#13642=DIRECTION ( 'NONE',  ( -1.000000000000000000, 0.000000000000000000, 0.000000000000000000 ) ) ;
#13644=PLANE ( 'NONE',  #32498 ) ;
#13646=ORIENTED_EDGE ( 'NONE', *, *, #35490, .F. ) ;
#13653=VECTOR ( 'NONE', #37224, 1000.000000000000000 ) ;
#13654=VECTOR ( 'NONE', #28752, 1000.000000000000000 ) ;
#13656=ORIENTED_EDGE ( 'NONE', *, *, #39133, .T. ) ;
#13660=CARTESIAN_POINT ( 'NONE',  ( -30.97867591359219119, -24.55319635012989110, 6.800000000000000711 ) ) ;
#13671=DIRECTION ( 'NONE',  ( 0.000000000000000000, 0.000000000000000000, 1.000000000000000000 ) ) ;
#13679=ADVANCED_FACE ( 'NONE', ( #12930 ), #38038, .T. ) ;
#13691=VECTOR ( 'NONE', #38410, 1000.000000000000000 ) ;
#13693=DIRECTION ( 'NONE',  ( -0.000000000000000000, -0.000000000000000000, 1.000000000000000000 ) ) ;
#13694=VERTEX_POINT ( 'NONE', #35185 ) ;
#13699=DIRECTION ( 'NONE',  ( 0.000000000000000000, 0.000000000000000000, 1.000000000000000000 ) ) ;
#13717=LINE ( 'NONE', #4257, #25833 ) ;
#13719=CARTESIAN_POINT ( 'NONE',  ( -36.87867591359218977, -26.64985754041175525, 6.700000000000000178 ) ) ;
#13722=ORIENTED_EDGE ( 'NONE', *, *, #20587, .F. ) ;
#13724=EDGE_CURVE ( 'NONE', #23016, #26349, #6958, .T. ) ;
#13725=ORIENTED_EDGE ( 'NONE', *, *, #27696, .F. ) ;
#13727=DIRECTION ( 'NONE',  ( -0.000000000000000000, -0.000000000000000000, 1.000000000000000000 ) ) ;
#13729=EDGE_CURVE ( 'NONE', #36180, #29149, #32097, .T. ) ;
#13731=CYLINDRICAL_SURFACE ( 'NONE', #6401, 0.1000000000000028644 ) ;
#13732=DIRECTION ( 'NONE',  ( 1.000000000000000000, 0.000000000000000000, 0.000000000000000000 ) ) ;
#13737=DIRECTION ( 'NONE',  ( 0.000000000000000000, 0.000000000000000000, 1.000000000000000000 ) ) ;
#13740=LINE ( 'NONE', #29582, #34675 ) ;
#13745=AXIS2_PLACEMENT_3D ( 'NONE', #8242, #14832, #21232 ) ;
#13746=CARTESIAN_POINT ( 'NONE',  ( -22.34874870218063947, -25.49307895267003587, 6.700000000000000178 ) ) ;
#13753=CARTESIAN_POINT ( 'NONE',  ( -10.34874870218063769, -26.64985754041175525, 6.700000000000000178 ) ) ;
#13757=AXIS2_PLACEMENT_3D ( 'NONE', #4312, #13557, #10463 ) ;
#13767=DIRECTION ( 'NONE',  ( 1.000000000000000000, 0.000000000000000000, 0.000000000000000000 ) ) ;
#13769=VERTEX_POINT ( 'NONE', #4091 ) ;
#13770=DIRECTION ( 'NONE',  ( 1.000000000000000000, 0.000000000000000000, 0.000000000000000000 ) ) ;
#13776=EDGE_CURVE ( 'NONE', #12843, #3833, #11632, .T. ) ;
#13782=ORIENTED_EDGE ( 'NONE', *, *, #916, .F. ) ;
#13791=CARTESIAN_POINT ( 'NONE',  ( -8.248748702180632719, -26.64985754041175525, 6.700000000000000178 ) ) ;
#13793=CARTESIAN_POINT ( 'NONE',  ( -15.07867591359219439, -24.55319635012989110, 6.800000000000000711 ) ) ;
#13795=ORIENTED_EDGE ( 'NONE', *, *, #17922, .T. ) ;
#13805=ORIENTED_EDGE ( 'NONE', *, *, #4934, .F. ) ;
#13806=CARTESIAN_POINT ( 'NONE',  ( -7.078675913592194391, -24.55319635012989110, 6.700000000000000178 ) ) ;
#13811=VECTOR ( 'NONE', #39839, 1000.000000000000000 ) ;
#13812=DIRECTION ( 'NONE',  ( -0.000000000000000000, -1.000000000000000000, -0.000000000000000000 ) ) ;
#13813=VERTEX_POINT ( 'NONE', #17605 ) ;
#13820=DIRECTION ( 'NONE',  ( 1.000000000000000000, 0.000000000000000000, -0.000000000000000000 ) ) ;
#13822=EDGE_CURVE ( 'NONE', #37478, #34807, #1062, .T. ) ;
#13824=CYLINDRICAL_SURFACE ( 'NONE', #4418, 0.1000000000000028644 ) ;
#13828=CARTESIAN_POINT ( 'NONE',  ( -23.07867591359219617, -26.64985754041175525, 6.800000000000000711 ) ) ;
#13830=AXIS2_PLACEMENT_3D ( 'NONE', #19907, #16413, #16601 ) ;
#13831=CYLINDRICAL_SURFACE ( 'NONE', #17589, 0.1000000000000028644 ) ;
#13832=DIRECTION ( 'NONE',  ( 0.000000000000000000, 1.000000000000000000, 0.000000000000000000 ) ) ;
#13835=DIRECTION ( 'NONE',  ( 1.000000000000000000, 0.000000000000000000, 0.000000000000000000 ) ) ;
#13836=PLANE ( 'NONE',  #22019 ) ;
#13848=CARTESIAN_POINT ( 'NONE',  ( -4.978675913592189417, -26.64985754041175525, 6.700000000000000178 ) ) ;
#13855=ORIENTED_EDGE ( 'NONE', *, *, #10457, .T. ) ;
#13856=ADVANCED_FACE ( 'NONE', ( #1797 ), #17008, .F. ) ;
#13858=VECTOR ( 'NONE', #3995, 1000.000000000000000 ) ;
#13859=DIRECTION ( 'NONE',  ( -6.367278819747329048E-17, -1.000000000000000000, 0.000000000000000000 ) ) ;
#13862=ORIENTED_EDGE ( 'NONE', *, *, #23971, .T. ) ;
#13878=CARTESIAN_POINT ( 'NONE',  ( 1.751251297819361730, -25.49307895267003587, 6.700000000000000178 ) ) ;
#13880=EDGE_LOOP ( 'NONE', ( #7764, #33676, #927, #7793 ) ) ;
#13901=EDGE_CURVE ( 'NONE', #15938, #10309, #17208, .T. ) ;
#13902=DIRECTION ( 'NONE',  ( 0.000000000000000000, 0.000000000000000000, 1.000000000000000000 ) ) ;
#13906=DIRECTION ( 'NONE',  ( 1.000000000000000000, 0.000000000000000000, 0.000000000000000000 ) ) ;
#13911=DIRECTION ( 'NONE',  ( 1.000000000000000000, 0.000000000000000000, 0.000000000000000000 ) ) ;
#13943=DIRECTION ( 'NONE',  ( 1.000000000000000000, 0.000000000000000000, -0.000000000000000000 ) ) ;
#13946=VERTEX_POINT ( 'NONE', #40667 ) ;
#13947=CARTESIAN_POINT ( 'NONE',  ( -12.44874870218064267, -25.49307895267003587, 6.800000000000000711 ) ) ;
#13952=CARTESIAN_POINT ( 'NONE',  ( -10.44874870218064089, -26.64985754041175525, 6.800000000000000711 ) ) ;
#13956=AXIS2_PLACEMENT_3D ( 'NONE', #20334, #1238, #13770 ) ;
#13963=EDGE_LOOP ( 'NONE', ( #4746, #20130, #12294, #35654 ) ) ;
#13977=CARTESIAN_POINT ( 'NONE',  ( -36.97867591359219119, -24.55319635012989110, 6.700000000000000178 ) ) ;
#13981=CARTESIAN_POINT ( 'NONE',  ( -42.44874870218064444, -26.64985754041175525, 6.700000000000000178 ) ) ;
#13989=EDGE_LOOP ( 'NONE', ( #21002, #26661, #18107, #18404 ) ) ;
#13995=AXIS2_PLACEMENT_3D ( 'NONE', #35950, #38210, #6932 ) ;
#13998=ORIENTED_EDGE ( 'NONE', *, *, #23369, .T. ) ;
#14005=CYLINDRICAL_SURFACE ( 'NONE', #24415, 0.1000000000000028644 ) ;
#14013=CARTESIAN_POINT ( 'NONE',  ( -51.21549048184568420, -38.28842912540938670, 4.000000000000000000 ) ) ;
#14020=EDGE_LOOP ( 'NONE', ( #21649, #26957, #35140, #13145 ) ) ;
#14024=CARTESIAN_POINT ( 'NONE',  ( 1.651251297819358754, -26.64985754041175525, 6.700000000000000178 ) ) ;
#14028=DIRECTION ( 'NONE',  ( 1.000000000000000000, 0.000000000000000000, 0.000000000000000000 ) ) ;
#14035=ORIENTED_EDGE ( 'NONE', *, *, #39786, .F. ) ;
#14037=CARTESIAN_POINT ( 'NONE',  ( -22.44874870218064089, -25.49307895267003587, 6.700000000000000178 ) ) ;
#14050=ORIENTED_EDGE ( 'NONE', *, *, #13426, .T. ) ;
#14056=VECTOR ( 'NONE', #6727, 1000.000000000000000 ) ;
#14063=ORIENTED_EDGE ( 'NONE', *, *, #21819, .F. ) ;
#14066=CARTESIAN_POINT ( 'NONE',  ( -30.97867591359219119, -26.64985754041175525, 6.800000000000000711 ) ) ;
#14073=DIRECTION ( 'NONE',  ( 1.000000000000000000, -0.000000000000000000, 0.000000000000000000 ) ) ;
#14077=LINE ( 'NONE', #23754, #36864 ) ;
#14079=VERTEX_POINT ( 'NONE', #14173 ) ;
#14087=ADVANCED_FACE ( 'NONE', ( #39283 ), #20346, .T. ) ;
#14090=CARTESIAN_POINT ( 'NONE',  ( -29.07867591359219617, -24.55319635012989110, 6.800000000000000711 ) ) ;
#14091=CARTESIAN_POINT ( 'NONE',  ( -38.34874870218063592, -26.64985754041175525, 6.800000000000000711 ) ) ;
#14093=ORIENTED_EDGE ( 'NONE', *, *, #19990, .T. ) ;
#14100=AXIS2_PLACEMENT_3D ( 'NONE', #16598, #35380, #28575 ) ;
#14101=DIRECTION ( 'NONE',  ( 0.000000000000000000, 0.000000000000000000, 1.000000000000000000 ) ) ;
#14106=EDGE_LOOP ( 'NONE', ( #25025, #24376, #4728, #32609 ) ) ;
#14108=VECTOR ( 'NONE', #10742, 1000.000000000000000 ) ;
#14120=ADVANCED_FACE ( 'NONE', ( #33741 ), #32925, .F. ) ;
#14139=VECTOR ( 'NONE', #16379, 1000.000000000000000 ) ;
#14151=ADVANCED_FACE ( 'NONE', ( #27547 ), #30654, .F. ) ;
#14153=CARTESIAN_POINT ( 'NONE',  ( -51.01549048184568846, -30.38627270959228710, 6.800000000000000711 ) ) ;
#14156=LINE ( 'NONE', #26730, #12692 ) ;
#14161=CIRCLE ( 'NONE', #16803, 0.1000000000000028644 ) ;
#14164=EDGE_CURVE ( 'NONE', #14484, #4585, #2389, .T. ) ;
#14166=ORIENTED_EDGE ( 'NONE', *, *, #8349, .F. ) ;
#14172=EDGE_LOOP ( 'NONE', ( #36010, #13193, #6978, #31277 ) ) ;
#14173=CARTESIAN_POINT ( 'NONE',  ( -0.4487487021806388365, -26.64985754041175525, 6.700000000000000178 ) ) ;
#14182=EDGE_LOOP ( 'NONE', ( #39099, #27632, #15409, #30044, #18503, #7416 ) ) ;
#14184=DIRECTION ( 'NONE',  ( 1.000000000000000000, 0.000000000000000000, 0.000000000000000000 ) ) ;
#14187=ORIENTED_EDGE ( 'NONE', *, *, #11318, .F. ) ;
#14194=ORIENTED_EDGE ( 'NONE', *, *, #26487, .F. ) ;
#14197=ORIENTED_EDGE ( 'NONE', *, *, #854, .F. ) ;
#14201=VECTOR ( 'NONE', #7690, 1000.000000000000000 ) ;
#14211=DIRECTION ( 'NONE',  ( 1.000000000000000000, -0.000000000000000000, 0.000000000000000000 ) ) ;
#14212=DIRECTION ( 'NONE',  ( 1.000000000000000000, 0.000000000000000000, 0.000000000000000000 ) ) ;
#14221=EDGE_CURVE ( 'NONE', #36180, #29402, #22212, .T. ) ;
#14231=AXIS2_PLACEMENT_3D ( 'NONE', #472, #35068, #13013 ) ;
#14233=EDGE_LOOP ( 'NONE', ( #22355, #22166, #19322, #35538 ) ) ;
#14238=ORIENTED_EDGE ( 'NONE', *, *, #34163, .F. ) ;
#14245=ORIENTED_EDGE ( 'NONE', *, *, #22243, .T. ) ;
#14249=VECTOR ( 'NONE', #3132, 1000.000000000000000 ) ;
#14250=CARTESIAN_POINT ( 'NONE',  ( 11.65737507970504616, -30.94667987854474234, 6.800000000000000711 ) ) ;
#14260=AXIS2_PLACEMENT_3D ( 'NONE', #3493, #16017, #17767 ) ;
#14272=ADVANCED_FACE ( 'NONE', ( #2669 ), #15603, .T. ) ;
#14279=CARTESIAN_POINT ( 'NONE',  ( 3.551251297819357777, -26.64985754041175525, 6.700000000000000178 ) ) ;
#14287=AXIS2_PLACEMENT_3D ( 'NONE', #956, #13491, #19872 ) ;
#14295=FACE_OUTER_BOUND ( 'NONE', #2890, .T. ) ;
#14302=EDGE_CURVE ( 'NONE', #27373, #24427, #179, .T. ) ;
#14307=VECTOR ( 'NONE', #20991, 1000.000000000000000 ) ;
#14309=ORIENTED_EDGE ( 'NONE', *, *, #36356, .T. ) ;
#14313=ADVANCED_FACE ( 'NONE', ( #28155 ), #18270, .F. ) ;
#14318=DIRECTION ( 'NONE',  ( 1.000000000000000000, -0.000000000000000000, 0.000000000000000000 ) ) ;
#14324=CARTESIAN_POINT ( 'NONE',  ( -51.01549048184568846, -38.28842912540938670, 6.000000000000000000 ) ) ;
#14337=CIRCLE ( 'NONE', #20257, 0.1000000000000028644 ) ;
#14338=ORIENTED_EDGE ( 'NONE', *, *, #9779, .F. ) ;
#14342=EDGE_CURVE ( 'NONE', #8717, #39757, #14161, .T. ) ;
#14350=AXIS2_PLACEMENT_3D ( 'NONE', #36654, #28920, #23293 ) ;
#14379=CIRCLE ( 'NONE', #642, 0.1000000000000028644 ) ;
#14386=DIRECTION ( 'NONE',  ( 1.000000000000000000, -0.000000000000000000, 0.000000000000000000 ) ) ;
#14388=CARTESIAN_POINT ( 'NONE',  ( -0.9786759135921931918, -26.64985754041175525, 6.700000000000000178 ) ) ;
#14391=ORIENTED_EDGE ( 'NONE', *, *, #14719, .F. ) ;
#14404=ORIENTED_EDGE ( 'NONE', *, *, #1096, .T. ) ;
#14413=CARTESIAN_POINT ( 'NONE',  ( 7.021324086407807030, -24.55319635012989110, 6.700000000000000178 ) ) ;
#14414=AXIS2_PLACEMENT_3D ( 'NONE', #11720, #2505, #26983 ) ;
#14415=DIRECTION ( 'NONE',  ( 0.000000000000000000, 1.000000000000000000, 0.000000000000000000 ) ) ;
#14425=CARTESIAN_POINT ( 'NONE',  ( -42.83131703149249603, -32.06993018339340296, 6.000000000000000000 ) ) ;
#14428=DIRECTION ( 'NONE',  ( 1.000000000000000000, 0.000000000000000000, 0.000000000000000000 ) ) ;
#14435=EDGE_CURVE ( 'NONE', #23121, #36016, #20913, .T. ) ;
#14442=DIRECTION ( 'NONE',  ( 0.000000000000000000, 1.000000000000000000, 0.000000000000000000 ) ) ;
#14447=EDGE_CURVE ( 'NONE', #36291, #5244, #26695, .T. ) ;
#14451=CARTESIAN_POINT ( 'NONE',  ( -41.07867591359219972, -26.64985754041175525, 6.800000000000000711 ) ) ;
#14458=ORIENTED_EDGE ( 'NONE', *, *, #6383, .F. ) ;
#14468=EDGE_LOOP ( 'NONE', ( #39454, #30695, #12986, #29690 ) ) ;
#14476=DIRECTION ( 'NONE',  ( -0.000000000000000000, -0.000000000000000000, 1.000000000000000000 ) ) ;
#14479=LINE ( 'NONE', #30353, #7923 ) ;
#14480=CARTESIAN_POINT ( 'NONE',  ( -2.348748702180637693, -26.64985754041175525, 6.700000000000000178 ) ) ;
#14484=VERTEX_POINT ( 'NONE', #8338 ) ;
#14487=AXIS2_PLACEMENT_3D ( 'NONE', #12823, #25595, #25192 ) ;
#14493=DIRECTION ( 'NONE',  ( -1.000000000000000000, 0.000000000000000000, -0.000000000000000000 ) ) ;
#14494=LINE ( 'NONE', #24384, #38315 ) ;
#14497=ADVANCED_FACE ( 'NONE', ( #33695 ), #11624, .F. ) ;
#14505=CARTESIAN_POINT ( 'NONE',  ( -10.24874870218063450, -26.64985754041175525, 6.700000000000000178 ) ) ;
#14509=ORIENTED_EDGE ( 'NONE', *, *, #2459, .F. ) ;
#14511=CIRCLE ( 'NONE', #9946, 0.1000000000000028644 ) ;
#14520=FACE_OUTER_BOUND ( 'NONE', #18536, .T. ) ;
#14535=ORIENTED_EDGE ( 'NONE', *, *, #17686, .F. ) ;
#14537=ADVANCED_FACE ( 'NONE', ( #14520 ), #24202, .F. ) ;
#14543=ORIENTED_EDGE ( 'NONE', *, *, #17741, .F. ) ;
#14546=VECTOR ( 'NONE', #16476, 1000.000000000000000 ) ;
#14547=FACE_OUTER_BOUND ( 'NONE', #36207, .T. ) ;
#14549=CARTESIAN_POINT ( 'NONE',  ( -2.248748702180634940, -26.64985754041175525, 6.700000000000000178 ) ) ;
#14554=DIRECTION ( 'NONE',  ( 0.000000000000000000, -1.000000000000000000, 0.000000000000000000 ) ) ;
#14558=LINE ( 'NONE', #39476, #32733 ) ;
#14563=EDGE_CURVE ( 'NONE', #10365, #32868, #1728, .T. ) ;
#14567=CARTESIAN_POINT ( 'NONE',  ( 3.121324086407806231, -26.64985754041175525, 6.700000000000000178 ) ) ;
#14570=CARTESIAN_POINT ( 'NONE',  ( -12.44874870218064267, -26.64985754041175525, 6.700000000000000178 ) ) ;
#14571=VERTEX_POINT ( 'NONE', #23989 ) ;
#14573=LINE ( 'NONE', #17675, #14307 ) ;
#14576=VERTEX_POINT ( 'NONE', #2198 ) ;
#14581=VECTOR ( 'NONE', #39300, 1000.000000000000000 ) ;
#14582=DIRECTION ( 'NONE',  ( 0.000000000000000000, 1.000000000000000000, 0.000000000000000000 ) ) ;
#14583=ORIENTED_EDGE ( 'NONE', *, *, #36526, .F. ) ;
#14592=CARTESIAN_POINT ( 'NONE',  ( -40.87867591359218977, -24.55319635012989110, 6.700000000000000178 ) ) ;
#14621=DIRECTION ( 'NONE',  ( 1.000000000000000000, 0.000000000000000000, 0.000000000000000000 ) ) ;
#14626=VERTEX_POINT ( 'NONE', #21740 ) ;
#14632=DIRECTION ( 'NONE',  ( 1.000000000000000000, 0.000000000000000000, 0.000000000000000000 ) ) ;
#14633=DIRECTION ( 'NONE',  ( 0.000000000000000000, 1.000000000000000000, 0.000000000000000000 ) ) ;
#14634=ORIENTED_EDGE ( 'NONE', *, *, #9368, .F. ) ;
#14640=CARTESIAN_POINT ( 'NONE',  ( -4.878675913592187108, -26.64985754041175525, 6.800000000000000711 ) ) ;
#14647=ORIENTED_EDGE ( 'NONE', *, *, #33943, .T. ) ;
#14653=VERTEX_POINT ( 'NONE', #9364 ) ;
#14654=AXIS2_PLACEMENT_3D ( 'NONE', #23358, #1352, #17157 ) ;
#14656=VERTEX_POINT ( 'NONE', #11828 ) ;
#14671=EDGE_CURVE ( 'NONE', #11908, #26319, #18846, .T. ) ;
#14687=AXIS2_PLACEMENT_3D ( 'NONE', #17776, #30362, #2169 ) ;
#14689=CIRCLE ( 'NONE', #16003, 0.1000000000000028644 ) ;
#14694=PLANE ( 'NONE',  #19894 ) ;
#14695=ORIENTED_EDGE ( 'NONE', *, *, #264, .T. ) ;
#14697=ORIENTED_EDGE ( 'NONE', *, *, #17587, .T. ) ;
#14710=CIRCLE ( 'NONE', #35791, 7.341749246864647915 ) ;
#14715=CARTESIAN_POINT ( 'NONE',  ( -7.078675913592194391, -26.64985754041175525, 6.800000000000000711 ) ) ;
#14719=EDGE_CURVE ( 'NONE', #23027, #33929, #19473, .T. ) ;
#14720=EDGE_CURVE ( 'NONE', #10898, #22409, #15760, .T. ) ;
#14729=CYLINDRICAL_SURFACE ( 'NONE', #19455, 0.1000000000000028644 ) ;
#14738=DIRECTION ( 'NONE',  ( -0.000000000000000000, -0.000000000000000000, 1.000000000000000000 ) ) ;
#14739=AXIS2_PLACEMENT_3D ( 'NONE', #38933, #25794, #13422 ) ;
#14740=VECTOR ( 'NONE', #15082, 1000.000000000000000 ) ;
#14754=DIRECTION ( 'NONE',  ( -0.000000000000000000, -0.000000000000000000, 1.000000000000000000 ) ) ;
#14760=CARTESIAN_POINT ( 'NONE',  ( -20.44874870218064444, -25.49307895267003587, 6.800000000000000711 ) ) ;
#14763=VERTEX_POINT ( 'NONE', #40444 ) ;
#14768=ORIENTED_EDGE ( 'NONE', *, *, #15097, .T. ) ;
#14770=ORIENTED_EDGE ( 'NONE', *, *, #14435, .T. ) ;
#14771=CIRCLE ( 'NONE', #14739, 0.1000000000000028644 ) ;
#14775=EDGE_CURVE ( 'NONE', #7027, #33685, #10894, .T. ) ;
#14790=LINE ( 'NONE', #27359, #23108 ) ;
#14791=CARTESIAN_POINT ( 'NONE',  ( -16.87867591359218977, -26.64985754041175525, 6.700000000000000178 ) ) ;
#14792=ORIENTED_EDGE ( 'NONE', *, *, #7675, .F. ) ;
#14802=ORIENTED_EDGE ( 'NONE', *, *, #20208, .T. ) ;
#14804=AXIS2_PLACEMENT_3D ( 'NONE', #17055, #35628, #22860 ) ;
#14814=AXIS2_PLACEMENT_3D ( 'NONE', #35882, #27755, #36824 ) ;
#14827=EDGE_CURVE ( 'NONE', #10700, #22883, #14935, .T. ) ;
#14829=CARTESIAN_POINT ( 'NONE',  ( -27.07867591359219972, -24.55319635012989110, 6.800000000000000711 ) ) ;
#14830=DIRECTION ( 'NONE',  ( -0.000000000000000000, -0.000000000000000000, 1.000000000000000000 ) ) ;
#14832=DIRECTION ( 'NONE',  ( 0.000000000000000000, 0.000000000000000000, 1.000000000000000000 ) ) ;
#14833=DIRECTION ( 'NONE',  ( 1.000000000000000000, 0.000000000000000000, 0.000000000000000000 ) ) ;
#14834=CIRCLE ( 'NONE', #7619, 0.1000000000000028644 ) ;
#14839=CIRCLE ( 'NONE', #36546, 0.1000000000000028644 ) ;
#14840=ADVANCED_FACE ( 'NONE', ( #30814 ), #37169, .F. ) ;
#14846=DIRECTION ( 'NONE',  ( -0.000000000000000000, -1.000000000000000000, -0.000000000000000000 ) ) ;
#14855=EDGE_LOOP ( 'NONE', ( #16179, #39607, #32940, #17836 ) ) ;
#14863=EDGE_LOOP ( 'NONE', ( #3068, #38342, #2136, #4890 ) ) ;
#14870=CIRCLE ( 'NONE', #12947, 0.1000000000000028644 ) ;
#14872=DIRECTION ( 'NONE',  ( 1.000000000000000000, 0.000000000000000000, 0.000000000000000000 ) ) ;
#14875=AXIS2_PLACEMENT_3D ( 'NONE', #16892, #29472, #13820 ) ;
#14887=DIRECTION ( 'NONE',  ( 0.000000000000000000, 0.000000000000000000, -1.000000000000000000 ) ) ;
#14892=CYLINDRICAL_SURFACE ( 'NONE', #8688, 0.1000000000000028644 ) ;
#14894=ORIENTED_EDGE ( 'NONE', *, *, #19980, .F. ) ;
#14897=EDGE_CURVE ( 'NONE', #17894, #5789, #16002, .T. ) ;
#14899=EDGE_LOOP ( 'NONE', ( #38795, #6998, #40700, #11009 ) ) ;
#14909=VECTOR ( 'NONE', #8601, 1000.000000000000000 ) ;
#14910=FACE_OUTER_BOUND ( 'NONE', #18278, .T. ) ;
#14915=EDGE_CURVE ( 'NONE', #34445, #25426, #22602, .T. ) ;
#14916=EDGE_LOOP ( 'NONE', ( #27546, #21714, #5139, #10655 ) ) ;
#14935=LINE ( 'NONE', #5680, #10723 ) ;
#14937=VECTOR ( 'NONE', #39200, 1000.000000000000000 ) ;
#14939=CIRCLE ( 'NONE', #20845, 0.1000000000000028644 ) ;
#14940=DIRECTION ( 'NONE',  ( 0.000000000000000000, 0.000000000000000000, 1.000000000000000000 ) ) ;
#14948=CARTESIAN_POINT ( 'NONE',  ( -34.87867591359218977, -26.64985754041175525, 6.700000000000000178 ) ) ;
#14952=ORIENTED_EDGE ( 'NONE', *, *, #3447, .T. ) ;
#14954=CYLINDRICAL_SURFACE ( 'NONE', #23915, 0.1000000000000028644 ) ;
#14963=VECTOR ( 'NONE', #13366, 1000.000000000000000 ) ;
#14967=VECTOR ( 'NONE', #9804, 1000.000000000000000 ) ;
#14971=DIRECTION ( 'NONE',  ( 0.000000000000000000, 0.000000000000000000, 1.000000000000000000 ) ) ;
#14975=CARTESIAN_POINT ( 'NONE',  ( -38.87867591359218977, -26.64985754041175525, 6.700000000000000178 ) ) ;
#14988=DIRECTION ( 'NONE',  ( 0.000000000000000000, 0.000000000000000000, 1.000000000000000000 ) ) ;
#14990=VECTOR ( 'NONE', #26398, 1000.000000000000000 ) ;
#14991=LINE ( 'NONE', #9011, #13183 ) ;
#14994=LINE ( 'NONE', #15194, #30589 ) ;
#14998=ORIENTED_EDGE ( 'NONE', *, *, #24174, .F. ) ;
#15004=PLANE ( 'NONE',  #33637 ) ;
#15006=DIRECTION ( 'NONE',  ( 0.000000000000000000, 0.000000000000000000, 1.000000000000000000 ) ) ;
#15008=ORIENTED_EDGE ( 'NONE', *, *, #7794, .T. ) ;
#15017=ADVANCED_FACE ( 'NONE', ( #2157 ), #17351, .F. ) ;
#15019=EDGE_CURVE ( 'NONE', #30682, #26162, #4831, .T. ) ;
#15055=ORIENTED_EDGE ( 'NONE', *, *, #18627, .F. ) ;
#15060=DIRECTION ( 'NONE',  ( 0.000000000000000000, 0.000000000000000000, 1.000000000000000000 ) ) ;
#15068=EDGE_CURVE ( 'NONE', #273, #1547, #3541, .T. ) ;
#15082=DIRECTION ( 'NONE',  ( -0.000000000000000000, -0.000000000000000000, 1.000000000000000000 ) ) ;
#15085=AXIS2_PLACEMENT_3D ( 'NONE', #16696, #3586, #6855 ) ;
#15086=CARTESIAN_POINT ( 'NONE',  ( -34.44874870218064444, -25.49307895267003587, 6.800000000000000711 ) ) ;
#15089=CARTESIAN_POINT ( 'NONE',  ( -4.348748702180639469, -25.49307895267003587, 6.700000000000000178 ) ) ;
#15093=CARTESIAN_POINT ( 'NONE',  ( -21.07867591359219617, -24.55319635012989110, 6.700000000000000178 ) ) ;
#15097=EDGE_CURVE ( 'NONE', #25288, #18231, #36718, .T. ) ;
#15101=VECTOR ( 'NONE', #7036, 1000.000000000000000 ) ;
#15103=EDGE_CURVE ( 'NONE', #34769, #18315, #16962, .T. ) ;
#15108=DIRECTION ( 'NONE',  ( 1.000000000000000000, 0.000000000000000000, 0.000000000000000000 ) ) ;
#15109=CARTESIAN_POINT ( 'NONE',  ( -0.8786759135921904385, -24.55319635012989110, 6.700000000000000178 ) ) ;
#15115=ORIENTED_EDGE ( 'NONE', *, *, #23481, .T. ) ;
#15117=AXIS2_PLACEMENT_3D ( 'NONE', #5818, #27629, #29754 ) ;
#15118=FACE_OUTER_BOUND ( 'NONE', #35639, .T. ) ;
#15120=EDGE_LOOP ( 'NONE', ( #38607, #10928, #18870, #14697 ) ) ;
#15125=ORIENTED_EDGE ( 'NONE', *, *, #35181, .T. ) ;
#15127=VECTOR ( 'NONE', #28500, 1000.000000000000000 ) ;
#15129=ORIENTED_EDGE ( 'NONE', *, *, #13258, .F. ) ;
#15140=AXIS2_PLACEMENT_3D ( 'NONE', #40447, #8752, #21546 ) ;
#15145=ORIENTED_EDGE ( 'NONE', *, *, #18630, .T. ) ;
#15151=LINE ( 'NONE', #31431, #29960 ) ;
#15154=AXIS2_PLACEMENT_3D ( 'NONE', #30501, #27196, #23702 ) ;
#15160=ORIENTED_EDGE ( 'NONE', *, *, #1148, .F. ) ;
#15162=ORIENTED_EDGE ( 'NONE', *, *, #34569, .T. ) ;
#15179=ADVANCED_FACE ( 'NONE', ( #6249 ), #25186, .T. ) ;
#15187=DIRECTION ( 'NONE',  ( -1.000000000000000000, 6.367278819747327815E-17, -0.000000000000000000 ) ) ;
#15190=FACE_OUTER_BOUND ( 'NONE', #28554, .T. ) ;
#15194=CARTESIAN_POINT ( 'NONE',  ( -23.07867591359219617, -26.64985754041175525, 6.700000000000000178 ) ) ;
#15196=DIRECTION ( 'NONE',  ( 1.000000000000000000, 0.000000000000000000, 0.000000000000000000 ) ) ;
#15212=AXIS2_PLACEMENT_3D ( 'NONE', #4559, #26183, #10313 ) ;
#15221=LINE ( 'NONE', #24698, #7106 ) ;
#15242=AXIS2_PLACEMENT_3D ( 'NONE', #8782, #30012, #36394 ) ;
#15249=EDGE_CURVE ( 'NONE', #9234, #12066, #2776, .T. ) ;
#15262=PLANE ( 'NONE',  #35199 ) ;
#15264=LINE ( 'NONE', #14640, #414 ) ;
#15265=DIRECTION ( 'NONE',  ( 0.000000000000000000, 0.000000000000000000, 1.000000000000000000 ) ) ;
#15280=AXIS2_PLACEMENT_3D ( 'NONE', #10136, #13642, #19422 ) ;
#15294=DIRECTION ( 'NONE',  ( 0.000000000000000000, 0.000000000000000000, 1.000000000000000000 ) ) ;
#15295=DIRECTION ( 'NONE',  ( -1.000000000000000000, 0.000000000000000000, 0.000000000000000000 ) ) ;
#15299=CYLINDRICAL_SURFACE ( 'NONE', #33197, 0.1000000000000028644 ) ;
#15303=DIRECTION ( 'NONE',  ( 0.000000000000000000, 0.000000000000000000, 1.000000000000000000 ) ) ;
#15304=VECTOR ( 'NONE', #8323, 1000.000000000000000 ) ;
#15305=CARTESIAN_POINT ( 'NONE',  ( -3.078675913592197944, -24.55319635012989110, 6.700000000000000178 ) ) ;
#15309=DIRECTION ( 'NONE',  ( -0.000000000000000000, -0.000000000000000000, 1.000000000000000000 ) ) ;
#15323=ORIENTED_EDGE ( 'NONE', *, *, #40555, .T. ) ;
#15334=STYLED_ITEM('',(#40773),#26090);
#15336=EDGE_CURVE ( 'NONE', #3101, #31945, #18179, .T. ) ;
#15337=CARTESIAN_POINT ( 'NONE',  ( -4.878675913592187108, -24.55319635012989110, 6.700000000000000178 ) ) ;
#15352=EDGE_LOOP ( 'NONE', ( #21989, #16487, #25528, #39191 ) ) ;
#15357=LINE ( 'NONE', #31837, #31955 ) ;
#15360=EDGE_LOOP ( 'NONE', ( #22640, #19612, #13116, #8642 ) ) ;
#15363=EDGE_CURVE ( 'NONE', #6556, #8986, #3398, .T. ) ;
#15366=VERTEX_POINT ( 'NONE', #35626 ) ;
#15373=VECTOR ( 'NONE', #36935, 1000.000000000000000 ) ;
#15378=CARTESIAN_POINT ( 'NONE',  ( -51.01549048184568846, -30.38627270959228710, 6.800000000000000711 ) ) ;
#15386=VECTOR ( 'NONE', #3003, 1000.000000000000000 ) ;
#15389=FACE_OUTER_BOUND ( 'NONE', #26315, .T. ) ;
#15399=DIRECTION ( 'NONE',  ( 0.000000000000000000, 0.000000000000000000, 1.000000000000000000 ) ) ;
#15409=ORIENTED_EDGE ( 'NONE', *, *, #22662, .T. ) ;
#15419=EDGE_CURVE ( 'NONE', #38102, #513, #40498, .T. ) ;
#15434=AXIS2_PLACEMENT_3D ( 'NONE', #22767, #29134, #25034 ) ;
#15439=AXIS2_PLACEMENT_3D ( 'NONE', #9785, #31827, #19667 ) ;
#15443=CARTESIAN_POINT ( 'NONE',  ( -22.87867591359218977, -24.55319635012989110, 6.800000000000000711 ) ) ;
#15456=VERTEX_POINT ( 'NONE', #38036 ) ;
#15460=ORIENTED_EDGE ( 'NONE', *, *, #33958, .T. ) ;
#15463=DIRECTION ( 'NONE',  ( -0.000000000000000000, -0.000000000000000000, 1.000000000000000000 ) ) ;
#15465=CARTESIAN_POINT ( 'NONE',  ( -40.87867591359218977, -26.64985754041175525, 6.800000000000000711 ) ) ;
#15472=FACE_OUTER_BOUND ( 'NONE', #28042, .T. ) ;
#15482=EDGE_CURVE ( 'NONE', #33264, #2584, #6561, .T. ) ;
#15488=CARTESIAN_POINT ( 'NONE',  ( -16.87867591359218977, -24.55319635012989110, 6.700000000000000178 ) ) ;
#15499=VECTOR ( 'NONE', #3364, 1000.000000000000000 ) ;
#15501=DIRECTION ( 'NONE',  ( -0.000000000000000000, -0.000000000000000000, 1.000000000000000000 ) ) ;
#15508=DIRECTION ( 'NONE',  ( -0.000000000000000000, -1.000000000000000000, -0.000000000000000000 ) ) ;
#15514=ORIENTED_EDGE ( 'NONE', *, *, #3095, .T. ) ;
#15518=EDGE_LOOP ( 'NONE', ( #34821, #2438, #22012, #4159 ) ) ;
#15523=DIRECTION ( 'NONE',  ( 1.000000000000000000, 0.000000000000000000, 0.000000000000000000 ) ) ;
#15536=CIRCLE ( 'NONE', #7016, 0.1000000000000028644 ) ;
#15553=CARTESIAN_POINT ( 'NONE',  ( -41.07867591359219972, -24.55319635012989110, 6.700000000000000178 ) ) ;
#15556=CARTESIAN_POINT ( 'NONE',  ( -12.44874870218064267, -26.64985754041175525, 6.700000000000000178 ) ) ;
#15565=EDGE_CURVE ( 'NONE', #38692, #11094, #21982, .T. ) ;
#15577=CYLINDRICAL_SURFACE ( 'NONE', #30680, 0.1000000000000028644 ) ;
#15579=ORIENTED_EDGE ( 'NONE', *, *, #24794, .F. ) ;
#15584=EDGE_LOOP ( 'NONE', ( #16664, #27963, #17029, #26122 ) ) ;
#15585=AXIS2_PLACEMENT_3D ( 'NONE', #38676, #17244, #4324 ) ;
#15587=EDGE_CURVE ( 'NONE', #18339, #30328, #25691, .T. ) ;
#15588=CARTESIAN_POINT ( 'NONE',  ( -2.978675913592195190, -24.55319635012989110, 6.700000000000000178 ) ) ;
#15592=CARTESIAN_POINT ( 'NONE',  ( -16.34874870218063592, -26.64985754041175525, 6.700000000000000178 ) ) ;
#15603=PLANE ( 'NONE',  #34605 ) ;
#15609=DIRECTION ( 'NONE',  ( 0.000000000000000000, 0.000000000000000000, -1.000000000000000000 ) ) ;
#15615=DIRECTION ( 'NONE',  ( 0.000000000000000000, 0.000000000000000000, 1.000000000000000000 ) ) ;
#15619=DIRECTION ( 'NONE',  ( 1.000000000000000000, 0.000000000000000000, 0.000000000000000000 ) ) ;
#15620=CIRCLE ( 'NONE', #5748, 0.1000000000000028644 ) ;
#15622=ORIENTED_EDGE ( 'NONE', *, *, #19078, .T. ) ;
#15625=ORIENTED_EDGE ( 'NONE', *, *, #27918, .F. ) ;
#15627=VERTEX_POINT ( 'NONE', #4482 ) ;
#15630=ORIENTED_EDGE ( 'NONE', *, *, #31064, .F. ) ;
#15633=ORIENTED_EDGE ( 'NONE', *, *, #33161, .T. ) ;
#15639=CARTESIAN_POINT ( 'NONE',  ( -32.24874870218063450, -26.64985754041175525, 6.700000000000000178 ) ) ;
#15645=CARTESIAN_POINT ( 'NONE',  ( -14.24874870218063450, -26.64985754041175525, 6.800000000000000711 ) ) ;
#15649=ORIENTED_EDGE ( 'NONE', *, *, #38711, .F. ) ;
#15660=PLANE ( 'NONE',  #10554 ) ;
#15664=ORIENTED_EDGE ( 'NONE', *, *, #3167, .T. ) ;
#15674=CARTESIAN_POINT ( 'NONE',  ( -13.07867591359219617, -24.55319635012989110, 6.800000000000000711 ) ) ;
#15675=( LENGTH_UNIT ( ) NAMED_UNIT ( * ) SI_UNIT ( .MILLI., .METRE. ) );
#15677=FACE_BOUND ( 'NONE', #37503, .T. ) ;
#15691=ORIENTED_EDGE ( 'NONE', *, *, #8969, .T. ) ;
#15692=CARTESIAN_POINT ( 'NONE',  ( -36.97867591359219119, -24.55319635012989110, 6.700000000000000178 ) ) ;
#15693=CIRCLE ( 'NONE', #18995, 0.1000000000000028644 ) ;
#15704=EDGE_CURVE ( 'NONE', #39964, #12335, #7948, .T. ) ;
#15714=EDGE_CURVE ( 'NONE', #1980, #25803, #20498, .T. ) ;
#15716=CIRCLE ( 'NONE', #1273, 0.1000000000000028644 ) ;
#15718=EDGE_CURVE ( 'NONE', #9410, #6472, #943, .T. ) ;
#15719=LINE ( 'NONE', #27860, #1490 ) ;
#15722=DIRECTION ( 'NONE',  ( 0.000000000000000000, 0.000000000000000000, 1.000000000000000000 ) ) ;
#15724=EDGE_CURVE ( 'NONE', #26758, #19353, #20919, .T. ) ;
#15729=CARTESIAN_POINT ( 'NONE',  ( 1.021324086407808585, -24.55319635012989110, 6.700000000000000178 ) ) ;
#15731=CARTESIAN_POINT ( 'NONE',  ( -36.24874870218063450, -26.64985754041175525, 6.800000000000000711 ) ) ;
#15736=FACE_OUTER_BOUND ( 'NONE', #15869, .T. ) ;
#15760=LINE ( 'NONE', #21948, #35908 ) ;
#15763=CARTESIAN_POINT ( 'NONE',  ( -4.448748702180642667, -26.64985754041175525, 6.800000000000000711 ) ) ;
#15775=CARTESIAN_POINT ( 'NONE',  ( 11.65737507970504439, -23.60493063168009442, 6.000000000000000000 ) ) ;
#15785=DIRECTION ( 'NONE',  ( -0.000000000000000000, -0.000000000000000000, -1.000000000000000000 ) ) ;
#15795=VERTEX_POINT ( 'NONE', #23026 ) ;
#15800=DIRECTION ( 'NONE',  ( 0.000000000000000000, 0.000000000000000000, 1.000000000000000000 ) ) ;
#15802=ORIENTED_EDGE ( 'NONE', *, *, #30918, .F. ) ;
#15810=CARTESIAN_POINT ( 'NONE',  ( -22.87867591359218977, -26.64985754041175525, 6.800000000000000711 ) ) ;
#15816=VECTOR ( 'NONE', #7606, 1000.000000000000000 ) ;
#15824=VERTEX_POINT ( 'NONE', #1408 ) ;
#15827=DIRECTION ( 'NONE',  ( -0.000000000000000000, -0.000000000000000000, 1.000000000000000000 ) ) ;
#15829=DIRECTION ( 'NONE',  ( 0.000000000000000000, 0.000000000000000000, 1.000000000000000000 ) ) ;
#15833=ORIENTED_EDGE ( 'NONE', *, *, #19360, .T. ) ;
#15841=DIRECTION ( 'NONE',  ( -0.000000000000000000, -0.000000000000000000, 1.000000000000000000 ) ) ;
#15843=LINE ( 'NONE', #12957, #12602 ) ;
#15854=ORIENTED_EDGE ( 'NONE', *, *, #8041, .T. ) ;
#15855=EDGE_CURVE ( 'NONE', #9480, #38999, #30406, .T. ) ;
#15856=AXIS2_PLACEMENT_3D ( 'NONE', #19162, #16268, #22673 ) ;
#15863=LINE ( 'NONE', #35235, #22893 ) ;
#15865=AXIS2_PLACEMENT_3D ( 'NONE', #27154, #1863, #18289 ) ;
#15866=FACE_OUTER_BOUND ( 'NONE', #33528, .T. ) ;
#15867=ADVANCED_FACE ( 'NONE', ( #18034 ), #14954, .F. ) ;
#15869=EDGE_LOOP ( 'NONE', ( #8002, #1866, #23767, #32108 ) ) ;
#15879=FACE_BOUND ( 'NONE', #121, .T. ) ;
#15880=CARTESIAN_POINT ( 'NONE',  ( 5.551251297819359110, -25.49307895267003587, 6.800000000000000711 ) ) ;
#15881=ORIENTED_EDGE ( 'NONE', *, *, #907, .F. ) ;
#15894=CARTESIAN_POINT ( 'NONE',  ( -32.87867591359218977, -24.55319635012989110, 6.700000000000000178 ) ) ;
#15898=DIRECTION ( 'NONE',  ( -0.000000000000000000, -1.000000000000000000, -0.000000000000000000 ) ) ;
#15902=ADVANCED_FACE ( 'NONE', ( #15866 ), #25548, .F. ) ;
#15904=CARTESIAN_POINT ( 'NONE',  ( -26.34874870218063947, -26.64985754041175525, 6.700000000000000178 ) ) ;
#15909=CARTESIAN_POINT ( 'NONE',  ( -2.248748702180634940, -25.49307895267003587, 6.800000000000000711 ) ) ;
#15918=ORIENTED_EDGE ( 'NONE', *, *, #6850, .F. ) ;
#15923=CARTESIAN_POINT ( 'NONE',  ( -35.07867591359219972, -26.64985754041175525, 6.800000000000000711 ) ) ;
#15928=VERTEX_POINT ( 'NONE', #13793 ) ;
#15932=EDGE_LOOP ( 'NONE', ( #13039, #8935, #23030, #2940 ) ) ;
#15938=VERTEX_POINT ( 'NONE', #29444 ) ;
#15945=LINE ( 'NONE', #3022, #31208 ) ;
#15946=ORIENTED_EDGE ( 'NONE', *, *, #19911, .T. ) ;
#15951=EDGE_CURVE ( 'NONE', #10008, #13769, #11416, .T. ) ;
#15952=CYLINDRICAL_SURFACE ( 'NONE', #37948, 0.1000000000000028644 ) ;
#15978=CARTESIAN_POINT ( 'NONE',  ( -38.44874870218063734, -25.49307895267003587, 6.800000000000000711 ) ) ;
#15981=ORIENTED_EDGE ( 'NONE', *, *, #236, .T. ) ;
#16002=CIRCLE ( 'NONE', #11388, 0.1000000000000028644 ) ;
#16003=AXIS2_PLACEMENT_3D ( 'NONE', #13660, #39158, #2542 ) ;
#16011=ORIENTED_EDGE ( 'NONE', *, *, #22804, .F. ) ;
#16017=DIRECTION ( 'NONE',  ( 0.000000000000000000, 0.000000000000000000, 1.000000000000000000 ) ) ;
#16023=CARTESIAN_POINT ( 'NONE',  ( -7.078675913592194391, -26.64985754041175525, 6.700000000000000178 ) ) ;
#16026=PLANE ( 'NONE',  #32625 ) ;
#16028=DIRECTION ( 'NONE',  ( -0.000000000000000000, -1.000000000000000000, -0.000000000000000000 ) ) ;
#16029=VECTOR ( 'NONE', #20668, 1000.000000000000000 ) ;
#16030=AXIS2_PLACEMENT_3D ( 'NONE', #14250, #7476, #23537 ) ;
#16036=ORIENTED_EDGE ( 'NONE', *, *, #8041, .F. ) ;
#16055=VERTEX_POINT ( 'NONE', #11793 ) ;
#16059=VECTOR ( 'NONE', #21207, 1000.000000000000000 ) ;
#16060=AXIS2_PLACEMENT_3D ( 'NONE', #31813, #16153, #28717 ) ;
#16064=CARTESIAN_POINT ( 'NONE',  ( 3.751251297819363728, -25.49307895267003587, 6.700000000000000178 ) ) ;
#16065=EDGE_LOOP ( 'NONE', ( #21812, #8755, #23082, #9649 ) ) ;
#16067=AXIS2_PLACEMENT_3D ( 'NONE', #35478, #35876, #19813 ) ;
#16068=FACE_OUTER_BOUND ( 'NONE', #19425, .T. ) ;
#16075=ORIENTED_EDGE ( 'NONE', *, *, #2258, .F. ) ;
#16082=LINE ( 'NONE', #19380, #3048 ) ;
#16098=EDGE_LOOP ( 'NONE', ( #22875, #30119, #32630, #15833 ) ) ;
#16102=EDGE_CURVE ( 'NONE', #19329, #35983, #17985, .T. ) ;
#16106=DIRECTION ( 'NONE',  ( -0.000000000000000000, -1.000000000000000000, -0.000000000000000000 ) ) ;
#16119=EDGE_CURVE ( 'NONE', #33685, #13364, #39608, .T. ) ;
#16130=LINE ( 'NONE', #37536, #21295 ) ;
#16134=EDGE_CURVE ( 'NONE', #6556, #27970, #10750, .T. ) ;
#16135=EDGE_CURVE ( 'NONE', #169, #25414, #27666, .T. ) ;
#16149=VECTOR ( 'NONE', #194, 1000.000000000000000 ) ;
#16150=ADVANCED_FACE ( 'NONE', ( #36531 ), #5238, .F. ) ;
#16153=DIRECTION ( 'NONE',  ( 0.000000000000000000, 0.000000000000000000, 1.000000000000000000 ) ) ;
#16165=CARTESIAN_POINT ( 'NONE',  ( -36.34874870218064302, -26.64985754041175525, 6.800000000000000711 ) ) ;
#16168=CARTESIAN_POINT ( 'NONE',  ( -32.34874870218063592, -26.64985754041175525, 6.700000000000000178 ) ) ;
#16170=CARTESIAN_POINT ( 'NONE',  ( -36.24874870218063450, -25.49307895267003587, 6.700000000000000178 ) ) ;
#16171=EDGE_LOOP ( 'NONE', ( #14647, #39765, #29111, #25307 ) ) ;
#16177=EDGE_CURVE ( 'NONE', #26349, #7986, #12834, .T. ) ;
#16179=ORIENTED_EDGE ( 'NONE', *, *, #24487, .T. ) ;
#16190=DIRECTION ( 'NONE',  ( 1.000000000000000000, 0.000000000000000000, 0.000000000000000000 ) ) ;
#16193=CARTESIAN_POINT ( 'NONE',  ( -11.07867591359219794, -24.55319635012989110, 6.800000000000000711 ) ) ;
#16196=FACE_OUTER_BOUND ( 'NONE', #30269, .T. ) ;
#16198=FACE_OUTER_BOUND ( 'NONE', #19479, .T. ) ;
#16202=EDGE_LOOP ( 'NONE', ( #34144, #31191, #1439, #24185 ) ) ;
#16215=CARTESIAN_POINT ( 'NONE',  ( -22.44874870218064089, -26.64985754041175525, 6.800000000000000711 ) ) ;
#16225=DIRECTION ( 'NONE',  ( 0.000000000000000000, 0.000000000000000000, 1.000000000000000000 ) ) ;
#16228=LINE ( 'NONE', #25506, #16149 ) ;
#16229=EDGE_CURVE ( 'NONE', #21394, #20712, #24582, .T. ) ;
#16232=AXIS2_PLACEMENT_3D ( 'NONE', #33923, #21558, #6313 ) ;
#16234=ORIENTED_EDGE ( 'NONE', *, *, #32592, .T. ) ;
#16237=AXIS2_PLACEMENT_3D ( 'NONE', #21806, #15827, #15619 ) ;
#16239=CIRCLE ( 'NONE', #3112, 0.1000000000000028644 ) ;
#16250=ORIENTED_EDGE ( 'NONE', *, *, #6059, .F. ) ;
#16254=DIRECTION ( 'NONE',  ( 0.000000000000000000, 0.000000000000000000, 1.000000000000000000 ) ) ;
#16256=ORIENTED_EDGE ( 'NONE', *, *, #30787, .F. ) ;
#16268=DIRECTION ( 'NONE',  ( -0.000000000000000000, -0.000000000000000000, 1.000000000000000000 ) ) ;
#16271=ORIENTED_EDGE ( 'NONE', *, *, #26830, .T. ) ;
#16273=CARTESIAN_POINT ( 'NONE',  ( -44.23414840393349579, -30.38627270959228710, 6.800000000000000711 ) ) ;
#16275=EDGE_CURVE ( 'NONE', #9053, #9101, #16130, .T. ) ;
#16281=DIRECTION ( 'NONE',  ( -0.000000000000000000, -0.000000000000000000, 1.000000000000000000 ) ) ;
#16282=CARTESIAN_POINT ( 'NONE',  ( -22.87867591359218977, -26.64985754041175525, 6.700000000000000178 ) ) ;
#16292=DIRECTION ( 'NONE',  ( 0.000000000000000000, 0.000000000000000000, 1.000000000000000000 ) ) ;
#16295=VECTOR ( 'NONE', #11103, 1000.000000000000000 ) ;
#16311=LINE ( 'NONE', #22514, #13096 ) ;
#16324=EDGE_CURVE ( 'NONE', #40691, #35752, #25200, .T. ) ;
#16330=CARTESIAN_POINT ( 'NONE',  ( -40.24874870218063450, -26.64985754041175525, 6.700000000000000178 ) ) ;
#16343=CARTESIAN_POINT ( 'NONE',  ( 11.65737507970504439, -27.06993018339339940, 6.800000000000000711 ) ) ;
#16346=DIRECTION ( 'NONE',  ( 0.000000000000000000, 0.000000000000000000, -1.000000000000000000 ) ) ;
#16362=EDGE_CURVE ( 'NONE', #1149, #22787, #32996, .T. ) ;
#16365=ADVANCED_FACE ( 'NONE', ( #38750 ), #10352, .F. ) ;
#16371=EDGE_LOOP ( 'NONE', ( #28620, #24446, #4350, #28341 ) ) ;
#16374=EDGE_CURVE ( 'NONE', #28154, #18594, #26417, .T. ) ;
#16379=DIRECTION ( 'NONE',  ( -0.000000000000000000, -0.000000000000000000, 1.000000000000000000 ) ) ;
#16382=LINE ( 'NONE', #38004, #14967 ) ;
#16389=EDGE_CURVE ( 'NONE', #3169, #12201, #7667, .T. ) ;
#16390=FACE_OUTER_BOUND ( 'NONE', #20788, .T. ) ;
#16391=AXIS2_PLACEMENT_3D ( 'NONE', #40143, #23877, #4959 ) ;
#16393=CARTESIAN_POINT ( 'NONE',  ( -34.24874870218063450, -26.64985754041175525, 6.700000000000000178 ) ) ;
#16398=EDGE_LOOP ( 'NONE', ( #7811, #24296, #32303, #21465 ) ) ;
#16413=DIRECTION ( 'NONE',  ( -0.000000000000000000, -0.000000000000000000, -1.000000000000000000 ) ) ;
#16416=DIRECTION ( 'NONE',  ( -0.000000000000000000, -0.000000000000000000, -1.000000000000000000 ) ) ;
#16422=EDGE_LOOP ( 'NONE', ( #31533, #24631, #8415, #25710 ) ) ;
#16425=CARTESIAN_POINT ( 'NONE',  ( -23.07867591359219617, -24.55319635012989110, 6.800000000000000711 ) ) ;
#16426=ORIENTED_EDGE ( 'NONE', *, *, #36326, .T. ) ;
#16437=VECTOR ( 'NONE', #22612, 1000.000000000000000 ) ;
#16446=ORIENTED_EDGE ( 'NONE', *, *, #3312, .T. ) ;
#16447=EDGE_CURVE ( 'NONE', #14079, #10139, #10740, .T. ) ;
#16448=ORIENTED_EDGE ( 'NONE', *, *, #23470, .F. ) ;
#16451=VECTOR ( 'NONE', #30946, 1000.000000000000000 ) ;
#16462=EDGE_CURVE ( 'NONE', #4265, #10217, #39148, .T. ) ;
#16464=DIRECTION ( 'NONE',  ( -0.000000000000000000, -1.000000000000000000, -0.000000000000000000 ) ) ;
#16466=DIRECTION ( 'NONE',  ( -1.000000000000000000, 6.367278819747327815E-17, -0.000000000000000000 ) ) ;
#16468=CIRCLE ( 'NONE', #25038, 0.1000000000000028644 ) ;
#16476=DIRECTION ( 'NONE',  ( -0.000000000000000000, -1.000000000000000000, -0.000000000000000000 ) ) ;
#16477=ORIENTED_EDGE ( 'NONE', *, *, #33744, .T. ) ;
#16481=FACE_BOUND ( 'NONE', #25053, .T. ) ;
#16483=EDGE_LOOP ( 'NONE', ( #38141, #25771, #37865, #11792 ) ) ;
#16487=ORIENTED_EDGE ( 'NONE', *, *, #9843, .F. ) ;
#16500=LINE ( 'NONE', #38928, #18941 ) ;
#16502=ADVANCED_FACE ( 'NONE', ( #32204 ), #901, .F. ) ;
#16505=PLANE ( 'NONE',  #15085 ) ;
#16506=AXIS2_PLACEMENT_3D ( 'NONE', #25905, #1406, #16610 ) ;
#16515=DIRECTION ( 'NONE',  ( -0.000000000000000000, -0.000000000000000000, 1.000000000000000000 ) ) ;
#16520=CARTESIAN_POINT ( 'NONE',  ( -25.07867591359219617, -26.64985754041175525, 6.700000000000000178 ) ) ;
#16521=EDGE_LOOP ( 'NONE', ( #19191, #17665, #21197, #34531 ) ) ;
#16528=ORIENTED_EDGE ( 'NONE', *, *, #31297, .F. ) ;
#16540=ORIENTED_EDGE ( 'NONE', *, *, #38522, .F. ) ;
#16550=ORIENTED_EDGE ( 'NONE', *, *, #22056, .T. ) ;
#16551=DIRECTION ( 'NONE',  ( -0.000000000000000000, -0.000000000000000000, 1.000000000000000000 ) ) ;
#16559=CARTESIAN_POINT ( 'NONE',  ( -18.87867591359219333, -26.64985754041175525, 6.800000000000000711 ) ) ;
#16562=VERTEX_POINT ( 'NONE', #17513 ) ;
#16564=VECTOR ( 'NONE', #22679, 1000.000000000000000 ) ;
#16567=DIRECTION ( 'NONE',  ( 0.000000000000000000, 0.000000000000000000, -1.000000000000000000 ) ) ;
#16569=ORIENTED_EDGE ( 'NONE', *, *, #39786, .T. ) ;
#16576=EDGE_LOOP ( 'NONE', ( #4551, #8820, #11358, #1816 ) ) ;
#16588=LINE ( 'NONE', #29761, #1847 ) ;
#16598=CARTESIAN_POINT ( 'NONE',  ( -32.97867591359219119, -26.64985754041175525, 6.800000000000000711 ) ) ;
#16601=DIRECTION ( 'NONE',  ( -1.000000000000000000, 0.000000000000000000, 0.000000000000000000 ) ) ;
#16606=EDGE_CURVE ( 'NONE', #1810, #14763, #21242, .T. ) ;
#16607=DIRECTION ( 'NONE',  ( 1.000000000000000000, 0.000000000000000000, 0.000000000000000000 ) ) ;
#16610=DIRECTION ( 'NONE',  ( 1.000000000000000000, 0.000000000000000000, 0.000000000000000000 ) ) ;
#16612=( GEOMETRIC_REPRESENTATION_CONTEXT ( 3 ) GLOBAL_UNCERTAINTY_ASSIGNED_CONTEXT ( ( #9805 ) ) GLOBAL_UNIT_ASSIGNED_CONTEXT ( ( #32556, #16671, #28649 ) ) REPRESENTATION_CONTEXT ( 'NONE', 'WORKASPACE' ) );
#16617=ORIENTED_EDGE ( 'NONE', *, *, #2408, .F. ) ;
#16633=EDGE_LOOP ( 'NONE', ( #2027, #37004, #24, #11188 ) ) ;
#16635=VERTEX_POINT ( 'NONE', #2117 ) ;
#16637=ORIENTED_EDGE ( 'NONE', *, *, #36071, .F. ) ;
#16655=CIRCLE ( 'NONE', #2893, 0.1000000000000028644 ) ;
#16664=ORIENTED_EDGE ( 'NONE', *, *, #21151, .T. ) ;
#16668=DIRECTION ( 'NONE',  ( -0.000000000000000000, -0.000000000000000000, 1.000000000000000000 ) ) ;
#16671=( NAMED_UNIT ( * ) PLANE_ANGLE_UNIT ( ) SI_UNIT ( $, .RADIAN. ) );
#16673=EDGE_CURVE ( 'NONE', #36487, #39450, #4002, .T. ) ;
#16675=DIRECTION ( 'NONE',  ( -1.000000000000000000, 0.000000000000000000, 0.000000000000000000 ) ) ;
#16676=ORIENTED_EDGE ( 'NONE', *, *, #20970, .T. ) ;
#16683=CARTESIAN_POINT ( 'NONE',  ( -6.978675913592191193, -26.64985754041175525, 6.700000000000000178 ) ) ;
#16684=VECTOR ( 'NONE', #13040, 1000.000000000000000 ) ;
#16685=DIRECTION ( 'NONE',  ( 1.000000000000000000, 0.000000000000000000, 0.000000000000000000 ) ) ;
#16687=DIRECTION ( 'NONE',  ( 0.000000000000000000, 0.000000000000000000, 1.000000000000000000 ) ) ;
#16696=CARTESIAN_POINT ( 'NONE',  ( -24.97867591359219475, -26.64985754041175525, 6.700000000000000178 ) ) ;
#16698=AXIS2_PLACEMENT_3D ( 'NONE', #35260, #7029, #19598 ) ;
#16700=CARTESIAN_POINT ( 'NONE',  ( -20.44874870218064444, -26.64985754041175525, 6.700000000000000178 ) ) ;
#16703=CARTESIAN_POINT ( 'NONE',  ( -26.44874870218064089, -26.64985754041175525, 6.700000000000000178 ) ) ;
#16705=VERTEX_POINT ( 'NONE', #899 ) ;
#16709=FACE_OUTER_BOUND ( 'NONE', #18834, .T. ) ;
#16711=CIRCLE ( 'NONE', #16060, 0.1000000000000028644 ) ;
#16718=EDGE_CURVE ( 'NONE', #21616, #35240, #14710, .T. ) ;
#16725=DIRECTION ( 'NONE',  ( 1.000000000000000000, 0.000000000000000000, 0.000000000000000000 ) ) ;
#16733=ORIENTED_EDGE ( 'NONE', *, *, #24147, .T. ) ;
#16737=ORIENTED_EDGE ( 'NONE', *, *, #4744, .T. ) ;
#16738=ADVANCED_FACE ( 'NONE', ( #16709, #29300 ), #13644, .F. ) ;
#16741=ORIENTED_EDGE ( 'NONE', *, *, #23351, .F. ) ;
#16747=DIRECTION ( 'NONE',  ( 0.000000000000000000, 1.000000000000000000, 0.000000000000000000 ) ) ;
#16756=CARTESIAN_POINT ( 'NONE',  ( -40.24874870218063450, -26.64985754041175525, 6.700000000000000178 ) ) ;
#16757=VECTOR ( 'NONE', #38001, 1000.000000000000000 ) ;
#16766=CARTESIAN_POINT ( 'NONE',  ( -16.44874870218064089, -26.64985754041175525, 6.700000000000000178 ) ) ;
#16767=ORIENTED_EDGE ( 'NONE', *, *, #2109, .T. ) ;
#16775=AXIS2_PLACEMENT_3D ( 'NONE', #29827, #26749, #11076 ) ;
#16777=EDGE_CURVE ( 'NONE', #9686, #25800, #37730, .T. ) ;
#16802=ADVANCED_FACE ( 'NONE', ( #33613 ), #4984, .F. ) ;
#16803=AXIS2_PLACEMENT_3D ( 'NONE', #7546, #38427, #7345 ) ;
#16807=DIRECTION ( 'NONE',  ( 1.000000000000000000, 0.000000000000000000, 0.000000000000000000 ) ) ;
#16809=CARTESIAN_POINT ( 'NONE',  ( 4.921324086407802056, -26.64985754041175525, 6.700000000000000178 ) ) ;
#16813=EDGE_CURVE ( 'NONE', #1190, #1835, #2734, .T. ) ;
#16814=DIRECTION ( 'NONE',  ( 0.000000000000000000, 0.000000000000000000, 1.000000000000000000 ) ) ;
#16835=CIRCLE ( 'NONE', #6439, 0.1000000000000028644 ) ;
#16839=EDGE_LOOP ( 'NONE', ( #17788, #27158, #10014, #34587 ) ) ;
#16859=CARTESIAN_POINT ( 'NONE',  ( -24.34874870218063592, -25.49307895267003587, 6.800000000000000711 ) ) ;
#16870=AXIS2_PLACEMENT_3D ( 'NONE', #26790, #13617, #4961 ) ;
#16873=ORIENTED_EDGE ( 'NONE', *, *, #27737, .F. ) ;
#16879=ORIENTED_EDGE ( 'NONE', *, *, #10559, .F. ) ;
#16882=ORIENTED_EDGE ( 'NONE', *, *, #27126, .T. ) ;
#16885=FACE_OUTER_BOUND ( 'NONE', #2220, .T. ) ;
#16892=CARTESIAN_POINT ( 'NONE',  ( -30.34874870218063947, -26.64985754041175525, 6.700000000000000178 ) ) ;
#16898=AXIS2_PLACEMENT_3D ( 'NONE', #8104, #11797, #14493 ) ;
#16901=CARTESIAN_POINT ( 'NONE',  ( -36.24874870218063450, -26.64985754041175525, 6.700000000000000178 ) ) ;
#16906=FACE_OUTER_BOUND ( 'NONE', #13327, .T. ) ;
#16914=DIRECTION ( 'NONE',  ( -0.000000000000000000, -0.000000000000000000, 1.000000000000000000 ) ) ;
#16928=CIRCLE ( 'NONE', #2512, 0.1000000000000028644 ) ;
#16929=FACE_OUTER_BOUND ( 'NONE', #9563, .T. ) ;
#16932=DIRECTION ( 'NONE',  ( 1.000000000000000000, -6.367278819747329048E-17, 0.000000000000000000 ) ) ;
#16935=LINE ( 'NONE', #17326, #13377 ) ;
#16936=EDGE_LOOP ( 'NONE', ( #23089, #13782, #29001, #31458 ) ) ;
#16960=CARTESIAN_POINT ( 'NONE',  ( 1.651251297819358754, -26.64985754041175525, 6.700000000000000178 ) ) ;
#16962=LINE ( 'NONE', #29538, #5477 ) ;
#16966=DIRECTION ( 'NONE',  ( 0.000000000000000000, 1.000000000000000000, 0.000000000000000000 ) ) ;
#16967=EDGE_CURVE ( 'NONE', #16635, #9241, #17225, .T. ) ;
#16969=EDGE_LOOP ( 'NONE', ( #29156, #253, #38278, #2882 ) ) ;
#16980=FACE_OUTER_BOUND ( 'NONE', #33335, .T. ) ;
#16991=ORIENTED_EDGE ( 'NONE', *, *, #2170, .T. ) ;
#16992=DIRECTION ( 'NONE',  ( 0.000000000000000000, 0.000000000000000000, 1.000000000000000000 ) ) ;
#16993=CARTESIAN_POINT ( 'NONE',  ( -16.44874870218064089, -25.49307895267003587, 6.700000000000000178 ) ) ;
#16997=DIRECTION ( 'NONE',  ( 1.000000000000000000, 0.000000000000000000, -0.000000000000000000 ) ) ;
#16999=LINE ( 'NONE', #39428, #22921 ) ;
#17003=ADVANCED_FACE ( 'NONE', ( #1018 ), #35991, .F. ) ;
#17006=EDGE_CURVE ( 'NONE', #11338, #7017, #20321, .T. ) ;
#17008=CYLINDRICAL_SURFACE ( 'NONE', #32623, 0.1000000000000028644 ) ;
#17019=CARTESIAN_POINT ( 'NONE',  ( 7.121324086407810228, -24.55319635012989110, 6.700000000000000178 ) ) ;
#17020=VERTEX_POINT ( 'NONE', #10850 ) ;
#17021=CARTESIAN_POINT ( 'NONE',  ( -18.87867591359219333, -26.64985754041175525, 6.800000000000000711 ) ) ;
#17026=LINE ( 'NONE', #22834, #35221 ) ;
#17029=ORIENTED_EDGE ( 'NONE', *, *, #31768, .T. ) ;
#17032=DIRECTION ( 'NONE',  ( -0.000000000000000000, -0.000000000000000000, 1.000000000000000000 ) ) ;
#17037=VECTOR ( 'NONE', #4224, 1000.000000000000000 ) ;
#17053=EDGE_CURVE ( 'NONE', #37912, #25803, #35881, .T. ) ;
#17055=CARTESIAN_POINT ( 'NONE',  ( -0.3487487021806359722, -26.64985754041175525, 6.700000000000000178 ) ) ;
#17062=ORIENTED_EDGE ( 'NONE', *, *, #6333, .F. ) ;
#17067=CIRCLE ( 'NONE', #4610, 0.1000000000000028644 ) ;
#17073=EDGE_CURVE ( 'NONE', #1547, #2693, #26323, .T. ) ;
#17079=AXIS2_PLACEMENT_3D ( 'NONE', #40378, #8886, #31752 ) ;
#17090=EDGE_CURVE ( 'NONE', #32857, #26162, #32903, .T. ) ;
#17102=LINE ( 'NONE', #4379, #7283 ) ;
#17104=PLANE ( 'NONE',  #7857 ) ;
#17105=EDGE_CURVE ( 'NONE', #17630, #7892, #17026, .T. ) ;
#17109=CARTESIAN_POINT ( 'NONE',  ( -14.97867591359219119, -26.64985754041175525, 6.700000000000000178 ) ) ;
#17110=LINE ( 'NONE', #7659, #20424 ) ;
#17111=CIRCLE ( 'NONE', #19751, 0.1000000000000028644 ) ;
#17113=ORIENTED_EDGE ( 'NONE', *, *, #3762, .F. ) ;
#17115=DIRECTION ( 'NONE',  ( -0.000000000000000000, -0.000000000000000000, 1.000000000000000000 ) ) ;
#17128=CARTESIAN_POINT ( 'NONE',  ( -42.34874870218063592, -26.64985754041175525, 6.800000000000000711 ) ) ;
#17137=EDGE_CURVE ( 'NONE', #37233, #3771, #23230, .T. ) ;
#17146=DIRECTION ( 'NONE',  ( -0.000000000000000000, -0.000000000000000000, 1.000000000000000000 ) ) ;
#17157=DIRECTION ( 'NONE',  ( 1.000000000000000000, 0.000000000000000000, 0.000000000000000000 ) ) ;
#17160=FACE_OUTER_BOUND ( 'NONE', #18589, .T. ) ;
#17161=CIRCLE ( 'NONE', #22457, 0.1000000000000028644 ) ;
#17171=CYLINDRICAL_SURFACE ( 'NONE', #25892, 0.1000000000000028644 ) ;
#17177=CARTESIAN_POINT ( 'NONE',  ( -33.07867591359219972, -26.64985754041175525, 6.700000000000000178 ) ) ;
#17184=PLANE ( 'NONE',  #15117 ) ;
#17186=ADVANCED_FACE ( 'NONE', ( #25917 ), #35404, .F. ) ;
#17187=CARTESIAN_POINT ( 'NONE',  ( -28.24874870218063805, -26.64985754041175525, 6.700000000000000178 ) ) ;
#17194=VERTEX_POINT ( 'NONE', #23035 ) ;
#17196=VECTOR ( 'NONE', #22646, 1000.000000000000000 ) ;
#17208=LINE ( 'NONE', #29775, #40456 ) ;
#17212=CARTESIAN_POINT ( 'NONE',  ( -3.078675913592197944, -26.64985754041175525, 6.800000000000000711 ) ) ;
#17225=LINE ( 'NONE', #13952, #12853 ) ;
#17229=ORIENTED_EDGE ( 'NONE', *, *, #39407, .F. ) ;
#17233=EDGE_CURVE ( 'NONE', #40311, #23873, #8156, .T. ) ;
#17235=CARTESIAN_POINT ( 'NONE',  ( -54.01549048184568846, -38.28842912540938670, -4.152976064860135708 ) ) ;
#17244=DIRECTION ( 'NONE',  ( -0.000000000000000000, -0.000000000000000000, 1.000000000000000000 ) ) ;
#17247=CARTESIAN_POINT ( 'NONE',  ( -14.44874870218064089, -25.49307895267003587, 6.700000000000000178 ) ) ;
#17250=VERTEX_POINT ( 'NONE', #33313 ) ;
#17251=CARTESIAN_POINT ( 'NONE',  ( -36.24874870218063450, -25.49307895267003587, 6.800000000000000711 ) ) ;
#17255=CARTESIAN_POINT ( 'NONE',  ( -0.9786759135921931918, -26.64985754041175525, 6.800000000000000711 ) ) ;
#17260=LINE ( 'NONE', #3949, #35594 ) ;
#17263=ORIENTED_EDGE ( 'NONE', *, *, #12630, .F. ) ;
#17271=AXIS2_PLACEMENT_3D ( 'NONE', #6737, #28558, #37199 ) ;
#17273=DIRECTION ( 'NONE',  ( 1.000000000000000000, 0.000000000000000000, 0.000000000000000000 ) ) ;
#17281=DIRECTION ( 'NONE',  ( 0.000000000000000000, 0.000000000000000000, 1.000000000000000000 ) ) ;
#17283=DIRECTION ( 'NONE',  ( 1.000000000000000000, 0.000000000000000000, 0.000000000000000000 ) ) ;
#17285=CIRCLE ( 'NONE', #4165, 0.1000000000000028644 ) ;
#17287=CARTESIAN_POINT ( 'NONE',  ( 7.121324086407810228, -26.64985754041175525, 6.700000000000000178 ) ) ;
#17289=DIRECTION ( 'NONE',  ( -0.000000000000000000, -0.000000000000000000, 1.000000000000000000 ) ) ;
#17295=DIRECTION ( 'NONE',  ( 0.000000000000000000, 0.000000000000000000, 1.000000000000000000 ) ) ;
#17326=CARTESIAN_POINT ( 'NONE',  ( -14.87867591359218977, -24.55319635012989110, 6.700000000000000178 ) ) ;
#17337=DIRECTION ( 'NONE',  ( -0.000000000000000000, -0.000000000000000000, 1.000000000000000000 ) ) ;
#17343=EDGE_CURVE ( 'NONE', #29464, #5443, #36788, .T. ) ;
#17351=PLANE ( 'NONE',  #12039 ) ;
#17355=VECTOR ( 'NONE', #6080, 1000.000000000000000 ) ;
#17366=DIRECTION ( 'NONE',  ( -0.000000000000000000, -0.000000000000000000, 1.000000000000000000 ) ) ;
#17372=EDGE_CURVE ( 'NONE', #33264, #24867, #9810, .T. ) ;
#17381=AXIS2_PLACEMENT_3D ( 'NONE', #3641, #34932, #22965 ) ;
#17385=ORIENTED_EDGE ( 'NONE', *, *, #12472, .F. ) ;
#17397=ADVANCED_FACE ( 'NONE', ( #9391 ), #34759, .F. ) ;
#17399=EDGE_CURVE ( 'NONE', #826, #7900, #6534, .T. ) ;
#17406=VECTOR ( 'NONE', #11495, 1000.000000000000000 ) ;
#17412=ORIENTED_EDGE ( 'NONE', *, *, #38061, .T. ) ;
#17422=CARTESIAN_POINT ( 'NONE',  ( -21.07867591359219617, -26.64985754041175525, 6.700000000000000178 ) ) ;
#17426=CARTESIAN_POINT ( 'NONE',  ( -36.44874870218064444, -26.64985754041175525, 6.700000000000000178 ) ) ;
#17427=DIRECTION ( 'NONE',  ( 0.000000000000000000, 0.000000000000000000, 1.000000000000000000 ) ) ;
#17441=AXIS2_PLACEMENT_3D ( 'NONE', #24839, #21752, #37386 ) ;
#17451=EDGE_CURVE ( 'NONE', #4930, #17020, #8870, .T. ) ;
#17456=EDGE_LOOP ( 'NONE', ( #4521, #10603, #19950, #34596 ) ) ;
#17459=DIRECTION ( 'NONE',  ( 1.000000000000000000, 0.000000000000000000, 0.000000000000000000 ) ) ;
#17465=ORIENTED_EDGE ( 'NONE', *, *, #22520, .T. ) ;
#17471=ORIENTED_EDGE ( 'NONE', *, *, #1751, .T. ) ;
#17473=VECTOR ( 'NONE', #4175, 1000.000000000000000 ) ;
#17482=ORIENTED_EDGE ( 'NONE', *, *, #23971, .F. ) ;
#17492=LINE ( 'NONE', #36862, #6316 ) ;
#17499=FACE_OUTER_BOUND ( 'NONE', #3601, .T. ) ;
#17502=AXIS2_PLACEMENT_3D ( 'NONE', #15692, #69, #2552 ) ;
#17504=ADVANCED_FACE ( 'NONE', ( #37799 ), #25663, .F. ) ;
#17505=DIRECTION ( 'NONE',  ( 1.000000000000000000, 0.000000000000000000, -0.000000000000000000 ) ) ;
#17511=DIRECTION ( 'NONE',  ( -0.000000000000000000, -0.000000000000000000, 1.000000000000000000 ) ) ;
#17513=CARTESIAN_POINT ( 'NONE',  ( -30.87867591359218977, -26.64985754041175525, 6.800000000000000711 ) ) ;
#17522=AXIS2_PLACEMENT_3D ( 'NONE', #11619, #40050, #36159 ) ;
#17527=DIRECTION ( 'NONE',  ( -0.000000000000000000, -0.000000000000000000, 1.000000000000000000 ) ) ;
#17534=AXIS2_PLACEMENT_3D ( 'NONE', #32473, #3888, #38631 ) ;
#17543=CARTESIAN_POINT ( 'NONE',  ( -34.24874870218063450, -26.64985754041175525, 6.700000000000000178 ) ) ;
#17547=ADVANCED_FACE ( 'NONE', ( #8413 ), #20987, .F. ) ;
#17561=VERTEX_POINT ( 'NONE', #5544 ) ;
#17574=DIRECTION ( 'NONE',  ( 1.000000000000000000, 0.000000000000000000, 0.000000000000000000 ) ) ;
#17578=VECTOR ( 'NONE', #34155, 1000.000000000000000 ) ;
#17580=ADVANCED_FACE ( 'NONE', ( #27361 ), #27765, .T. ) ;
#17584=AXIS2_PLACEMENT_3D ( 'NONE', #31457, #16992, #26086 ) ;
#17587=EDGE_CURVE ( 'NONE', #12705, #29312, #17671, .T. ) ;
#17589=AXIS2_PLACEMENT_3D ( 'NONE', #26399, #10721, #35871 ) ;
#17592=EDGE_CURVE ( 'NONE', #8931, #4265, #5631, .T. ) ;
#17600=DIRECTION ( 'NONE',  ( 0.000000000000000000, 0.000000000000000000, 1.000000000000000000 ) ) ;
#17605=CARTESIAN_POINT ( 'NONE',  ( -9.078675913592196167, -26.64985754041175525, 6.700000000000000178 ) ) ;
#17607=ORIENTED_EDGE ( 'NONE', *, *, #33161, .F. ) ;
#17608=AXIS2_PLACEMENT_3D ( 'NONE', #26834, #36306, #36111 ) ;
#17611=ORIENTED_EDGE ( 'NONE', *, *, #6055, .T. ) ;
#17624=ORIENTED_EDGE ( 'NONE', *, *, #15363, .T. ) ;
#17630=VERTEX_POINT ( 'NONE', #26959 ) ;
#17632=DIRECTION ( 'NONE',  ( 1.000000000000000000, 0.000000000000000000, 0.000000000000000000 ) ) ;
#17633=VECTOR ( 'NONE', #31164, 1000.000000000000000 ) ;
#17642=FACE_OUTER_BOUND ( 'NONE', #30979, .T. ) ;
#17644=ORIENTED_EDGE ( 'NONE', *, *, #1049, .F. ) ;
#17647=ORIENTED_EDGE ( 'NONE', *, *, #36071, .T. ) ;
#17648=CARTESIAN_POINT ( 'NONE',  ( -8.878675913592189772, -26.64985754041175525, 6.700000000000000178 ) ) ;
#17663=AXIS2_PLACEMENT_3D ( 'NONE', #27535, #12288, #31048 ) ;
#17664=ORIENTED_EDGE ( 'NONE', *, *, #57, .T. ) ;
#17665=ORIENTED_EDGE ( 'NONE', *, *, #38813, .F. ) ;
#17667=CARTESIAN_POINT ( 'NONE',  ( -6.878675913592188884, -24.55319635012989110, 6.700000000000000178 ) ) ;
#17670=ORIENTED_EDGE ( 'NONE', *, *, #35777, .F. ) ;
#17671=LINE ( 'NONE', #11901, #17406 ) ;
#17674=DIRECTION ( 'NONE',  ( 1.000000000000000000, 0.000000000000000000, 0.000000000000000000 ) ) ;
#17675=CARTESIAN_POINT ( 'NONE',  ( -20.87867591359218977, -24.55319635012989110, 6.700000000000000178 ) ) ;
#17686=EDGE_CURVE ( 'NONE', #5705, #13694, #3017, .T. ) ;
#17690=LINE ( 'NONE', #24077, #10127 ) ;
#17695=ADVANCED_FACE ( 'NONE', ( #3706 ), #37234, .F. ) ;
#17696=CYLINDRICAL_SURFACE ( 'NONE', #38535, 0.1000000000000028644 ) ;
#17697=EDGE_CURVE ( 'NONE', #24389, #8458, #13501, .T. ) ;
#17709=CARTESIAN_POINT ( 'NONE',  ( -9.078675913592196167, -26.64985754041175525, 6.700000000000000178 ) ) ;
#17710=DIRECTION ( 'NONE',  ( 1.000000000000000000, 0.000000000000000000, 0.000000000000000000 ) ) ;
#17711=CARTESIAN_POINT ( 'NONE',  ( -2.248748702180634940, -25.49307895267003587, 6.700000000000000178 ) ) ;
#17712=VECTOR ( 'NONE', #40714, 1000.000000000000000 ) ;
#17713=CARTESIAN_POINT ( 'NONE',  ( -12.34874870218063947, -25.49307895267003587, 6.700000000000000178 ) ) ;
#17732=ORIENTED_EDGE ( 'NONE', *, *, #3489, .F. ) ;
#17737=DIRECTION ( 'NONE',  ( 0.000000000000000000, 0.000000000000000000, 1.000000000000000000 ) ) ;
#17739=EDGE_LOOP ( 'NONE', ( #21770, #28097, #29564, #15323 ) ) ;
#17741=EDGE_CURVE ( 'NONE', #19582, #32758, #16228, .T. ) ;
#17745=EDGE_CURVE ( 'NONE', #7170, #33227, #25101, .T. ) ;
#17767=DIRECTION ( 'NONE',  ( 1.000000000000000000, 0.000000000000000000, 0.000000000000000000 ) ) ;
#17770=VERTEX_POINT ( 'NONE', #31688 ) ;
#17774=AXIS2_PLACEMENT_3D ( 'NONE', #4391, #38741, #14028 ) ;
#17776=CARTESIAN_POINT ( 'NONE',  ( -1.078675913592196167, -26.64985754041175525, 6.700000000000000178 ) ) ;
#17777=LINE ( 'NONE', #39609, #40328 ) ;
#17778=CARTESIAN_POINT ( 'NONE',  ( -0.2487487021806331078, -26.64985754041175525, 6.700000000000000178 ) ) ;
#17782=CARTESIAN_POINT ( 'NONE',  ( -34.44874870218064444, -26.64985754041175525, 6.700000000000000178 ) ) ;
#17785=CARTESIAN_POINT ( 'NONE',  ( -6.878675913592188884, -26.64985754041175525, 6.800000000000000711 ) ) ;
#17788=ORIENTED_EDGE ( 'NONE', *, *, #35018, .T. ) ;
#17795=ADVANCED_FACE ( 'NONE', ( #3504 ), #16026, .T. ) ;
#17808=DIRECTION ( 'NONE',  ( -0.000000000000000000, -1.000000000000000000, -0.000000000000000000 ) ) ;
#17809=VECTOR ( 'NONE', #4517, 1000.000000000000000 ) ;
#17811=FACE_OUTER_BOUND ( 'NONE', #31715, .T. ) ;
#17813=AXIS2_PLACEMENT_3D ( 'NONE', #5798, #8865, #14632 ) ;
#17826=DIRECTION ( 'NONE',  ( -0.000000000000000000, -0.000000000000000000, 1.000000000000000000 ) ) ;
#17829=EDGE_CURVE ( 'NONE', #21972, #2270, #4978, .T. ) ;
#17830=ORIENTED_EDGE ( 'NONE', *, *, #40093, .F. ) ;
#17832=DIRECTION ( 'NONE',  ( -0.000000000000000000, -0.000000000000000000, 1.000000000000000000 ) ) ;
#17836=ORIENTED_EDGE ( 'NONE', *, *, #5642, .T. ) ;
#17838=VECTOR ( 'NONE', #19743, 1000.000000000000000 ) ;
#17840=EDGE_CURVE ( 'NONE', #33660, #3598, #29000, .T. ) ;
#17842=LINE ( 'NONE', #26922, #1927 ) ;
#17844=CYLINDRICAL_SURFACE ( 'NONE', #511, 0.1000000000000028644 ) ;
#17847=ORIENTED_EDGE ( 'NONE', *, *, #29714, .F. ) ;
#17851=DIRECTION ( 'NONE',  ( 0.000000000000000000, 1.000000000000000000, 0.000000000000000000 ) ) ;
#17852=CARTESIAN_POINT ( 'NONE',  ( -2.348748702180637693, -26.64985754041175525, 6.700000000000000178 ) ) ;
#17858=ADVANCED_FACE ( 'NONE', ( #10049 ), #32110, .F. ) ;
#17869=EDGE_LOOP ( 'NONE', ( #20856, #14187, #14391, #16446 ) ) ;
#17873=ADVANCED_FACE ( 'NONE', ( #25707 ), #1220, .F. ) ;
#17874=ADVANCED_FACE ( 'NONE', ( #1412 ), #26118, .F. ) ;
#17876=AXIS2_PLACEMENT_3D ( 'NONE', #12573, #21449, #34025 ) ;
#17877=CARTESIAN_POINT ( 'NONE',  ( 1.751251297819361730, -26.64985754041175525, 6.700000000000000178 ) ) ;
#17879=ADVANCED_FACE ( 'NONE', ( #35198 ), #38445, .F. ) ;
#17882=EDGE_LOOP ( 'NONE', ( #21980, #16741, #6132, #12234 ) ) ;
#17886=LINE ( 'NONE', #24280, #20774 ) ;
#17887=EDGE_LOOP ( 'NONE', ( #16879, #13492, #25966, #15649 ) ) ;
#17894=VERTEX_POINT ( 'NONE', #10646 ) ;
#17910=CIRCLE ( 'NONE', #19260, 0.1000000000000028644 ) ;
#17917=LINE ( 'NONE', #2307, #31217 ) ;
#17922=EDGE_CURVE ( 'NONE', #13813, #5244, #10249, .T. ) ;
#17923=VERTEX_POINT ( 'NONE', #35399 ) ;
#17932=DIRECTION ( 'NONE',  ( -0.000000000000000000, -1.000000000000000000, -0.000000000000000000 ) ) ;
#17934=CARTESIAN_POINT ( 'NONE',  ( -38.34874870218063592, -26.64985754041175525, 6.700000000000000178 ) ) ;
#17935=LINE ( 'NONE', #21661, #33949 ) ;
#17936=AXIS2_PLACEMENT_3D ( 'NONE', #36004, #23819, #13767 ) ;
#17943=EDGE_LOOP ( 'NONE', ( #37953, #28553, #26013, #3052 ) ) ;
#17949=VECTOR ( 'NONE', #24990, 1000.000000000000000 ) ;
#17955=VERTEX_POINT ( 'NONE', #10447 ) ;
#17957=CARTESIAN_POINT ( 'NONE',  ( -24.87867591359218977, -26.64985754041175525, 6.700000000000000178 ) ) ;
#17958=CARTESIAN_POINT ( 'NONE',  ( 5.651251297819362307, -26.64985754041175525, 6.800000000000000711 ) ) ;
#17985=LINE ( 'NONE', #18190, #1578 ) ;
#17988=CARTESIAN_POINT ( 'NONE',  ( -20.44874870218064444, -26.64985754041175525, 6.800000000000000711 ) ) ;
#17991=PRODUCT_CONTEXT ( 'NONE', #12393, 'mechanical' ) ;
#17994=DIRECTION ( 'NONE',  ( -1.000000000000000000, 0.000000000000000000, 0.000000000000000000 ) ) ;
#17999=EDGE_CURVE ( 'NONE', #37105, #33136, #40226, .T. ) ;
#18003=PLANE ( 'NONE',  #23833 ) ;
#18006=VERTEX_POINT ( 'NONE', #31184 ) ;
#18010=AXIS2_PLACEMENT_3D ( 'NONE', #37077, #2529, #1914 ) ;
#18013=CARTESIAN_POINT ( 'NONE',  ( -20.97867591359219475, -24.55319635012989110, 6.700000000000000178 ) ) ;
#18014=CARTESIAN_POINT ( 'NONE',  ( -10.24874870218063450, -26.64985754041175525, 6.800000000000000711 ) ) ;
#18024=CIRCLE ( 'NONE', #308, 0.1000000000000028644 ) ;
#18028=ADVANCED_FACE ( 'NONE', ( #3005 ), #28077, .F. ) ;
#18030=EDGE_CURVE ( 'NONE', #1346, #19329, #24032, .T. ) ;
#18031=DIRECTION ( 'NONE',  ( 0.000000000000000000, 0.000000000000000000, 1.000000000000000000 ) ) ;
#18033=CARTESIAN_POINT ( 'NONE',  ( -30.97867591359219119, -24.55319635012989110, 6.700000000000000178 ) ) ;
#18034=FACE_OUTER_BOUND ( 'NONE', #13963, .T. ) ;
#18036=ORIENTED_EDGE ( 'NONE', *, *, #38628, .F. ) ;
#18037=DIRECTION ( 'NONE',  ( 0.000000000000000000, 0.000000000000000000, 1.000000000000000000 ) ) ;
#18045=CIRCLE ( 'NONE', #40415, 0.1000000000000028644 ) ;
#18050=DIRECTION ( 'NONE',  ( 1.000000000000000000, 0.000000000000000000, 0.000000000000000000 ) ) ;
#18067=VECTOR ( 'NONE', #33739, 1000.000000000000000 ) ;
#18068=LINE ( 'NONE', #31471, #17712 ) ;
#18072=AXIS2_PLACEMENT_3D ( 'NONE', #14279, #26848, #11180 ) ;
#18093=ORIENTED_EDGE ( 'NONE', *, *, #33744, .F. ) ;
#18095=VECTOR ( 'NONE', #16416, 1000.000000000000000 ) ;
#18099=DIRECTION ( 'NONE',  ( 0.000000000000000000, 0.000000000000000000, 1.000000000000000000 ) ) ;
#18106=PLANE ( 'NONE',  #14414 ) ;
#18107=ORIENTED_EDGE ( 'NONE', *, *, #23161, .T. ) ;
#18121=DIRECTION ( 'NONE',  ( 0.000000000000000000, 0.000000000000000000, 1.000000000000000000 ) ) ;
#18138=DIRECTION ( 'NONE',  ( 0.000000000000000000, 1.000000000000000000, 0.000000000000000000 ) ) ;
#18142=CYLINDRICAL_SURFACE ( 'NONE', #26670, 6.781342077912186461 ) ;
#18143=DIRECTION ( 'NONE',  ( 0.000000000000000000, 1.000000000000000000, 0.000000000000000000 ) ) ;
#18150=ORIENTED_EDGE ( 'NONE', *, *, #30697, .F. ) ;
#18152=APPLICATION_CONTEXT ( 'automotive_design' ) ;
#18154=DIRECTION ( 'NONE',  ( 0.000000000000000000, -1.000000000000000000, 0.000000000000000000 ) ) ;
#18158=CYLINDRICAL_SURFACE ( 'NONE', #6989, 0.1000000000000028644 ) ;
#18164=ADVANCED_FACE ( 'NONE', ( #30112 ), #10947, .F. ) ;
#18166=DIRECTION ( 'NONE',  ( 1.000000000000000000, 0.000000000000000000, 0.000000000000000000 ) ) ;
#18168=VECTOR ( 'NONE', #10820, 1000.000000000000000 ) ;
#18171=LINE ( 'NONE', #36919, #6656 ) ;
#18175=DIRECTION ( 'NONE',  ( 0.000000000000000000, 0.000000000000000000, 1.000000000000000000 ) ) ;
#18179=LINE ( 'NONE', #12419, #17949 ) ;
#18183=CYLINDRICAL_SURFACE ( 'NONE', #25706, 0.1000000000000028644 ) ;
#18185=ORIENTED_EDGE ( 'NONE', *, *, #2596, .F. ) ;
#18188=AXIS2_PLACEMENT_3D ( 'NONE', #17934, #5601, #37083 ) ;
#18190=CARTESIAN_POINT ( 'NONE',  ( -33.07867591359219972, -26.64985754041175525, 6.800000000000000711 ) ) ;
#18191=DIRECTION ( 'NONE',  ( 1.000000000000000000, 0.000000000000000000, -0.000000000000000000 ) ) ;
#18195=AXIS2_PLACEMENT_3D ( 'NONE', #24151, #15295, #33752 ) ;
#18199=EDGE_LOOP ( 'NONE', ( #18668, #21376, #27477, #3498 ) ) ;
#18208=CARTESIAN_POINT ( 'NONE',  ( -30.44874870218064089, -26.64985754041175525, 6.700000000000000178 ) ) ;
#18209=EDGE_CURVE ( 'NONE', #2951, #35983, #29506, .T. ) ;
#18212=ORIENTED_EDGE ( 'NONE', *, *, #38628, .T. ) ;
#18222=DIRECTION ( 'NONE',  ( -0.000000000000000000, -0.000000000000000000, 1.000000000000000000 ) ) ;
#18225=CARTESIAN_POINT ( 'NONE',  ( -8.878675913592189772, -24.55319635012989110, 6.700000000000000178 ) ) ;
#18226=CIRCLE ( 'NONE', #20198, 0.1000000000000028644 ) ;
#18227=AXIS2_PLACEMENT_3D ( 'NONE', #24425, #18443, #8970 ) ;
#18231=VERTEX_POINT ( 'NONE', #2535 ) ;
#18254=CARTESIAN_POINT ( 'NONE',  ( -6.248748702180631831, -26.64985754041175525, 6.700000000000000178 ) ) ;
#18260=CARTESIAN_POINT ( 'NONE',  ( -14.97867591359219119, -26.64985754041175525, 6.700000000000000178 ) ) ;
#18261=ADVANCED_FACE ( 'NONE', ( #6011 ), #18142, .T. ) ;
#18262=EDGE_CURVE ( 'NONE', #6408, #22775, #14834, .T. ) ;
#18270=PLANE ( 'NONE',  #8903 ) ;
#18272=AXIS2_PLACEMENT_3D ( 'NONE', #38034, #22411, #13128 ) ;
#18275=CARTESIAN_POINT ( 'NONE',  ( -54.01549048184568846, -30.38627270959228710, 4.800000000000000711 ) ) ;
#18276=DIRECTION ( 'NONE',  ( 1.000000000000000000, -0.000000000000000000, 0.000000000000000000 ) ) ;
#18278=EDGE_LOOP ( 'NONE', ( #33574, #38268, #21850, #6970 ) ) ;
#18280=AXIS2_PLACEMENT_3D ( 'NONE', #19997, #28670, #13412 ) ;
#18281=CARTESIAN_POINT ( 'NONE',  ( 5.121324086407808451, -26.64985754041175525, 6.700000000000000178 ) ) ;
#18289=DIRECTION ( 'NONE',  ( 1.000000000000000000, 0.000000000000000000, 0.000000000000000000 ) ) ;
#18297=DIRECTION ( 'NONE',  ( 1.000000000000000000, 0.000000000000000000, 0.000000000000000000 ) ) ;
#18298=ORIENTED_EDGE ( 'NONE', *, *, #30031, .T. ) ;
#18306=FACE_OUTER_BOUND ( 'NONE', #28015, .T. ) ;
#18314=ADVANCED_FACE ( 'NONE', ( #11749 ), #27618, .F. ) ;
#18315=VERTEX_POINT ( 'NONE', #33620 ) ;
#18318=DIRECTION ( 'NONE',  ( 1.000000000000000000, -0.000000000000000000, 0.000000000000000000 ) ) ;
#18323=AXIS2_PLACEMENT_3D ( 'NONE', #9246, #24704, #21621 ) ;
#18337=VECTOR ( 'NONE', #26447, 1000.000000000000000 ) ;
#18339=VERTEX_POINT ( 'NONE', #27414 ) ;
#18342=CARTESIAN_POINT ( 'NONE',  ( -30.44874870218064089, -26.64985754041175525, 6.700000000000000178 ) ) ;
#18344=ORIENTED_EDGE ( 'NONE', *, *, #21958, .T. ) ;
#18358=CARTESIAN_POINT ( 'NONE',  ( -42.44874870218064444, -26.64985754041175525, 6.700000000000000178 ) ) ;
#18363=VERTEX_POINT ( 'NONE', #37086 ) ;
#18366=ADVANCED_FACE ( 'NONE', ( #9084 ), #39977, .F. ) ;
#18371=CARTESIAN_POINT ( 'NONE',  ( -23.07867591359219617, -24.55319635012989110, 6.700000000000000178 ) ) ;
#18372=FACE_OUTER_BOUND ( 'NONE', #6729, .T. ) ;
#18378=DIRECTION ( 'NONE',  ( -1.000000000000000000, 0.000000000000000000, 0.000000000000000000 ) ) ;
#18388=EDGE_CURVE ( 'NONE', #28508, #9457, #24326, .T. ) ;
#18391=VECTOR ( 'NONE', #8226, 1000.000000000000000 ) ;
#18392=EDGE_LOOP ( 'NONE', ( #27040, #39921, #17732, #8011 ) ) ;
#18393=CARTESIAN_POINT ( 'NONE',  ( -19.07867591359219972, -26.64985754041175525, 6.800000000000000711 ) ) ;
#18400=EDGE_CURVE ( 'NONE', #29312, #21972, #15264, .T. ) ;
#18404=ORIENTED_EDGE ( 'NONE', *, *, #33263, .T. ) ;
#18426=DIRECTION ( 'NONE',  ( -0.000000000000000000, -0.000000000000000000, 1.000000000000000000 ) ) ;
#18430=EDGE_CURVE ( 'NONE', #16055, #23873, #40367, .T. ) ;
#18438=EDGE_CURVE ( 'NONE', #34397, #6604, #17935, .T. ) ;
#18441=EDGE_CURVE ( 'NONE', #3524, #744, #5604, .T. ) ;
#18443=DIRECTION ( 'NONE',  ( 0.000000000000000000, 0.000000000000000000, 1.000000000000000000 ) ) ;
#18448=ADVANCED_FACE ( 'NONE', ( #6629, #52, #28648, #3962, #35250, #456, #16481, #10100, #15677, #6420, #13197, #28225, #38103, #21861, #25765, #29053, #9488, #861, #3159, #12994, #6215, #7020, #22685, #25967, #22484, #31951, #34852, #19588, #34436, #22074, #13393, #12582, #25559, #18760, #25148, #9905, #35050, #37683, #32164, #31335, #31740, #34649, #18976, #9282, #31540, #15879, #3757, #28437, #245, #6826, #12783, #25358 ), #37896, .T. ) ;
#18449=EDGE_LOOP ( 'NONE', ( #30114, #28287, #31147, #605 ) ) ;
#18450=DIRECTION ( 'NONE',  ( 1.000000000000000000, 0.000000000000000000, 0.000000000000000000 ) ) ;
#18452=EDGE_LOOP ( 'NONE', ( #11257, #14093, #13358, #35623 ) ) ;
#18453=ORIENTED_EDGE ( 'NONE', *, *, #15482, .T. ) ;
#18459=AXIS2_PLACEMENT_3D ( 'NONE', #39139, #20604, #32593 ) ;
#18462=FACE_OUTER_BOUND ( 'NONE', #21428, .T. ) ;
#18474=ORIENTED_EDGE ( 'NONE', *, *, #34982, .F. ) ;
#18484=ORIENTED_EDGE ( 'NONE', *, *, #28132, .T. ) ;
#18491=EDGE_CURVE ( 'NONE', #14653, #12843, #16082, .T. ) ;
#18497=VERTEX_POINT ( 'NONE', #39103 ) ;
#18503=ORIENTED_EDGE ( 'NONE', *, *, #31024, .T. ) ;
#18506=ORIENTED_EDGE ( 'NONE', *, *, #25251, .T. ) ;
#18509=CARTESIAN_POINT ( 'NONE',  ( 5.751251297819365504, -26.64985754041175525, 6.700000000000000178 ) ) ;
#18518=CARTESIAN_POINT ( 'NONE',  ( 0.9213240864078056092, -26.64985754041175525, 6.700000000000000178 ) ) ;
#18519=VERTEX_POINT ( 'NONE', #13806 ) ;
#18533=CIRCLE ( 'NONE', #19227, 0.1000000000000028644 ) ;
#18534=DIRECTION ( 'NONE',  ( 0.000000000000000000, 0.000000000000000000, 1.000000000000000000 ) ) ;
#18536=EDGE_LOOP ( 'NONE', ( #13045, #21530, #14338, #6643 ) ) ;
#18539=PLANE ( 'NONE',  #813 ) ;
#18547=DIRECTION ( 'NONE',  ( 1.000000000000000000, 0.000000000000000000, 0.000000000000000000 ) ) ;
#18557=LINE ( 'NONE', #256, #1345 ) ;
#18570=DIRECTION ( 'NONE',  ( 1.000000000000000000, 0.000000000000000000, 0.000000000000000000 ) ) ;
#18571=PLANE ( 'NONE',  #24608 ) ;
#18577=CARTESIAN_POINT ( 'NONE',  ( -38.44874870218063734, -25.49307895267003587, 6.700000000000000178 ) ) ;
#18583=CARTESIAN_POINT ( 'NONE',  ( -35.07867591359219972, -26.64985754041175525, 6.700000000000000178 ) ) ;
#18585=LINE ( 'NONE', #15305, #7044 ) ;
#18589=EDGE_LOOP ( 'NONE', ( #2312, #8767, #2420, #7022 ) ) ;
#18593=VECTOR ( 'NONE', #21862, 1000.000000000000000 ) ;
#18594=VERTEX_POINT ( 'NONE', #1461 ) ;
#18595=DIRECTION ( 'NONE',  ( 0.000000000000000000, 0.000000000000000000, 1.000000000000000000 ) ) ;
#18603=DIRECTION ( 'NONE',  ( 0.000000000000000000, 0.000000000000000000, 1.000000000000000000 ) ) ;
#18615=CARTESIAN_POINT ( 'NONE',  ( -31.07867591359219617, -24.55319635012989110, 6.700000000000000178 ) ) ;
#18627=EDGE_CURVE ( 'NONE', #18363, #23072, #12232, .T. ) ;
#18630=EDGE_CURVE ( 'NONE', #35146, #16635, #17886, .T. ) ;
#18637=VERTEX_POINT ( 'NONE', #36840 ) ;
#18642=DIRECTION ( 'NONE',  ( 1.000000000000000000, 0.000000000000000000, 0.000000000000000000 ) ) ;
#18645=DIRECTION ( 'NONE',  ( 0.000000000000000000, 0.000000000000000000, 1.000000000000000000 ) ) ;
#18646=CARTESIAN_POINT ( 'NONE',  ( -38.44874870218063734, -25.49307895267003587, 6.700000000000000178 ) ) ;
#18657=CARTESIAN_POINT ( 'NONE',  ( -28.97867591359219475, -26.64985754041175525, 6.700000000000000178 ) ) ;
#18661=VECTOR ( 'NONE', #26178, 1000.000000000000000 ) ;
#18664=CYLINDRICAL_SURFACE ( 'NONE', #17663, 0.1000000000000028644 ) ;
#18668=ORIENTED_EDGE ( 'NONE', *, *, #22195, .T. ) ;
#18671=VECTOR ( 'NONE', #18138, 1000.000000000000000 ) ;
#18680=LINE ( 'NONE', #15810, #23349 ) ;
#18681=ORIENTED_EDGE ( 'NONE', *, *, #17451, .T. ) ;
#18690=ORIENTED_EDGE ( 'NONE', *, *, #14563, .F. ) ;
#18702=EDGE_LOOP ( 'NONE', ( #37786, #25820, #20557, #13265 ) ) ;
#18709=ORIENTED_EDGE ( 'NONE', *, *, #17840, .F. ) ;
#18715=ADVANCED_FACE ( 'NONE', ( #3713 ), #31694, .F. ) ;
#18716=CARTESIAN_POINT ( 'NONE',  ( -0.9786759135921931918, -24.55319635012989110, 6.700000000000000178 ) ) ;
#18717=DIRECTION ( 'NONE',  ( 0.000000000000000000, 0.000000000000000000, 1.000000000000000000 ) ) ;
#18718=CARTESIAN_POINT ( 'NONE',  ( -10.97867591359219475, -26.64985754041175525, 6.700000000000000178 ) ) ;
#18732=VECTOR ( 'NONE', #4041, 1000.000000000000000 ) ;
#18745=DIRECTION ( 'NONE',  ( 0.000000000000000000, 0.000000000000000000, 1.000000000000000000 ) ) ;
#18748=EDGE_LOOP ( 'NONE', ( #6372, #29253, #12428, #12155 ) ) ;
#18755=VECTOR ( 'NONE', #31244, 1000.000000000000000 ) ;
#18760=FACE_BOUND ( 'NONE', #25429, .T. ) ;
#18764=VECTOR ( 'NONE', #20713, 1000.000000000000000 ) ;
#18771=CARTESIAN_POINT ( 'NONE',  ( -26.24874870218063450, -26.64985754041175525, 6.700000000000000178 ) ) ;
#18783=DIRECTION ( 'NONE',  ( 0.000000000000000000, 1.000000000000000000, 0.000000000000000000 ) ) ;
#18790=AXIS2_PLACEMENT_3D ( 'NONE', #4686, #4101, #4298 ) ;
#18795=CARTESIAN_POINT ( 'NONE',  ( -38.24874870218063450, -26.64985754041175525, 6.700000000000000178 ) ) ;
#18798=PLANE ( 'NONE',  #33204 ) ;
#18801=DIRECTION ( 'NONE',  ( 0.000000000000000000, 0.000000000000000000, 1.000000000000000000 ) ) ;
#18802=DIRECTION ( 'NONE',  ( -0.000000000000000000, -0.000000000000000000, 1.000000000000000000 ) ) ;
#18807=EDGE_LOOP ( 'NONE', ( #10853, #6653, #19114, #23419 ) ) ;
#18818=DIRECTION ( 'NONE',  ( -0.000000000000000000, -0.000000000000000000, 1.000000000000000000 ) ) ;
#18828=AXIS2_PLACEMENT_3D ( 'NONE', #10711, #14211, #11113 ) ;
#18833=DIRECTION ( 'NONE',  ( 1.000000000000000000, 0.000000000000000000, 0.000000000000000000 ) ) ;
#18834=EDGE_LOOP ( 'NONE', ( #11278, #662, #15125, #15160, #37685, #3126 ) ) ;
#18837=EDGE_LOOP ( 'NONE', ( #6686, #23279, #8636, #15881 ) ) ;
#18838=CARTESIAN_POINT ( 'NONE',  ( -52.01549048184568846, -38.28842912540938670, 6.800000000000000711 ) ) ;
#18841=CARTESIAN_POINT ( 'NONE',  ( -37.07867591359219261, -24.55319635012989110, 6.700000000000000178 ) ) ;
#18846=LINE ( 'NONE', #15553, #39165 ) ;
#18848=PLANE ( 'NONE',  #28956 ) ;
#18853=EDGE_LOOP ( 'NONE', ( #39790, #3410, #1497, #31814 ) ) ;
#18857=CIRCLE ( 'NONE', #25448, 0.1000000000000028644 ) ;
#18859=DIRECTION ( 'NONE',  ( 1.000000000000000000, -0.000000000000000000, -0.000000000000000000 ) ) ;
#18862=ORIENTED_EDGE ( 'NONE', *, *, #5073, .F. ) ;
#18867=DIRECTION ( 'NONE',  ( -1.000000000000000000, 0.000000000000000000, -0.000000000000000000 ) ) ;
#18870=ORIENTED_EDGE ( 'NONE', *, *, #34462, .F. ) ;
#18875=CARTESIAN_POINT ( 'NONE',  ( -2.248748702180634940, -26.64985754041175525, 6.700000000000000178 ) ) ;
#18881=DIRECTION ( 'NONE',  ( -1.000000000000000000, 0.000000000000000000, 0.000000000000000000 ) ) ;
#18884=FACE_OUTER_BOUND ( 'NONE', #26632, .T. ) ;
#18888=PLANE ( 'NONE',  #17584 ) ;
#18890=ORIENTED_EDGE ( 'NONE', *, *, #11134, .T. ) ;
#18899=ORIENTED_EDGE ( 'NONE', *, *, #26499, .F. ) ;
#18900=DIRECTION ( 'NONE',  ( 0.000000000000000000, 1.000000000000000000, 0.000000000000000000 ) ) ;
#18905=PLANE ( 'NONE',  #4320 ) ;
#18908=EDGE_CURVE ( 'NONE', #18951, #1190, #31243, .T. ) ;
#18914=FACE_OUTER_BOUND ( 'NONE', #28326, .T. ) ;
#18915=VECTOR ( 'NONE', #22669, 1000.000000000000000 ) ;
#18916=AXIS2_PLACEMENT_3D ( 'NONE', #25659, #9600, #34754 ) ;
#18920=LINE ( 'NONE', #17021, #13627 ) ;
#18933=DIRECTION ( 'NONE',  ( -1.000000000000000000, 0.000000000000000000, 0.000000000000000000 ) ) ;
#18938=VERTEX_POINT ( 'NONE', #30815 ) ;
#18941=VECTOR ( 'NONE', #1091, 1000.000000000000000 ) ;
#18949=CIRCLE ( 'NONE', #24193, 0.1000000000000028644 ) ;
#18951=VERTEX_POINT ( 'NONE', #27695 ) ;
#18959=EDGE_LOOP ( 'NONE', ( #29748, #3815, #36388, #33622 ) ) ;
#18962=VECTOR ( 'NONE', #16106, 1000.000000000000000 ) ;
#18965=ADVANCED_FACE ( 'NONE', ( #21540 ), #12037, .F. ) ;
#18975=ORIENTED_EDGE ( 'NONE', *, *, #9733, .T. ) ;
#18976=FACE_BOUND ( 'NONE', #21422, .T. ) ;
#18980=EDGE_CURVE ( 'NONE', #17250, #39647, #6927, .T. ) ;
#18993=ORIENTED_EDGE ( 'NONE', *, *, #29895, .F. ) ;
#18994=DIRECTION ( 'NONE',  ( 0.000000000000000000, 0.000000000000000000, 1.000000000000000000 ) ) ;
#18995=AXIS2_PLACEMENT_3D ( 'NONE', #8906, #5224, #21490 ) ;
#19003=CARTESIAN_POINT ( 'NONE',  ( -8.878675913592189772, -26.64985754041175525, 6.700000000000000178 ) ) ;
#19005=PLANE ( 'NONE',  #26125 ) ;
#19007=DIRECTION ( 'NONE',  ( -0.000000000000000000, -1.000000000000000000, -0.000000000000000000 ) ) ;
#19008=CARTESIAN_POINT ( 'NONE',  ( -22.87867591359218977, -26.64985754041175525, 6.800000000000000711 ) ) ;
#19022=EDGE_LOOP ( 'NONE', ( #825, #6827, #8327, #3615 ) ) ;
#19032=EDGE_CURVE ( 'NONE', #25414, #40311, #20687, .T. ) ;
#19050=LINE ( 'NONE', #31819, #33397 ) ;
#19052=VECTOR ( 'NONE', #31970, 1000.000000000000000 ) ;
#19059=DIRECTION ( 'NONE',  ( 0.000000000000000000, 1.000000000000000000, 0.000000000000000000 ) ) ;
#19060=CARTESIAN_POINT ( 'NONE',  ( 3.551251297819357777, -25.49307895267003587, 6.700000000000000178 ) ) ;
#19067=AXIS2_PLACEMENT_3D ( 'NONE', #18657, #28138, #25062 ) ;
#19071=EDGE_LOOP ( 'NONE', ( #9238, #6821, #10446, #2275 ) ) ;
#19073=LINE ( 'NONE', #6317, #32479 ) ;
#19078=EDGE_CURVE ( 'NONE', #3677, #4425, #22769, .T. ) ;
#19079=VERTEX_POINT ( 'NONE', #19861 ) ;
#19081=DIRECTION ( 'NONE',  ( -0.000000000000000000, -1.000000000000000000, -0.000000000000000000 ) ) ;
#19084=EDGE_LOOP ( 'NONE', ( #21350, #2710, #17830, #39510 ) ) ;
#19085=CARTESIAN_POINT ( 'NONE',  ( -40.24874870218063450, -26.64985754041175525, 6.800000000000000711 ) ) ;
#19087=CARTESIAN_POINT ( 'NONE',  ( -30.87867591359218977, -24.55319635012989110, 6.800000000000000711 ) ) ;
#19090=EDGE_LOOP ( 'NONE', ( #31783, #9996, #19555, #25897 ) ) ;
#19095=LINE ( 'NONE', #22403, #20336 ) ;
#19104=ADVANCED_FACE ( 'NONE', ( #35530 ), #13078, .F. ) ;
#19114=ORIENTED_EDGE ( 'NONE', *, *, #14221, .T. ) ;
#19119=ORIENTED_EDGE ( 'NONE', *, *, #30973, .F. ) ;
#19120=DIRECTION ( 'NONE',  ( 1.000000000000000000, 0.000000000000000000, 0.000000000000000000 ) ) ;
#19129=FACE_OUTER_BOUND ( 'NONE', #37096, .T. ) ;
#19131=ORIENTED_EDGE ( 'NONE', *, *, #4869, .T. ) ;
#19136=CARTESIAN_POINT ( 'NONE',  ( -6.448748702180637338, -26.64985754041175525, 6.700000000000000178 ) ) ;
#19145=CARTESIAN_POINT ( 'NONE',  ( -36.87867591359218977, -26.64985754041175525, 6.800000000000000711 ) ) ;
#19162=CARTESIAN_POINT ( 'NONE',  ( -34.34874870218063592, -26.64985754041175525, 6.700000000000000178 ) ) ;
#19171=CARTESIAN_POINT ( 'NONE',  ( -40.24874870218063450, -26.64985754041175525, 6.700000000000000178 ) ) ;
#19175=ORIENTED_EDGE ( 'NONE', *, *, #9514, .T. ) ;
#19176=DIRECTION ( 'NONE',  ( 1.000000000000000000, 0.000000000000000000, -0.000000000000000000 ) ) ;
#19191=ORIENTED_EDGE ( 'NONE', *, *, #3069, .F. ) ;
#19195=AXIS2_PLACEMENT_3D ( 'NONE', #31301, #24705, #619 ) ;
#19227=AXIS2_PLACEMENT_3D ( 'NONE', #38492, #6819, #444 ) ;
#19232=VERTEX_POINT ( 'NONE', #30352 ) ;
#19233=CYLINDRICAL_SURFACE ( 'NONE', #27191, 0.1000000000000028644 ) ;
#19246=DIRECTION ( 'NONE',  ( -0.000000000000000000, -0.000000000000000000, 1.000000000000000000 ) ) ;
#19260=AXIS2_PLACEMENT_3D ( 'NONE', #37142, #25409, #15523 ) ;
#19266=ADVANCED_FACE ( 'NONE', ( #4823 ), #29931, .F. ) ;
#19278=EDGE_LOOP ( 'NONE', ( #12437, #24354, #23853, #8179 ) ) ;
#19280=ORIENTED_EDGE ( 'NONE', *, *, #7898, .T. ) ;
#19284=CIRCLE ( 'NONE', #25868, 0.1000000000000028644 ) ;
#19307=EDGE_CURVE ( 'NONE', #20724, #11501, #37527, .T. ) ;
#19310=ADVANCED_FACE ( 'NONE', ( #6049 ), #31171, .F. ) ;
#19316=VERTEX_POINT ( 'NONE', #25187 ) ;
#19319=PRODUCT_DEFINITION_SHAPE ( 'NONE', 'NONE',  #35317 ) ;
#19322=ORIENTED_EDGE ( 'NONE', *, *, #37217, .F. ) ;
#19329=VERTEX_POINT ( 'NONE', #21287 ) ;
#19334=ORIENTED_EDGE ( 'NONE', *, *, #30824, .F. ) ;
#19335=ORIENTED_EDGE ( 'NONE', *, *, #23077, .F. ) ;
#19337=CIRCLE ( 'NONE', #1593, 0.1000000000000028644 ) ;
#19340=DIRECTION ( 'NONE',  ( -0.000000000000000000, -0.000000000000000000, 1.000000000000000000 ) ) ;
#19345=CARTESIAN_POINT ( 'NONE',  ( 3.121324086407806231, -26.64985754041175525, 6.700000000000000178 ) ) ;
#19353=VERTEX_POINT ( 'NONE', #24573 ) ;
#19357=CIRCLE ( 'NONE', #230, 0.1000000000000028644 ) ;
#19358=CIRCLE ( 'NONE', #1608, 0.1000000000000028644 ) ;
#19360=EDGE_CURVE ( 'NONE', #23338, #20694, #27855, .T. ) ;
#19365=CARTESIAN_POINT ( 'NONE',  ( -16.24874870218063450, -25.49307895267003587, 6.700000000000000178 ) ) ;
#19375=ORIENTED_EDGE ( 'NONE', *, *, #27185, .F. ) ;
#19380=CARTESIAN_POINT ( 'NONE',  ( -27.07867591359219972, -24.55319635012989110, 6.700000000000000178 ) ) ;
#19388=VERTEX_POINT ( 'NONE', #24991 ) ;
#19392=EDGE_CURVE ( 'NONE', #24473, #4930, #6251, .T. ) ;
#19396=ADVANCED_FACE ( 'NONE', ( #24784 ), #18798, .F. ) ;
#19409=CARTESIAN_POINT ( 'NONE',  ( -31.07867591359219617, -26.64985754041175525, 6.800000000000000711 ) ) ;
#19412=CARTESIAN_POINT ( 'NONE',  ( 11.65737507970504616, -38.28842912540938670, 6.000000000000000000 ) ) ;
#19417=CARTESIAN_POINT ( 'NONE',  ( -30.87867591359218977, -24.55319635012989110, 6.700000000000000178 ) ) ;
#19418=VECTOR ( 'NONE', #10651, 1000.000000000000000 ) ;
#19422=DIRECTION ( 'NONE',  ( 0.000000000000000000, 0.000000000000000000, 1.000000000000000000 ) ) ;
#19425=EDGE_LOOP ( 'NONE', ( #28802, #16477, #29845, #7089 ) ) ;
#19440=EDGE_CURVE ( 'NONE', #3076, #28543, #30771, .T. ) ;
#19445=DIRECTION ( 'NONE',  ( -0.000000000000000000, -1.000000000000000000, -0.000000000000000000 ) ) ;
#19450=CARTESIAN_POINT ( 'NONE',  ( -24.97867591359219475, -24.55319635012989110, 6.700000000000000178 ) ) ;
#19451=ORIENTED_EDGE ( 'NONE', *, *, #27615, .T. ) ;
#19455=AXIS2_PLACEMENT_3D ( 'NONE', #36775, #24423, #27514 ) ;
#19460=CARTESIAN_POINT ( 'NONE',  ( -44.23414840393349579, -23.60493063168010153, 6.800000000000000711 ) ) ;
#19467=CARTESIAN_POINT ( 'NONE',  ( -8.878675913592189772, -26.64985754041175525, 6.700000000000000178 ) ) ;
#19473=CIRCLE ( 'NONE', #23402, 0.1000000000000028644 ) ;
#19474=CARTESIAN_POINT ( 'NONE',  ( -2.878675913592191993, -24.55319635012989110, 6.700000000000000178 ) ) ;
#19475=AXIS2_PLACEMENT_3D ( 'NONE', #34396, #12331, #22434 ) ;
#19479=EDGE_LOOP ( 'NONE', ( #12303, #30789, #27996, #34702 ) ) ;
#19482=VECTOR ( 'NONE', #32624, 1000.000000000000000 ) ;
#19485=EDGE_LOOP ( 'NONE', ( #32163, #12571, #10101, #32214 ) ) ;
#19486=CARTESIAN_POINT ( 'NONE',  ( -54.01549048184568846, -30.38627270959228710, 6.000000000000000000 ) ) ;
#19493=EDGE_LOOP ( 'NONE', ( #34215, #4152, #2326, #31087 ) ) ;
#19494=ADVANCED_FACE ( 'NONE', ( #34072 ), #30971, .T. ) ;
#19496=EDGE_CURVE ( 'NONE', #2944, #39282, #12211, .T. ) ;
#19501=EDGE_LOOP ( 'NONE', ( #21829, #21526, #35715, #14050 ) ) ;
#19503=EDGE_LOOP ( 'NONE', ( #25072, #10003, #3710, #12963 ) ) ;
#19513=CARTESIAN_POINT ( 'NONE',  ( -12.87867591359218977, -26.64985754041175525, 6.800000000000000711 ) ) ;
#19516=CARTESIAN_POINT ( 'NONE',  ( -34.87867591359218977, -24.55319635012989110, 6.700000000000000178 ) ) ;
#19520=CARTESIAN_POINT ( 'NONE',  ( -0.4487487021806388365, -26.64985754041175525, 6.700000000000000178 ) ) ;
#19521=EDGE_CURVE ( 'NONE', #10099, #36832, #21387, .T. ) ;
#19525=CYLINDRICAL_SURFACE ( 'NONE', #16506, 0.1000000000000028644 ) ;
#19532=CIRCLE ( 'NONE', #38585, 2.500000000000002220 ) ;
#19537=AXIS2_PLACEMENT_3D ( 'NONE', #26306, #10634, #26702 ) ;
#19539=EDGE_LOOP ( 'NONE', ( #13805, #18344, #30820, #33016 ) ) ;
#19544=DIRECTION ( 'NONE',  ( -0.000000000000000000, -0.000000000000000000, 1.000000000000000000 ) ) ;
#19549=CARTESIAN_POINT ( 'NONE',  ( 2.921324086407800280, -24.55319635012989110, 6.700000000000000178 ) ) ;
#19553=ORIENTED_EDGE ( 'NONE', *, *, #35580, .T. ) ;
#19555=ORIENTED_EDGE ( 'NONE', *, *, #19977, .F. ) ;
#19556=CARTESIAN_POINT ( 'NONE',  ( -38.87867591359218977, -26.64985754041175525, 6.700000000000000178 ) ) ;
#19570=DIRECTION ( 'NONE',  ( 0.000000000000000000, 1.000000000000000000, 0.000000000000000000 ) ) ;
#19571=VECTOR ( 'NONE', #36736, 1000.000000000000000 ) ;
#19574=CIRCLE ( 'NONE', #18227, 0.1000000000000028644 ) ;
#19575=CARTESIAN_POINT ( 'NONE',  ( -28.24874870218063805, -25.49307895267003587, 6.700000000000000178 ) ) ;
#19582=VERTEX_POINT ( 'NONE', #6661 ) ;
#19588=FACE_BOUND ( 'NONE', #8657, .T. ) ;
#19594=EDGE_CURVE ( 'NONE', #32703, #1854, #12819, .T. ) ;
#19598=DIRECTION ( 'NONE',  ( 1.000000000000000000, 0.000000000000000000, 0.000000000000000000 ) ) ;
#19602=AXIS2_PLACEMENT_3D ( 'NONE', #11681, #24257, #39695 ) ;
#19603=PLANE ( 'NONE',  #22818 ) ;
#19605=DIRECTION ( 'NONE',  ( -0.000000000000000000, -0.000000000000000000, 1.000000000000000000 ) ) ;
#19612=ORIENTED_EDGE ( 'NONE', *, *, #4839, .F. ) ;
#19613=DIRECTION ( 'NONE',  ( 0.000000000000000000, 0.000000000000000000, 1.000000000000000000 ) ) ;
#19614=FACE_OUTER_BOUND ( 'NONE', #14468, .T. ) ;
#19630=ORIENTED_EDGE ( 'NONE', *, *, #18441, .F. ) ;
#19632=CARTESIAN_POINT ( 'NONE',  ( -2.878675913592191993, -24.55319635012989110, 6.800000000000000711 ) ) ;
#19640=VECTOR ( 'NONE', #7427, 1000.000000000000000 ) ;
#19653=ORIENTED_EDGE ( 'NONE', *, *, #11786, .F. ) ;
#19656=VERTEX_POINT ( 'NONE', #26406 ) ;
#19661=ORIENTED_EDGE ( 'NONE', *, *, #38252, .T. ) ;
#19667=DIRECTION ( 'NONE',  ( 1.000000000000000000, 0.000000000000000000, 0.000000000000000000 ) ) ;
#19669=LINE ( 'NONE', #38185, #39432 ) ;
#19673=CARTESIAN_POINT ( 'NONE',  ( -40.24874870218063450, -26.64985754041175525, 6.700000000000000178 ) ) ;
#19678=EDGE_CURVE ( 'NONE', #20726, #28508, #21532, .T. ) ;
#19680=PLANE ( 'NONE',  #14287 ) ;
#19686=ORIENTED_EDGE ( 'NONE', *, *, #168, .T. ) ;
#19687=ORIENTED_EDGE ( 'NONE', *, *, #528, .T. ) ;
#19690=CARTESIAN_POINT ( 'NONE',  ( -39.07867591359219261, -24.55319635012989110, 6.700000000000000178 ) ) ;
#19691=ORIENTED_EDGE ( 'NONE', *, *, #15103, .F. ) ;
#19694=AXIS2_PLACEMENT_3D ( 'NONE', #8841, #11925, #24085 ) ;
#19696=DIRECTION ( 'NONE',  ( 0.000000000000000000, 1.000000000000000000, 0.000000000000000000 ) ) ;
#19709=CARTESIAN_POINT ( 'NONE',  ( -18.34874870218063947, -26.64985754041175525, 6.800000000000000711 ) ) ;
#19730=CARTESIAN_POINT ( 'NONE',  ( 11.65737507970504439, -23.60493063168009442, 6.800000000000000711 ) ) ;
#19736=CARTESIAN_POINT ( 'NONE',  ( 1.121324086407811338, -26.64985754041175525, 6.700000000000000178 ) ) ;
#19743=DIRECTION ( 'NONE',  ( -0.000000000000000000, -0.000000000000000000, 1.000000000000000000 ) ) ;
#19749=ORIENTED_EDGE ( 'NONE', *, *, #6152, .T. ) ;
#19751=AXIS2_PLACEMENT_3D ( 'NONE', #20810, #18121, #33406 ) ;
#19764=EDGE_LOOP ( 'NONE', ( #5259, #12367, #24945, #21506 ) ) ;
#19767=AXIS2_PLACEMENT_3D ( 'NONE', #5232, #5644, #27858 ) ;
#19769=EDGE_CURVE ( 'NONE', #8458, #13946, #26248, .T. ) ;
#19771=EDGE_CURVE ( 'NONE', #9354, #8785, #34924, .T. ) ;
#19774=ORIENTED_EDGE ( 'NONE', *, *, #35777, .T. ) ;
#19782=FACE_OUTER_BOUND ( 'NONE', #18392, .T. ) ;
#19788=CARTESIAN_POINT ( 'NONE',  ( -22.97867591359219119, -24.55319635012989110, 6.700000000000000178 ) ) ;
#19790=ORIENTED_EDGE ( 'NONE', *, *, #7898, .F. ) ;
#19798=DIRECTION ( 'NONE',  ( 0.000000000000000000, 1.000000000000000000, 0.000000000000000000 ) ) ;
#19799=VECTOR ( 'NONE', #15898, 1000.000000000000000 ) ;
#19802=DIRECTION ( 'NONE',  ( 0.000000000000000000, 0.000000000000000000, 1.000000000000000000 ) ) ;
#19810=DIRECTION ( 'NONE',  ( -1.000000000000000000, 0.000000000000000000, 0.000000000000000000 ) ) ;
#19813=DIRECTION ( 'NONE',  ( 0.000000000000000000, 0.000000000000000000, 1.000000000000000000 ) ) ;
#19827=CARTESIAN_POINT ( 'NONE',  ( -24.24874870218063450, -25.49307895267003587, 6.800000000000000711 ) ) ;
#19831=CARTESIAN_POINT ( 'NONE',  ( -32.97867591359219119, -24.55319635012989110, 6.800000000000000711 ) ) ;
#19838=AXIS2_PLACEMENT_3D ( 'NONE', #11304, #24079, #5155 ) ;
#19851=CARTESIAN_POINT ( 'NONE',  ( -32.24874870218063450, -26.64985754041175525, 6.800000000000000711 ) ) ;
#19858=DIRECTION ( 'NONE',  ( 1.000000000000000000, 0.000000000000000000, 0.000000000000000000 ) ) ;
#19861=CARTESIAN_POINT ( 'NONE',  ( -16.87867591359218977, -26.64985754041175525, 6.700000000000000178 ) ) ;
#19863=FACE_OUTER_BOUND ( 'NONE', #10360, .T. ) ;
#19868=ORIENTED_EDGE ( 'NONE', *, *, #30483, .T. ) ;
#19870=VECTOR ( 'NONE', #44, 1000.000000000000000 ) ;
#19872=DIRECTION ( 'NONE',  ( 1.000000000000000000, 0.000000000000000000, -0.000000000000000000 ) ) ;
#19875=FACE_OUTER_BOUND ( 'NONE', #35649, .T. ) ;
#19877=EDGE_CURVE ( 'NONE', #34412, #273, #1187, .T. ) ;
#19880=ORIENTED_EDGE ( 'NONE', *, *, #877, .T. ) ;
#19887=CARTESIAN_POINT ( 'NONE',  ( -10.44874870218064089, -26.64985754041175525, 6.700000000000000178 ) ) ;
#19892=ORIENTED_EDGE ( 'NONE', *, *, #22004, .T. ) ;
#19894=AXIS2_PLACEMENT_3D ( 'NONE', #33257, #26863, #36738 ) ;
#19900=PLANE ( 'NONE',  #26102 ) ;
#19902=CARTESIAN_POINT ( 'NONE',  ( 4.921324086407802056, -24.55319635012989110, 6.700000000000000178 ) ) ;
#19907=CARTESIAN_POINT ( 'NONE',  ( -42.83131703149249603, -29.56993018339339940, 6.800000000000000711 ) ) ;
#19911=EDGE_CURVE ( 'NONE', #10365, #25891, #15945, .T. ) ;
#19912=ORIENTED_EDGE ( 'NONE', *, *, #34604, .F. ) ;
#19915=AXIS2_PLACEMENT_3D ( 'NONE', #17187, #20279, #32459 ) ;
#19922=ORIENTED_EDGE ( 'NONE', *, *, #1938, .F. ) ;
#19923=DIRECTION ( 'NONE',  ( 0.000000000000000000, 0.000000000000000000, -1.000000000000000000 ) ) ;
#19925=EDGE_LOOP ( 'NONE', ( #39398, #29953, #33788, #16991 ) ) ;
#19942=ADVANCED_FACE ( 'NONE', ( #6893 ), #3230, .F. ) ;
#19950=ORIENTED_EDGE ( 'NONE', *, *, #13576, .F. ) ;
#19952=CARTESIAN_POINT ( 'NONE',  ( -40.24874870218063450, -25.49307895267003587, 6.700000000000000178 ) ) ;
#19955=DIRECTION ( 'NONE',  ( -0.000000000000000000, -0.000000000000000000, 1.000000000000000000 ) ) ;
#19959=ORIENTED_EDGE ( 'NONE', *, *, #24625, .T. ) ;
#19960=LINE ( 'NONE', #13791, #38809 ) ;
#19961=DIRECTION ( 'NONE',  ( -0.000000000000000000, -1.000000000000000000, -0.000000000000000000 ) ) ;
#19964=ORIENTED_EDGE ( 'NONE', *, *, #16673, .F. ) ;
#19970=ADVANCED_FACE ( 'NONE', ( #34508 ), #13264, .F. ) ;
#19977=EDGE_CURVE ( 'NONE', #37652, #18339, #16711, .T. ) ;
#19980=EDGE_CURVE ( 'NONE', #28082, #13946, #25831, .T. ) ;
#19990=EDGE_CURVE ( 'NONE', #20522, #25319, #32024, .T. ) ;
#19994=CYLINDRICAL_SURFACE ( 'NONE', #24294, 0.1000000000000028644 ) ;
#19997=CARTESIAN_POINT ( 'NONE',  ( -38.34874870218063592, -25.49307895267003587, 6.700000000000000178 ) ) ;
#20006=AXIS2_PLACEMENT_3D ( 'NONE', #2497, #25114, #37644 ) ;
#20012=DIRECTION ( 'NONE',  ( 1.000000000000000000, 0.000000000000000000, 0.000000000000000000 ) ) ;
#20017=DIRECTION ( 'NONE',  ( 1.000000000000000000, 0.000000000000000000, -0.000000000000000000 ) ) ;
#20018=VECTOR ( 'NONE', #7450, 1000.000000000000000 ) ;
#20020=CIRCLE ( 'NONE', #22010, 0.1000000000000028644 ) ;
#20030=PLANE ( 'NONE',  #25446 ) ;
#20044=EDGE_CURVE ( 'NONE', #29402, #863, #28557, .T. ) ;
#20054=CARTESIAN_POINT ( 'NONE',  ( -28.44874870218064444, -25.49307895267003587, 6.700000000000000178 ) ) ;
#20067=CARTESIAN_POINT ( 'NONE',  ( -30.24874870218063805, -26.64985754041175525, 6.800000000000000711 ) ) ;
#20068=VERTEX_POINT ( 'NONE', #18615 ) ;
#20078=ORIENTED_EDGE ( 'NONE', *, *, #6153, .T. ) ;
#20081=AXIS2_PLACEMENT_3D ( 'NONE', #38860, #10254, #39051 ) ;
#20082=ORIENTED_EDGE ( 'NONE', *, *, #16324, .F. ) ;
#20087=PLANE ( 'NONE',  #13995 ) ;
#20100=FACE_OUTER_BOUND ( 'NONE', #14172, .T. ) ;
#20118=ORIENTED_EDGE ( 'NONE', *, *, #6943, .F. ) ;
#20130=ORIENTED_EDGE ( 'NONE', *, *, #19771, .F. ) ;
#20133=EDGE_CURVE ( 'NONE', #19316, #29188, #3432, .T. ) ;
#20138=CYLINDRICAL_SURFACE ( 'NONE', #35727, 0.1000000000000028644 ) ;
#20140=ORIENTED_EDGE ( 'NONE', *, *, #480, .T. ) ;
#20153=DIRECTION ( 'NONE',  ( 1.000000000000000000, -0.000000000000000000, 0.000000000000000000 ) ) ;
#20155=LINE ( 'NONE', #13580, #8213 ) ;
#20157=DIRECTION ( 'NONE',  ( 0.000000000000000000, 1.000000000000000000, 0.000000000000000000 ) ) ;
#20158=LINE ( 'NONE', #4139, #3358 ) ;
#20159=DIRECTION ( 'NONE',  ( -0.000000000000000000, -1.000000000000000000, -0.000000000000000000 ) ) ;
#20163=VERTEX_POINT ( 'NONE', #19851 ) ;
#20173=ORIENTED_EDGE ( 'NONE', *, *, #29343, .F. ) ;
#20179=ORIENTED_EDGE ( 'NONE', *, *, #37591, .T. ) ;
#20188=CARTESIAN_POINT ( 'NONE',  ( -0.8786759135921904385, -26.64985754041175525, 6.700000000000000178 ) ) ;
#20196=AXIS2_PLACEMENT_3D ( 'NONE', #18033, #39655, #2214 ) ;
#20197=LINE ( 'NONE', #1291, #24041 ) ;
#20198=AXIS2_PLACEMENT_3D ( 'NONE', #14066, #10973, #33026 ) ;
#20208=EDGE_CURVE ( 'NONE', #9480, #39964, #7528, .T. ) ;
#20211=ORIENTED_EDGE ( 'NONE', *, *, #3167, .F. ) ;
#20214=FACE_OUTER_BOUND ( 'NONE', #6972, .T. ) ;
#20216=EDGE_CURVE ( 'NONE', #3101, #30906, #5419, .T. ) ;
#20218=ORIENTED_EDGE ( 'NONE', *, *, #11795, .T. ) ;
#20224=AXIS2_PLACEMENT_3D ( 'NONE', #9287, #3165, #28230 ) ;
#20231=ORIENTED_EDGE ( 'NONE', *, *, #15714, .F. ) ;
#20240=ORIENTED_EDGE ( 'NONE', *, *, #37643, .F. ) ;
#20241=AXIS2_PLACEMENT_3D ( 'NONE', #20481, #7734, #4654 ) ;
#20256=DIRECTION ( 'NONE',  ( 0.000000000000000000, 0.000000000000000000, 1.000000000000000000 ) ) ;
#20257=AXIS2_PLACEMENT_3D ( 'NONE', #26693, #32475, #11218 ) ;
#20259=EDGE_LOOP ( 'NONE', ( #34995, #27526, #20179, #3097 ) ) ;
#20263=EDGE_CURVE ( 'NONE', #10252, #38102, #39048, .T. ) ;
#20266=EDGE_CURVE ( 'NONE', #3811, #4425, #20020, .T. ) ;
#20271=CARTESIAN_POINT ( 'NONE',  ( -34.87867591359218977, -26.64985754041175525, 6.700000000000000178 ) ) ;
#20273=VERTEX_POINT ( 'NONE', #30542 ) ;
#20278=VECTOR ( 'NONE', #27501, 1000.000000000000000 ) ;
#20279=DIRECTION ( 'NONE',  ( 1.000000000000000000, -0.000000000000000000, 0.000000000000000000 ) ) ;
#20283=DIRECTION ( 'NONE',  ( 0.000000000000000000, 1.000000000000000000, 0.000000000000000000 ) ) ;
#20289=DIRECTION ( 'NONE',  ( 1.000000000000000000, 0.000000000000000000, 0.000000000000000000 ) ) ;
#20290=LINE ( 'NONE', #13522, #21515 ) ;
#20292=DIRECTION ( 'NONE',  ( 0.000000000000000000, 1.000000000000000000, 0.000000000000000000 ) ) ;
#20305=DIRECTION ( 'NONE',  ( -0.000000000000000000, -1.000000000000000000, -0.000000000000000000 ) ) ;
#20315=CARTESIAN_POINT ( 'NONE',  ( -9.078675913592196167, -26.64985754041175525, 6.700000000000000178 ) ) ;
#20316=ORIENTED_EDGE ( 'NONE', *, *, #5773, .T. ) ;
#20318=VECTOR ( 'NONE', #32910, 1000.000000000000000 ) ;
#20321=LINE ( 'NONE', #4692, #27952 ) ;
#20328=CARTESIAN_POINT ( 'NONE',  ( -16.87867591359218977, -26.64985754041175525, 6.800000000000000711 ) ) ;
#20333=ORIENTED_EDGE ( 'NONE', *, *, #39543, .F. ) ;
#20334=CARTESIAN_POINT ( 'NONE',  ( -12.34874870218063947, -25.49307895267003587, 6.800000000000000711 ) ) ;
#20336=VECTOR ( 'NONE', #12709, 1000.000000000000000 ) ;
#20346=PLANE ( 'NONE',  #36541 ) ;
#20348=ADVANCED_FACE ( 'NONE', ( #24144 ), #8694, .F. ) ;
#20353=CARTESIAN_POINT ( 'NONE',  ( -40.24874870218063450, -25.49307895267003587, 6.800000000000000711 ) ) ;
#20357=CARTESIAN_POINT ( 'NONE',  ( -34.24874870218063450, -25.49307895267003587, 6.700000000000000178 ) ) ;
#20358=PLANE ( 'NONE',  #21120 ) ;
#20366=VECTOR ( 'NONE', #29628, 1000.000000000000000 ) ;
#20373=ORIENTED_EDGE ( 'NONE', *, *, #865, .F. ) ;
#20379=LINE ( 'NONE', #4158, #21983 ) ;
#20381=DIRECTION ( 'NONE',  ( 1.000000000000000000, 0.000000000000000000, -0.000000000000000000 ) ) ;
#20388=LINE ( 'NONE', #1285, #15101 ) ;
#20390=DIRECTION ( 'NONE',  ( 0.000000000000000000, 1.000000000000000000, 0.000000000000000000 ) ) ;
#20394=EDGE_CURVE ( 'NONE', #29514, #22775, #21070, .T. ) ;
#20395=ADVANCED_FACE ( 'NONE', ( #18372 ), #33447, .T. ) ;
#20401=DIRECTION ( 'NONE',  ( 1.000000000000000000, 0.000000000000000000, 0.000000000000000000 ) ) ;
#20402=FACE_OUTER_BOUND ( 'NONE', #935, .T. ) ;
#20408=AXIS2_PLACEMENT_3D ( 'NONE', #22466, #18745, #438 ) ;
#20409=EDGE_CURVE ( 'NONE', #33969, #15938, #19358, .T. ) ;
#20415=EDGE_LOOP ( 'NONE', ( #35499, #19119, #11963, #39271 ) ) ;
#20424=VECTOR ( 'NONE', #26804, 1000.000000000000000 ) ;
#20426=ADVANCED_FACE ( 'NONE', ( #4129 ), #18571, .T. ) ;
#20440=LINE ( 'NONE', #4808, #5829 ) ;
#20448=ORIENTED_EDGE ( 'NONE', *, *, #4514, .F. ) ;
#20452=CARTESIAN_POINT ( 'NONE',  ( -0.8786759135921904385, -26.64985754041175525, 6.700000000000000178 ) ) ;
#20470=DIRECTION ( 'NONE',  ( 1.000000000000000000, 0.000000000000000000, 0.000000000000000000 ) ) ;
#20472=EDGE_CURVE ( 'NONE', #18231, #29781, #40395, .T. ) ;
#20475=DIRECTION ( 'NONE',  ( -0.000000000000000000, -0.000000000000000000, 1.000000000000000000 ) ) ;
#20479=CYLINDRICAL_SURFACE ( 'NONE', #29127, 0.1000000000000028644 ) ;
#20481=CARTESIAN_POINT ( 'NONE',  ( -18.97867591359219475, -24.55319635012989110, 6.700000000000000178 ) ) ;
#20488=ADVANCED_FACE ( 'NONE', ( #9516 ), #6450, .F. ) ;
#20491=DIRECTION ( 'NONE',  ( 0.000000000000000000, 0.000000000000000000, 1.000000000000000000 ) ) ;
#20494=CARTESIAN_POINT ( 'NONE',  ( -20.24874870218063805, -26.64985754041175525, 6.700000000000000178 ) ) ;
#20498=LINE ( 'NONE', #23992, #4854 ) ;
#20510=ORIENTED_EDGE ( 'NONE', *, *, #34982, .T. ) ;
#20522=VERTEX_POINT ( 'NONE', #5321 ) ;
#20523=FACE_OUTER_BOUND ( 'NONE', #33294, .T. ) ;
#20529=DIRECTION ( 'NONE',  ( 1.000000000000000000, 0.000000000000000000, 0.000000000000000000 ) ) ;
#20537=DIRECTION ( 'NONE',  ( 0.000000000000000000, 0.000000000000000000, 1.000000000000000000 ) ) ;
#20538=DIRECTION ( 'NONE',  ( -0.000000000000000000, -0.000000000000000000, 1.000000000000000000 ) ) ;
#20542=ORIENTED_EDGE ( 'NONE', *, *, #27726, .F. ) ;
#20546=FACE_OUTER_BOUND ( 'NONE', #3406, .T. ) ;
#20555=DIRECTION ( 'NONE',  ( -0.000000000000000000, -1.000000000000000000, -0.000000000000000000 ) ) ;
#20557=ORIENTED_EDGE ( 'NONE', *, *, #34299, .F. ) ;
#20561=CARTESIAN_POINT ( 'NONE',  ( -38.24874870218063450, -25.49307895267003587, 6.800000000000000711 ) ) ;
#20562=DIRECTION ( 'NONE',  ( 1.000000000000000000, 0.000000000000000000, 0.000000000000000000 ) ) ;
#20563=ORIENTED_EDGE ( 'NONE', *, *, #18630, .F. ) ;
#20565=ORIENTED_EDGE ( 'NONE', *, *, #35580, .F. ) ;
#20575=LINE ( 'NONE', #13606, #18661 ) ;
#20587=EDGE_CURVE ( 'NONE', #24867, #26610, #39686, .T. ) ;
#20598=VECTOR ( 'NONE', #38356, 1000.000000000000000 ) ;
#20599=FACE_OUTER_BOUND ( 'NONE', #30689, .T. ) ;
#20604=DIRECTION ( 'NONE',  ( -0.000000000000000000, -0.000000000000000000, 1.000000000000000000 ) ) ;
#20608=ADVANCED_FACE ( 'NONE', ( #24038 ), #30028, .F. ) ;
#20618=CARTESIAN_POINT ( 'NONE',  ( -33.07867591359219972, -26.64985754041175525, 6.700000000000000178 ) ) ;
#20620=ORIENTED_EDGE ( 'NONE', *, *, #23652, .T. ) ;
#20627=VERTEX_POINT ( 'NONE', #23253 ) ;
#20632=CARTESIAN_POINT ( 'NONE',  ( -18.44874870218064089, -25.49307895267003587, 6.700000000000000178 ) ) ;
#20634=VECTOR ( 'NONE', #9136, 1000.000000000000000 ) ;
#20637=VECTOR ( 'NONE', #36244, 1000.000000000000000 ) ;
#20646=VERTEX_POINT ( 'NONE', #17247 ) ;
#20663=ORIENTED_EDGE ( 'NONE', *, *, #29479, .T. ) ;
#20668=DIRECTION ( 'NONE',  ( -0.000000000000000000, -0.000000000000000000, 1.000000000000000000 ) ) ;
#20674=PLANE ( 'NONE',  #4140 ) ;
#20679=ORIENTED_EDGE ( 'NONE', *, *, #2921, .T. ) ;
#20687=CIRCLE ( 'NONE', #15439, 0.1000000000000028644 ) ;
#20688=EDGE_CURVE ( 'NONE', #32700, #21196, #8596, .T. ) ;
#20692=ORIENTED_EDGE ( 'NONE', *, *, #9150, .T. ) ;
#20694=VERTEX_POINT ( 'NONE', #2246 ) ;
#20711=ADVANCED_FACE ( 'NONE', ( #21174 ), #21375, .F. ) ;
#20712=VERTEX_POINT ( 'NONE', #9409 ) ;
#20713=DIRECTION ( 'NONE',  ( 0.000000000000000000, 1.000000000000000000, 0.000000000000000000 ) ) ;
#20718=CARTESIAN_POINT ( 'NONE',  ( -34.97867591359219830, -26.64985754041175525, 6.700000000000000178 ) ) ;
#20719=FACE_OUTER_BOUND ( 'NONE', #24479, .T. ) ;
#20721=AXIS2_PLACEMENT_3D ( 'NONE', #35587, #16814, #16607 ) ;
#20724=VERTEX_POINT ( 'NONE', #3082 ) ;
#20725=EDGE_CURVE ( 'NONE', #513, #35057, #33954, .T. ) ;
#20726=VERTEX_POINT ( 'NONE', #30436 ) ;
#20734=DIRECTION ( 'NONE',  ( 1.000000000000000000, 0.000000000000000000, 0.000000000000000000 ) ) ;
#20736=CARTESIAN_POINT ( 'NONE',  ( -16.44874870218064089, -25.49307895267003587, 6.700000000000000178 ) ) ;
#20737=CARTESIAN_POINT ( 'NONE',  ( -36.97867591359219119, -26.64985754041175525, 6.700000000000000178 ) ) ;
#20744=AXIS2_PLACEMENT_3D ( 'NONE', #38302, #22282, #19176 ) ;
#20751=ORIENTED_EDGE ( 'NONE', *, *, #2148, .T. ) ;
#20767=CARTESIAN_POINT ( 'NONE',  ( -42.24874870218063450, -26.64985754041175525, 6.700000000000000178 ) ) ;
#20768=CARTESIAN_POINT ( 'NONE',  ( -12.97867591359219297, -26.64985754041175525, 6.700000000000000178 ) ) ;
#20774=VECTOR ( 'NONE', #24482, 1000.000000000000000 ) ;
#20788=EDGE_LOOP ( 'NONE', ( #35452, #11100, #3148, #38395 ) ) ;
#20797=CARTESIAN_POINT ( 'NONE',  ( -24.44874870218064089, -26.64985754041175525, 6.700000000000000178 ) ) ;
#20805=CARTESIAN_POINT ( 'NONE',  ( 2.921324086407800280, -26.64985754041175525, 6.700000000000000178 ) ) ;
#20810=CARTESIAN_POINT ( 'NONE',  ( -8.348748702180635917, -25.49307895267003587, 6.800000000000000711 ) ) ;
#20811=VECTOR ( 'NONE', #39531, 1000.000000000000000 ) ;
#20814=CARTESIAN_POINT ( 'NONE',  ( -16.24874870218063450, -25.49307895267003587, 6.800000000000000711 ) ) ;
#20817=CARTESIAN_POINT ( 'NONE',  ( -34.24874870218063450, -25.49307895267003587, 6.800000000000000711 ) ) ;
#20820=CARTESIAN_POINT ( 'NONE',  ( 5.651251297819362307, -26.64985754041175525, 6.700000000000000178 ) ) ;
#20823=CYLINDRICAL_SURFACE ( 'NONE', #23928, 0.1000000000000028644 ) ;
#20829=DIRECTION ( 'NONE',  ( -0.000000000000000000, -0.000000000000000000, 1.000000000000000000 ) ) ;
#20834=CIRCLE ( 'NONE', #3139, 0.1000000000000028644 ) ;
#20845=AXIS2_PLACEMENT_3D ( 'NONE', #15592, #2656, #37203 ) ;
#20847=ORIENTED_EDGE ( 'NONE', *, *, #25489, .F. ) ;
#20851=EDGE_LOOP ( 'NONE', ( #27862, #36687, #31900, #8407 ) ) ;
#20853=EDGE_CURVE ( 'NONE', #212, #29188, #18680, .T. ) ;
#20854=CARTESIAN_POINT ( 'NONE',  ( -38.24874870218063450, -26.64985754041175525, 6.800000000000000711 ) ) ;
#20855=DIRECTION ( 'NONE',  ( 0.000000000000000000, 0.000000000000000000, 1.000000000000000000 ) ) ;
#20856=ORIENTED_EDGE ( 'NONE', *, *, #27570, .T. ) ;
#20859=DIRECTION ( 'NONE',  ( 1.000000000000000000, 0.000000000000000000, 0.000000000000000000 ) ) ;
#20861=CARTESIAN_POINT ( 'NONE',  ( -33.07867591359219972, -26.64985754041175525, 6.700000000000000178 ) ) ;
#20863=DIRECTION ( 'NONE',  ( 1.000000000000000000, 0.000000000000000000, 0.000000000000000000 ) ) ;
#20867=LINE ( 'NONE', #36926, #30533 ) ;
#20872=VECTOR ( 'NONE', #27132, 1000.000000000000000 ) ;
#20875=EDGE_LOOP ( 'NONE', ( #3756, #34186, #19868, #40451 ) ) ;
#20876=ORIENTED_EDGE ( 'NONE', *, *, #24600, .F. ) ;
#20889=ORIENTED_EDGE ( 'NONE', *, *, #18262, .F. ) ;
#20890=DIRECTION ( 'NONE',  ( 0.000000000000000000, 0.000000000000000000, 1.000000000000000000 ) ) ;
#20891=DIRECTION ( 'NONE',  ( 1.000000000000000000, -0.000000000000000000, 0.000000000000000000 ) ) ;
#20905=EDGE_LOOP ( 'NONE', ( #37463, #18185, #9534, #6349 ) ) ;
#20909=CARTESIAN_POINT ( 'NONE',  ( -24.87867591359218977, -26.64985754041175525, 6.800000000000000711 ) ) ;
#20913=LINE ( 'NONE', #33500, #29950 ) ;
#20919=LINE ( 'NONE', #36973, #7474 ) ;
#20920=DIRECTION ( 'NONE',  ( -0.000000000000000000, -1.000000000000000000, -0.000000000000000000 ) ) ;
#20925=ORIENTED_EDGE ( 'NONE', *, *, #2821, .F. ) ;
#20935=CARTESIAN_POINT ( 'NONE',  ( -16.97867591359219475, -26.64985754041175525, 6.700000000000000178 ) ) ;
#20943=DIRECTION ( 'NONE',  ( -0.000000000000000000, -0.000000000000000000, 1.000000000000000000 ) ) ;
#20946=CYLINDRICAL_SURFACE ( 'NONE', #29773, 0.1000000000000028644 ) ;
#20949=DIRECTION ( 'NONE',  ( 0.000000000000000000, 0.000000000000000000, 1.000000000000000000 ) ) ;
#20950=CARTESIAN_POINT ( 'NONE',  ( -36.44874870218064444, -26.64985754041175525, 6.700000000000000178 ) ) ;
#20955=LINE ( 'NONE', #5928, #33417 ) ;
#20958=EDGE_CURVE ( 'NONE', #35983, #38495, #39080, .T. ) ;
#20970=EDGE_CURVE ( 'NONE', #38778, #34298, #38437, .T. ) ;
#20975=EDGE_LOOP ( 'NONE', ( #34860, #3476, #10456, #39304 ) ) ;
#20978=VECTOR ( 'NONE', #8167, 1000.000000000000000 ) ;
#20980=ORIENTED_EDGE ( 'NONE', *, *, #31579, .T. ) ;
#20987=PLANE ( 'NONE',  #12164 ) ;
#20988=ORIENTED_EDGE ( 'NONE', *, *, #13776, .T. ) ;
#20989=ORIENTED_EDGE ( 'NONE', *, *, #20263, .F. ) ;
#20991=DIRECTION ( 'NONE',  ( -0.000000000000000000, -0.000000000000000000, 1.000000000000000000 ) ) ;
#20993=ORIENTED_EDGE ( 'NONE', *, *, #20958, .F. ) ;
#20996=ORIENTED_EDGE ( 'NONE', *, *, #5109, .F. ) ;
#21002=ORIENTED_EDGE ( 'NONE', *, *, #12175, .T. ) ;
#21009=VERTEX_POINT ( 'NONE', #11219 ) ;
#21013=DIRECTION ( 'NONE',  ( -0.000000000000000000, -0.000000000000000000, 1.000000000000000000 ) ) ;
#21024=ORIENTED_EDGE ( 'NONE', *, *, #7675, .T. ) ;
#21031=DIRECTION ( 'NONE',  ( -0.000000000000000000, -0.000000000000000000, 1.000000000000000000 ) ) ;
#21043=AXIS2_PLACEMENT_3D ( 'NONE', #12395, #21872, #37694 ) ;
#21047=PLANE ( 'NONE',  #18188 ) ;
#21050=CARTESIAN_POINT ( 'NONE',  ( -8.448748702180639114, -26.64985754041175525, 6.700000000000000178 ) ) ;
#21051=EDGE_LOOP ( 'NONE', ( #365, #29724, #1824, #28012 ) ) ;
#21062=ORIENTED_EDGE ( 'NONE', *, *, #12983, .F. ) ;
#21067=CARTESIAN_POINT ( 'NONE',  ( -13.07867591359219617, -26.64985754041175525, 6.800000000000000711 ) ) ;
#21070=LINE ( 'NONE', #17543, #14740 ) ;
#21075=DIRECTION ( 'NONE',  ( -1.000000000000000000, -1.241493069327139093E-16, 0.000000000000000000 ) ) ;
#21084=DIRECTION ( 'NONE',  ( 1.000000000000000000, 0.000000000000000000, -0.000000000000000000 ) ) ;
#21088=LINE ( 'NONE', #33659, #5986 ) ;
#21090=ORIENTED_EDGE ( 'NONE', *, *, #12422, .T. ) ;
#21094=LINE ( 'NONE', #33664, #25362 ) ;
#21105=EDGE_LOOP ( 'NONE', ( #18890, #28566, #35852, #24371 ) ) ;
#21106=CARTESIAN_POINT ( 'NONE',  ( 7.121324086407810228, -26.64985754041175525, 6.700000000000000178 ) ) ;
#21109=ORIENTED_EDGE ( 'NONE', *, *, #37990, .F. ) ;
#21120=AXIS2_PLACEMENT_3D ( 'NONE', #4339, #39090, #36029 ) ;
#21123=ADVANCED_FACE ( 'NONE', ( #20100 ), #32476, .F. ) ;
#21132=VECTOR ( 'NONE', #22425, 1000.000000000000000 ) ;
#21142=FACE_OUTER_BOUND ( 'NONE', #9904, .T. ) ;
#21143=FACE_OUTER_BOUND ( 'NONE', #38203, .T. ) ;
#21144=CARTESIAN_POINT ( 'NONE',  ( 3.651251297819360531, -25.49307895267003587, 6.700000000000000178 ) ) ;
#21146=ORIENTED_EDGE ( 'NONE', *, *, #20044, .F. ) ;
#21148=ORIENTED_EDGE ( 'NONE', *, *, #39453, .T. ) ;
#21149=VERTEX_POINT ( 'NONE', #1789 ) ;
#21151=EDGE_CURVE ( 'NONE', #23320, #28333, #37795, .T. ) ;
#21158=VECTOR ( 'NONE', #11867, 1000.000000000000000 ) ;
#21159=LINE ( 'NONE', #33938, #35792 ) ;
#21162=PLANE ( 'NONE',  #15242 ) ;
#21166=VERTEX_POINT ( 'NONE', #33076 ) ;
#21171=DIRECTION ( 'NONE',  ( 0.000000000000000000, 0.000000000000000000, 1.000000000000000000 ) ) ;
#21174=FACE_OUTER_BOUND ( 'NONE', #6258, .T. ) ;
#21176=CARTESIAN_POINT ( 'NONE',  ( -32.87867591359218977, -26.64985754041175525, 6.700000000000000178 ) ) ;
#21184=EDGE_CURVE ( 'NONE', #2141, #37191, #21739, .T. ) ;
#21193=CYLINDRICAL_SURFACE ( 'NONE', #29041, 0.1000000000000028644 ) ;
#21195=DIRECTION ( 'NONE',  ( 1.000000000000000000, 0.000000000000000000, -0.000000000000000000 ) ) ;
#21196=VERTEX_POINT ( 'NONE', #5889 ) ;
#21197=ORIENTED_EDGE ( 'NONE', *, *, #6153, .F. ) ;
#21201=ORIENTED_EDGE ( 'NONE', *, *, #6383, .T. ) ;
#21207=DIRECTION ( 'NONE',  ( -0.000000000000000000, -1.000000000000000000, -0.000000000000000000 ) ) ;
#21208=EDGE_LOOP ( 'NONE', ( #32543, #28760, #25166, #39087 ) ) ;
#21214=EDGE_LOOP ( 'NONE', ( #21706, #12801, #28365, #33490 ) ) ;
#21216=LINE ( 'NONE', #39944, #18391 ) ;
#21221=CARTESIAN_POINT ( 'NONE',  ( -35.07867591359219972, -24.55319635012989110, 6.800000000000000711 ) ) ;
#21224=CARTESIAN_POINT ( 'NONE',  ( -51.21549048184568420, -30.38627270959228710, 6.000000000000000000 ) ) ;
#21227=LINE ( 'NONE', #34011, #26301 ) ;
#21232=DIRECTION ( 'NONE',  ( 1.000000000000000000, 0.000000000000000000, 0.000000000000000000 ) ) ;
#21238=EDGE_CURVE ( 'NONE', #10219, #25277, #10170, .T. ) ;
#21241=ORIENTED_EDGE ( 'NONE', *, *, #37504, .F. ) ;
#21242=LINE ( 'NONE', #40171, #291 ) ;
#21287=CARTESIAN_POINT ( 'NONE',  ( -33.07867591359219972, -24.55319635012989110, 6.800000000000000711 ) ) ;
#21288=CARTESIAN_POINT ( 'NONE',  ( -14.87867591359218977, -26.64985754041175525, 6.700000000000000178 ) ) ;
#21291=LINE ( 'NONE', #33864, #34347 ) ;
#21292=ORIENTED_EDGE ( 'NONE', *, *, #35018, .F. ) ;
#21293=DIRECTION ( 'NONE',  ( -0.000000000000000000, -0.000000000000000000, 1.000000000000000000 ) ) ;
#21295=VECTOR ( 'NONE', #9948, 1000.000000000000000 ) ;
#21298=PLANE ( 'NONE',  #22641 ) ;
#21300=CARTESIAN_POINT ( 'NONE',  ( -2.878675913592191993, -26.64985754041175525, 6.800000000000000711 ) ) ;
#21302=CARTESIAN_POINT ( 'NONE',  ( -34.87867591359218977, -24.55319635012989110, 6.700000000000000178 ) ) ;
#21314=CARTESIAN_POINT ( 'NONE',  ( -12.44874870218064267, -26.64985754041175525, 6.700000000000000178 ) ) ;
#21325=AXIS2_PLACEMENT_3D ( 'NONE', #32121, #4115, #29210 ) ;
#21330=CARTESIAN_POINT ( 'NONE',  ( -10.24874870218063450, -26.64985754041175525, 6.700000000000000178 ) ) ;
#21339=ORIENTED_EDGE ( 'NONE', *, *, #2109, .F. ) ;
#21343=LINE ( 'NONE', #33917, #18764 ) ;
#21347=ORIENTED_EDGE ( 'NONE', *, *, #35482, .F. ) ;
#21348=CARTESIAN_POINT ( 'NONE',  ( -16.34874870218063592, -26.64985754041175525, 6.700000000000000178 ) ) ;
#21350=ORIENTED_EDGE ( 'NONE', *, *, #4092, .F. ) ;
#21352=VECTOR ( 'NONE', #33855, 1000.000000000000000 ) ;
#21365=DIRECTION ( 'NONE',  ( -0.000000000000000000, -1.000000000000000000, -0.000000000000000000 ) ) ;
#21375=CYLINDRICAL_SURFACE ( 'NONE', #12824, 0.1000000000000028644 ) ;
#21376=ORIENTED_EDGE ( 'NONE', *, *, #32592, .F. ) ;
#21377=DIRECTION ( 'NONE',  ( 0.000000000000000000, 0.000000000000000000, 1.000000000000000000 ) ) ;
#21379=ADVANCED_FACE ( 'NONE', ( #5430 ), #27853, .T. ) ;
#21381=AXIS2_PLACEMENT_3D ( 'NONE', #27551, #40108, #30868 ) ;
#21387=CIRCLE ( 'NONE', #3663, 0.1000000000000028644 ) ;
#21394=VERTEX_POINT ( 'NONE', #12209 ) ;
#21401=EDGE_LOOP ( 'NONE', ( #29936, #22358, #34753, #11756 ) ) ;
#21402=DIRECTION ( 'NONE',  ( 0.000000000000000000, 0.000000000000000000, 1.000000000000000000 ) ) ;
#21416=ORIENTED_EDGE ( 'NONE', *, *, #16119, .T. ) ;
#21417=DIRECTION ( 'NONE',  ( 0.000000000000000000, 0.000000000000000000, 1.000000000000000000 ) ) ;
#21422=EDGE_LOOP ( 'NONE', ( #33871, #33991, #2600, #34480 ) ) ;
#21424=EDGE_CURVE ( 'NONE', #37652, #33400, #20867, .T. ) ;
#21427=CARTESIAN_POINT ( 'NONE',  ( 0.9213240864078056092, -24.55319635012989110, 6.800000000000000711 ) ) ;
#21428=EDGE_LOOP ( 'NONE', ( #17465, #2021, #34795, #22311 ) ) ;
#21435=CARTESIAN_POINT ( 'NONE',  ( -28.34874870218063947, -26.64985754041175525, 6.700000000000000178 ) ) ;
#21437=CARTESIAN_POINT ( 'NONE',  ( -1.078675913592196167, -26.64985754041175525, 6.700000000000000178 ) ) ;
#21449=DIRECTION ( 'NONE',  ( 0.000000000000000000, 0.000000000000000000, 1.000000000000000000 ) ) ;
#21456=DIRECTION ( 'NONE',  ( 1.000000000000000000, 0.000000000000000000, -0.000000000000000000 ) ) ;
#21458=CARTESIAN_POINT ( 'NONE',  ( -34.34874870218063592, -26.64985754041175525, 6.800000000000000711 ) ) ;
#21465=ORIENTED_EDGE ( 'NONE', *, *, #32386, .T. ) ;
#21468=LINE ( 'NONE', #2960, #39443 ) ;
#21473=ADVANCED_FACE ( 'NONE', ( #30969 ), #2775, .F. ) ;
#21484=EDGE_CURVE ( 'NONE', #21149, #2729, #33857, .T. ) ;
#21490=DIRECTION ( 'NONE',  ( 1.000000000000000000, 0.000000000000000000, 0.000000000000000000 ) ) ;
#21496=CARTESIAN_POINT ( 'NONE',  ( -22.87867591359218977, -26.64985754041175525, 6.700000000000000178 ) ) ;
#21506=ORIENTED_EDGE ( 'NONE', *, *, #20472, .F. ) ;
#21513=VECTOR ( 'NONE', #1894, 1000.000000000000000 ) ;
#21515=VECTOR ( 'NONE', #38225, 1000.000000000000000 ) ;
#21516=LINE ( 'NONE', #8930, #26485 ) ;
#21526=ORIENTED_EDGE ( 'NONE', *, *, #6333, .T. ) ;
#21530=ORIENTED_EDGE ( 'NONE', *, *, #168, .F. ) ;
#21532=LINE ( 'NONE', #37161, #37798 ) ;
#21534=AXIS2_PLACEMENT_3D ( 'NONE', #6135, #12505, #37610 ) ;
#21540=FACE_OUTER_BOUND ( 'NONE', #18748, .T. ) ;
#21541=CARTESIAN_POINT ( 'NONE',  ( -21.07867591359219617, -24.55319635012989110, 6.800000000000000711 ) ) ;
#21542=AXIS2_PLACEMENT_3D ( 'NONE', #33647, #9311, #24562 ) ;
#21546=DIRECTION ( 'NONE',  ( 1.000000000000000000, 0.000000000000000000, 0.000000000000000000 ) ) ;
#21558=DIRECTION ( 'NONE',  ( -0.000000000000000000, -0.000000000000000000, 1.000000000000000000 ) ) ;
#21563=DIRECTION ( 'NONE',  ( -0.000000000000000000, -0.000000000000000000, 1.000000000000000000 ) ) ;
#21569=AXIS2_PLACEMENT_3D ( 'NONE', #33135, #1853, #38889 ) ;
#21575=LINE ( 'NONE', #30640, #26531 ) ;
#21579=ORIENTED_EDGE ( 'NONE', *, *, #27918, .T. ) ;
#21580=CARTESIAN_POINT ( 'NONE',  ( -34.87867591359218977, -26.64985754041175525, 6.800000000000000711 ) ) ;
#21595=CYLINDRICAL_SURFACE ( 'NONE', #11652, 0.1000000000000028644 ) ;
#21608=VERTEX_POINT ( 'NONE', #492 ) ;
#21616=VERTEX_POINT ( 'NONE', #19412 ) ;
#21620=FACE_OUTER_BOUND ( 'NONE', #30160, .T. ) ;
#21621=DIRECTION ( 'NONE',  ( -1.000000000000000000, -1.273455763949465810E-16, 0.000000000000000000 ) ) ;
#21630=EDGE_LOOP ( 'NONE', ( #24898, #34345, #24673, #20980 ) ) ;
#21639=LINE ( 'NONE', #11936, #1950 ) ;
#21649=ORIENTED_EDGE ( 'NONE', *, *, #24250, .T. ) ;
#21655=CIRCLE ( 'NONE', #3932, 0.1000000000000028644 ) ;
#21659=LINE ( 'NONE', #34237, #18671 ) ;
#21661=CARTESIAN_POINT ( 'NONE',  ( 3.121324086407806231, -26.64985754041175525, 6.700000000000000178 ) ) ;
#21672=DIRECTION ( 'NONE',  ( 1.000000000000000000, 0.000000000000000000, -0.000000000000000000 ) ) ;
#21674=ADVANCED_FACE ( 'NONE', ( #1299 ), #13836, .F. ) ;
#21680=LINE ( 'NONE', #261, #33270 ) ;
#21683=CARTESIAN_POINT ( 'NONE',  ( -4.448748702180642667, -26.64985754041175525, 6.700000000000000178 ) ) ;
#21702=CARTESIAN_POINT ( 'NONE',  ( -18.24874870218063450, -25.49307895267003587, 6.700000000000000178 ) ) ;
#21703=CARTESIAN_POINT ( 'NONE',  ( -10.34874870218063769, -25.49307895267003587, 6.700000000000000178 ) ) ;
#21706=ORIENTED_EDGE ( 'NONE', *, *, #3699, .T. ) ;
#21714=ORIENTED_EDGE ( 'NONE', *, *, #27060, .F. ) ;
#21734=VERTEX_POINT ( 'NONE', #13634 ) ;
#21739=LINE ( 'NONE', #14715, #27922 ) ;
#21740=CARTESIAN_POINT ( 'NONE',  ( -12.44874870218064267, -26.64985754041175525, 6.700000000000000178 ) ) ;
#21752=DIRECTION ( 'NONE',  ( 1.000000000000000000, -0.000000000000000000, 0.000000000000000000 ) ) ;
#21759=ADVANCED_FACE ( 'NONE', ( #7250 ), #22910, .F. ) ;
#21767=CARTESIAN_POINT ( 'NONE',  ( -42.24874870218063450, -26.64985754041175525, 6.700000000000000178 ) ) ;
#21770=ORIENTED_EDGE ( 'NONE', *, *, #19521, .T. ) ;
#21773=CARTESIAN_POINT ( 'NONE',  ( -19.07867591359219972, -26.64985754041175525, 6.700000000000000178 ) ) ;
#21776=DIRECTION ( 'NONE',  ( 1.000000000000000000, 0.000000000000000000, 0.000000000000000000 ) ) ;
#21785=AXIS2_PLACEMENT_3D ( 'NONE', #5739, #11683, #24464 ) ;
#21806=CARTESIAN_POINT ( 'NONE',  ( -0.3487487021806359722, -25.49307895267003587, 6.700000000000000178 ) ) ;
#21812=ORIENTED_EDGE ( 'NONE', *, *, #9150, .F. ) ;
#21815=EDGE_LOOP ( 'NONE', ( #33207, #18993, #22583, #19334 ) ) ;
#21819=EDGE_CURVE ( 'NONE', #10291, #13813, #4973, .T. ) ;
#21829=ORIENTED_EDGE ( 'NONE', *, *, #37038, .T. ) ;
#21830=PLANE ( 'NONE',  #36225 ) ;
#21839=ORIENTED_EDGE ( 'NONE', *, *, #13387, .T. ) ;
#21843=DIRECTION ( 'NONE',  ( 0.000000000000000000, 0.000000000000000000, 1.000000000000000000 ) ) ;
#21848=CARTESIAN_POINT ( 'NONE',  ( -26.24874870218063450, -25.49307895267003587, 6.700000000000000178 ) ) ;
#21850=ORIENTED_EDGE ( 'NONE', *, *, #10410, .F. ) ;
#21855=EDGE_CURVE ( 'NONE', #34205, #17894, #17917, .T. ) ;
#21861=FACE_BOUND ( 'NONE', #18837, .T. ) ;
#21862=DIRECTION ( 'NONE',  ( -0.000000000000000000, -1.000000000000000000, -0.000000000000000000 ) ) ;
#21872=DIRECTION ( 'NONE',  ( 0.000000000000000000, 0.000000000000000000, 1.000000000000000000 ) ) ;
#21876=VECTOR ( 'NONE', #23910, 1000.000000000000000 ) ;
#21877=ORIENTED_EDGE ( 'NONE', *, *, #33534, .T. ) ;
#21886=CARTESIAN_POINT ( 'NONE',  ( -2.978675913592195190, -26.64985754041175525, 6.700000000000000178 ) ) ;
#21890=CARTESIAN_POINT ( 'NONE',  ( -53.21549048184568420, -38.28842912540938670, -4.152976064860135708 ) ) ;
#21891=CARTESIAN_POINT ( 'NONE',  ( -22.34874870218063947, -25.49307895267003587, 6.700000000000000178 ) ) ;
#21903=LINE ( 'NONE', #6255, #13858 ) ;
#21908=CIRCLE ( 'NONE', #17936, 0.1000000000000028644 ) ;
#21912=CARTESIAN_POINT ( 'NONE',  ( -20.24874870218063805, -26.64985754041175525, 6.700000000000000178 ) ) ;
#21917=ORIENTED_EDGE ( 'NONE', *, *, #12983, .T. ) ;
#21930=LINE ( 'NONE', #525, #219 ) ;
#21931=DIRECTION ( 'NONE',  ( -0.000000000000000000, -0.000000000000000000, -1.000000000000000000 ) ) ;
#21932=VERTEX_POINT ( 'NONE', #31320 ) ;
#21948=CARTESIAN_POINT ( 'NONE',  ( -16.87867591359218977, -24.55319635012989110, 6.700000000000000178 ) ) ;
#21950=DIRECTION ( 'NONE',  ( 1.000000000000000000, 0.000000000000000000, 0.000000000000000000 ) ) ;
#21951=AXIS2_PLACEMENT_3D ( 'NONE', #12771, #6813, #31937 ) ;
#21958=EDGE_CURVE ( 'NONE', #863, #2870, #4891, .T. ) ;
#21970=EDGE_CURVE ( 'NONE', #32703, #169, #6198, .T. ) ;
#21971=CARTESIAN_POINT ( 'NONE',  ( 1.551251297819356001, -25.49307895267003587, 6.700000000000000178 ) ) ;
#21972=VERTEX_POINT ( 'NONE', #31933 ) ;
#21980=ORIENTED_EDGE ( 'NONE', *, *, #36132, .T. ) ;
#21981=ORIENTED_EDGE ( 'NONE', *, *, #33410, .T. ) ;
#21982=CIRCLE ( 'NONE', #4232, 0.1000000000000028644 ) ;
#21983=VECTOR ( 'NONE', #13812, 1000.000000000000000 ) ;
#21989=ORIENTED_EDGE ( 'NONE', *, *, #12845, .T. ) ;
#21991=VECTOR ( 'NONE', #17826, 1000.000000000000000 ) ;
#21993=VECTOR ( 'NONE', #22246, 1000.000000000000000 ) ;
#21999=CARTESIAN_POINT ( 'NONE',  ( -42.34874870218063592, -26.64985754041175525, 6.700000000000000178 ) ) ;
#22002=EDGE_LOOP ( 'NONE', ( #16569, #6205, #36682, #29547 ) ) ;
#22004=EDGE_CURVE ( 'NONE', #12066, #25120, #8818, .T. ) ;
#22007=CARTESIAN_POINT ( 'NONE',  ( -4.878675913592187108, -24.55319635012989110, 6.700000000000000178 ) ) ;
#22010=AXIS2_PLACEMENT_3D ( 'NONE', #17958, #20855, #11770 ) ;
#22012=ORIENTED_EDGE ( 'NONE', *, *, #15068, .F. ) ;
#22019=AXIS2_PLACEMENT_3D ( 'NONE', #16700, #7655, #10531 ) ;
#22028=ORIENTED_EDGE ( 'NONE', *, *, #17745, .F. ) ;
#22031=DIRECTION ( 'NONE',  ( 1.000000000000000000, -0.000000000000000000, 0.000000000000000000 ) ) ;
#22041=CARTESIAN_POINT ( 'NONE',  ( -38.44874870218063734, -26.64985754041175525, 6.700000000000000178 ) ) ;
#22055=LINE ( 'NONE', #31934, #18915 ) ;
#22056=EDGE_CURVE ( 'NONE', #27310, #6781, #33180, .T. ) ;
#22057=EDGE_CURVE ( 'NONE', #5089, #20694, #38285, .T. ) ;
#22058=CARTESIAN_POINT ( 'NONE',  ( 3.651251297819360531, -26.64985754041175525, 6.700000000000000178 ) ) ;
#22059=EDGE_CURVE ( 'NONE', #29405, #10219, #13581, .T. ) ;
#22068=VECTOR ( 'NONE', #28631, 1000.000000000000000 ) ;
#22069=ORIENTED_EDGE ( 'NONE', *, *, #2580, .F. ) ;
#22074=FACE_BOUND ( 'NONE', #20975, .T. ) ;
#22091=LINE ( 'NONE', #25576, #19052 ) ;
#22106=DIRECTION ( 'NONE',  ( -0.000000000000000000, -0.000000000000000000, 1.000000000000000000 ) ) ;
#22113=DIRECTION ( 'NONE',  ( -0.000000000000000000, -0.000000000000000000, 1.000000000000000000 ) ) ;
#22116=DIRECTION ( 'NONE',  ( 1.000000000000000000, 0.000000000000000000, 0.000000000000000000 ) ) ;
#22121=VERTEX_POINT ( 'NONE', #25744 ) ;
#22123=DIRECTION ( 'NONE',  ( 1.000000000000000000, 0.000000000000000000, 0.000000000000000000 ) ) ;
#22127=LINE ( 'NONE', #34701, #5441 ) ;
#22130=DIRECTION ( 'NONE',  ( 1.000000000000000000, -0.000000000000000000, 0.000000000000000000 ) ) ;
#22160=DIRECTION ( 'NONE',  ( 0.000000000000000000, 1.000000000000000000, 0.000000000000000000 ) ) ;
#22161=CARTESIAN_POINT ( 'NONE',  ( 7.021324086407807030, -26.64985754041175525, 6.700000000000000178 ) ) ;
#22166=ORIENTED_EDGE ( 'NONE', *, *, #6804, .F. ) ;
#22168=ORIENTED_EDGE ( 'NONE', *, *, #22706, .T. ) ;
#22179=CARTESIAN_POINT ( 'NONE',  ( -51.01549048184568846, -38.28842912540938670, 6.800000000000000711 ) ) ;
#22180=EDGE_CURVE ( 'NONE', #24066, #7569, #4989, .T. ) ;
#22190=ORIENTED_EDGE ( 'NONE', *, *, #3402, .T. ) ;
#22192=DIRECTION ( 'NONE',  ( 0.000000000000000000, 1.000000000000000000, 0.000000000000000000 ) ) ;
#22195=EDGE_CURVE ( 'NONE', #30906, #25222, #23907, .T. ) ;
#22197=CARTESIAN_POINT ( 'NONE',  ( -8.448748702180639114, -25.49307895267003587, 6.800000000000000711 ) ) ;
#22198=VECTOR ( 'NONE', #35920, 1000.000000000000000 ) ;
#22202=VECTOR ( 'NONE', #33309, 1000.000000000000000 ) ;
#22204=LINE ( 'NONE', #34770, #34585 ) ;
#22207=LINE ( 'NONE', #28571, #39251 ) ;
#22212=LINE ( 'NONE', #31467, #13529 ) ;
#22219=VECTOR ( 'NONE', #39679, 1000.000000000000000 ) ;
#22226=CIRCLE ( 'NONE', #1856, 0.1000000000000028644 ) ;
#22227=AXIS2_PLACEMENT_3D ( 'NONE', #8316, #20891, #30372 ) ;
#22242=ADVANCED_FACE ( 'NONE', ( #37289 ), #15262, .T. ) ;
#22243=EDGE_CURVE ( 'NONE', #6003, #17955, #12381, .T. ) ;
#22245=VECTOR ( 'NONE', #26480, 1000.000000000000000 ) ;
#22246=DIRECTION ( 'NONE',  ( 0.000000000000000000, 1.000000000000000000, 0.000000000000000000 ) ) ;
#22247=FACE_OUTER_BOUND ( 'NONE', #37592, .T. ) ;
#22248=CARTESIAN_POINT ( 'NONE',  ( -30.44874870218064089, -26.64985754041175525, 6.800000000000000711 ) ) ;
#22251=EDGE_LOOP ( 'NONE', ( #35638, #9076, #32, #20316 ) ) ;
#22253=ORIENTED_EDGE ( 'NONE', *, *, #40093, .T. ) ;
#22257=CARTESIAN_POINT ( 'NONE',  ( 1.121324086407811338, -24.55319635012989110, 6.700000000000000178 ) ) ;
#22261=EDGE_CURVE ( 'NONE', #18339, #17250, #34031, .T. ) ;
#22271=ORIENTED_EDGE ( 'NONE', *, *, #116, .F. ) ;
#22274=CYLINDRICAL_SURFACE ( 'NONE', #30396, 0.1000000000000028644 ) ;
#22282=DIRECTION ( 'NONE',  ( 0.000000000000000000, 0.000000000000000000, 1.000000000000000000 ) ) ;
#22287=CIRCLE ( 'NONE', #40655, 0.1000000000000028644 ) ;
#22289=ORIENTED_EDGE ( 'NONE', *, *, #21151, .F. ) ;
#22292=FACE_OUTER_BOUND ( 'NONE', #16371, .T. ) ;
#22301=CIRCLE ( 'NONE', #4538, 0.1000000000000028644 ) ;
#22311=ORIENTED_EDGE ( 'NONE', *, *, #20587, .T. ) ;
#22318=CARTESIAN_POINT ( 'NONE',  ( -36.87867591359218977, -26.64985754041175525, 6.700000000000000178 ) ) ;
#22321=DIRECTION ( 'NONE',  ( -0.000000000000000000, -0.000000000000000000, 1.000000000000000000 ) ) ;
#22322=VECTOR ( 'NONE', #33407, 1000.000000000000000 ) ;
#22329=ORIENTED_EDGE ( 'NONE', *, *, #22180, .T. ) ;
#22336=ORIENTED_EDGE ( 'NONE', *, *, #34294, .T. ) ;
#22354=DIRECTION ( 'NONE',  ( 0.000000000000000000, 0.000000000000000000, 1.000000000000000000 ) ) ;
#22355=ORIENTED_EDGE ( 'NONE', *, *, #24253, .F. ) ;
#22358=ORIENTED_EDGE ( 'NONE', *, *, #40558, .F. ) ;
#22369=PLANE ( 'NONE',  #35542 ) ;
#22372=ORIENTED_EDGE ( 'NONE', *, *, #15419, .T. ) ;
#22384=ORIENTED_EDGE ( 'NONE', *, *, #36534, .T. ) ;
#22387=VECTOR ( 'NONE', #31345, 1000.000000000000000 ) ;
#22388=VERTEX_POINT ( 'NONE', #15674 ) ;
#22393=ORIENTED_EDGE ( 'NONE', *, *, #5642, .F. ) ;
#22396=DIRECTION ( 'NONE',  ( 0.000000000000000000, 0.000000000000000000, 1.000000000000000000 ) ) ;
#22403=CARTESIAN_POINT ( 'NONE',  ( -35.07867591359219972, -26.64985754041175525, 6.700000000000000178 ) ) ;
#22409=VERTEX_POINT ( 'NONE', #35447 ) ;
#22411=DIRECTION ( 'NONE',  ( 0.000000000000000000, 0.000000000000000000, 1.000000000000000000 ) ) ;
#22413=AXIS2_PLACEMENT_3D ( 'NONE', #27604, #8654, #14621 ) ;
#22418=DIRECTION ( 'NONE',  ( 1.000000000000000000, 0.000000000000000000, 0.000000000000000000 ) ) ;
#22425=DIRECTION ( 'NONE',  ( -0.000000000000000000, -0.000000000000000000, 1.000000000000000000 ) ) ;
#22427=EDGE_CURVE ( 'NONE', #19656, #32235, #26565, .T. ) ;
#22428=VECTOR ( 'NONE', #29934, 1000.000000000000000 ) ;
#22429=CARTESIAN_POINT ( 'NONE',  ( -54.01549048184568846, -30.38627270959228710, -4.152976064860135708 ) ) ;
#22434=DIRECTION ( 'NONE',  ( 1.000000000000000000, 0.000000000000000000, 0.000000000000000000 ) ) ;
#22438=DIRECTION ( 'NONE',  ( -0.000000000000000000, -0.000000000000000000, -1.000000000000000000 ) ) ;
#22444=CARTESIAN_POINT ( 'NONE',  ( -16.24874870218063450, -26.64985754041175525, 6.700000000000000178 ) ) ;
#22457=AXIS2_PLACEMENT_3D ( 'NONE', #1648, #1053, #14184 ) ;
#22466=CARTESIAN_POINT ( 'NONE',  ( -32.34874870218063592, -26.64985754041175525, 6.700000000000000178 ) ) ;
#22467=FACE_OUTER_BOUND ( 'NONE', #13989, .T. ) ;
#22471=ORIENTED_EDGE ( 'NONE', *, *, #34855, .T. ) ;
#22484=FACE_BOUND ( 'NONE', #17456, .T. ) ;
#22488=EDGE_LOOP ( 'NONE', ( #29171, #405, #24713, #14404 ) ) ;
#22502=ORIENTED_EDGE ( 'NONE', *, *, #19307, .F. ) ;
#22504=VECTOR ( 'NONE', #36798, 1000.000000000000000 ) ;
#22514=CARTESIAN_POINT ( 'NONE',  ( -0.4487487021806388365, -26.64985754041175525, 6.800000000000000711 ) ) ;
#22516=LINE ( 'NONE', #31774, #32532 ) ;
#22520=EDGE_CURVE ( 'NONE', #26610, #9487, #18045, .T. ) ;
#22525=ORIENTED_EDGE ( 'NONE', *, *, #33683, .F. ) ;
#22526=CARTESIAN_POINT ( 'NONE',  ( -12.87867591359218977, -26.64985754041175525, 6.700000000000000178 ) ) ;
#22529=ORIENTED_EDGE ( 'NONE', *, *, #35482, .T. ) ;
#22536=PLANE ( 'NONE',  #36329 ) ;
#22539=DIRECTION ( 'NONE',  ( 0.000000000000000000, 0.000000000000000000, 1.000000000000000000 ) ) ;
#22549=DIRECTION ( 'NONE',  ( 1.000000000000000000, 0.000000000000000000, 0.000000000000000000 ) ) ;
#22551=CARTESIAN_POINT ( 'NONE',  ( 1.551251297819356001, -26.64985754041175525, 6.700000000000000178 ) ) ;
#22553=CARTESIAN_POINT ( 'NONE',  ( -42.83131703149249603, -29.56993018339339940, 6.800000000000000711 ) ) ;
#22566=AXIS2_PLACEMENT_3D ( 'NONE', #28901, #38350, #3608 ) ;
#22570=CARTESIAN_POINT ( 'NONE',  ( -41.07867591359219972, -24.55319635012989110, 6.700000000000000178 ) ) ;
#22571=VERTEX_POINT ( 'NONE', #11095 ) ;
#22583=ORIENTED_EDGE ( 'NONE', *, *, #12068, .F. ) ;
#22585=ORIENTED_EDGE ( 'NONE', *, *, #17741, .T. ) ;
#22594=DIRECTION ( 'NONE',  ( 0.000000000000000000, 0.000000000000000000, 1.000000000000000000 ) ) ;
#22601=CARTESIAN_POINT ( 'NONE',  ( -13.07867591359219617, -24.55319635012989110, 6.700000000000000178 ) ) ;
#22602=CIRCLE ( 'NONE', #34455, 0.1000000000000028644 ) ;
#22612=DIRECTION ( 'NONE',  ( -0.000000000000000000, -0.000000000000000000, 1.000000000000000000 ) ) ;
#22631=ORIENTED_EDGE ( 'NONE', *, *, #38344, .F. ) ;
#22633=VECTOR ( 'NONE', #10943, 1000.000000000000000 ) ;
#22635=ORIENTED_EDGE ( 'NONE', *, *, #34210, .F. ) ;
#22640=ORIENTED_EDGE ( 'NONE', *, *, #11139, .F. ) ;
#22641=AXIS2_PLACEMENT_3D ( 'NONE', #5653, #25001, #18191 ) ;
#22646=DIRECTION ( 'NONE',  ( 0.000000000000000000, 1.000000000000000000, 0.000000000000000000 ) ) ;
#22651=ORIENTED_EDGE ( 'NONE', *, *, #27748, .T. ) ;
#22662=EDGE_CURVE ( 'NONE', #28211, #4500, #5141, .T. ) ;
#22663=VECTOR ( 'NONE', #10140, 1000.000000000000000 ) ;
#22669=DIRECTION ( 'NONE',  ( -0.000000000000000000, -1.000000000000000000, -0.000000000000000000 ) ) ;
#22670=ORIENTED_EDGE ( 'NONE', *, *, #22180, .F. ) ;
#22673=DIRECTION ( 'NONE',  ( 1.000000000000000000, 0.000000000000000000, 0.000000000000000000 ) ) ;
#22675=EDGE_CURVE ( 'NONE', #2698, #2900, #36635, .T. ) ;
#22679=DIRECTION ( 'NONE',  ( -0.000000000000000000, -0.000000000000000000, 1.000000000000000000 ) ) ;
#22683=( NAMED_UNIT ( * ) PLANE_ANGLE_UNIT ( ) SI_UNIT ( $, .RADIAN. ) );
#22685=FACE_BOUND ( 'NONE', #15360, .T. ) ;
#22686=DIRECTION ( 'NONE',  ( 1.000000000000000000, 0.000000000000000000, 0.000000000000000000 ) ) ;
#22687=VERTEX_POINT ( 'NONE', #37035 ) ;
#22706=EDGE_CURVE ( 'NONE', #31748, #35240, #30257, .T. ) ;
#22721=DIRECTION ( 'NONE',  ( 1.000000000000000000, 0.000000000000000000, 0.000000000000000000 ) ) ;
#22722=AXIS2_PLACEMENT_3D ( 'NONE', #24275, #21402, #23852 ) ;
#22723=EDGE_LOOP ( 'NONE', ( #34707, #11135, #28347, #36235 ) ) ;
#22727=VECTOR ( 'NONE', #25901, 1000.000000000000000 ) ;
#22729=ORIENTED_EDGE ( 'NONE', *, *, #24487, .F. ) ;
#22745=LINE ( 'NONE', #29517, #12490 ) ;
#22748=EDGE_CURVE ( 'NONE', #26805, #13108, #5755, .T. ) ;
#22749=CARTESIAN_POINT ( 'NONE',  ( 3.551251297819357777, -26.64985754041175525, 6.800000000000000711 ) ) ;
#22750=AXIS2_PLACEMENT_3D ( 'NONE', #19831, #7069, #38349 ) ;
#22758=DIRECTION ( 'NONE',  ( -0.000000000000000000, -1.000000000000000000, -0.000000000000000000 ) ) ;
#22761=DIRECTION ( 'NONE',  ( 1.000000000000000000, 0.000000000000000000, 0.000000000000000000 ) ) ;
#22767=CARTESIAN_POINT ( 'NONE',  ( -16.34874870218063592, -25.49307895267003587, 6.800000000000000711 ) ) ;
#22769=LINE ( 'NONE', #7501, #18732 ) ;
#22775=VERTEX_POINT ( 'NONE', #33568 ) ;
#22779=CARTESIAN_POINT ( 'NONE',  ( 3.751251297819363728, -26.64985754041175525, 6.700000000000000178 ) ) ;
#22787=VERTEX_POINT ( 'NONE', #30464 ) ;
#22797=ORIENTED_EDGE ( 'NONE', *, *, #26701, .F. ) ;
#22801=EDGE_CURVE ( 'NONE', #16705, #14656, #40125, .T. ) ;
#22803=DIRECTION ( 'NONE',  ( -0.000000000000000000, -0.000000000000000000, 1.000000000000000000 ) ) ;
#22804=EDGE_CURVE ( 'NONE', #37085, #5530, #35150, .T. ) ;
#22806=CARTESIAN_POINT ( 'NONE',  ( 6.921324086407803833, -24.55319635012989110, 6.700000000000000178 ) ) ;
#22807=CARTESIAN_POINT ( 'NONE',  ( 11.65737507970504439, -32.06993018339339585, 6.800000000000000711 ) ) ;
#22816=DIRECTION ( 'NONE',  ( 1.000000000000000000, 0.000000000000000000, 0.000000000000000000 ) ) ;
#22817=LINE ( 'NONE', #32483, #5594 ) ;
#22818=AXIS2_PLACEMENT_3D ( 'NONE', #13210, #3018, #3974 ) ;
#22821=CARTESIAN_POINT ( 'NONE',  ( -17.07867591359219617, -26.64985754041175525, 6.700000000000000178 ) ) ;
#22823=ORIENTED_EDGE ( 'NONE', *, *, #3800, .F. ) ;
#22828=DIRECTION ( 'NONE',  ( -0.000000000000000000, -0.000000000000000000, 1.000000000000000000 ) ) ;
#22834=CARTESIAN_POINT ( 'NONE',  ( -8.448748702180639114, -26.64985754041175525, 6.700000000000000178 ) ) ;
#22838=AXIS2_PLACEMENT_3D ( 'NONE', #38837, #11585, #30560 ) ;
#22846=ORIENTED_EDGE ( 'NONE', *, *, #13776, .F. ) ;
#22852=CARTESIAN_POINT ( 'NONE',  ( -8.248748702180632719, -25.49307895267003587, 6.800000000000000711 ) ) ;
#22860=DIRECTION ( 'NONE',  ( 1.000000000000000000, 0.000000000000000000, 0.000000000000000000 ) ) ;
#22866=VECTOR ( 'NONE', #30365, 1000.000000000000000 ) ;
#22867=DIRECTION ( 'NONE',  ( -0.000000000000000000, -1.000000000000000000, -0.000000000000000000 ) ) ;
#22869=ORIENTED_EDGE ( 'NONE', *, *, #24214, .F. ) ;
#22875=ORIENTED_EDGE ( 'NONE', *, *, #40292, .T. ) ;
#22883=VERTEX_POINT ( 'NONE', #13497 ) ;
#22885=ADVANCED_FACE ( 'NONE', ( #10199 ), #35742, .F. ) ;
#22886=VECTOR ( 'NONE', #578, 1000.000000000000000 ) ;
#22887=DIRECTION ( 'NONE',  ( 0.000000000000000000, 0.000000000000000000, 1.000000000000000000 ) ) ;
#22893=VECTOR ( 'NONE', #25951, 1000.000000000000000 ) ;
#22899=LINE ( 'NONE', #32778, #8997 ) ;
#22906=LINE ( 'NONE', #26594, #107 ) ;
#22910=PLANE ( 'NONE',  #16067 ) ;
#22919=DIRECTION ( 'NONE',  ( -0.000000000000000000, -1.000000000000000000, -0.000000000000000000 ) ) ;
#22921=VECTOR ( 'NONE', #20292, 1000.000000000000000 ) ;
#22924=CARTESIAN_POINT ( 'NONE',  ( -0.4487487021806388365, -26.64985754041175525, 6.700000000000000178 ) ) ;
#22942=ORIENTED_EDGE ( 'NONE', *, *, #4539, .T. ) ;
#22959=CARTESIAN_POINT ( 'NONE',  ( -40.44874870218063734, -26.64985754041175525, 6.700000000000000178 ) ) ;
#22965=DIRECTION ( 'NONE',  ( 1.000000000000000000, 0.000000000000000000, 0.000000000000000000 ) ) ;
#22966=EDGE_CURVE ( 'NONE', #33369, #38905, #32058, .T. ) ;
#22974=ORIENTED_EDGE ( 'NONE', *, *, #6814, .T. ) ;
#22982=EDGE_CURVE ( 'NONE', #2693, #34412, #7566, .T. ) ;
#22992=CARTESIAN_POINT ( 'NONE',  ( -27.07867591359219972, -26.64985754041175525, 6.700000000000000178 ) ) ;
#22994=ADVANCED_BREP_SHAPE_REPRESENTATION ( '', ( #26090, #30744 ), #40552 ) ;
#22998=CARTESIAN_POINT ( 'NONE',  ( -0.4487487021806388365, -25.49307895267003587, 6.700000000000000178 ) ) ;
#23001=DIRECTION ( 'NONE',  ( 0.000000000000000000, 0.000000000000000000, 1.000000000000000000 ) ) ;
#23012=ADVANCED_FACE ( 'NONE', ( #26467 ), #36141, .F. ) ;
#23014=DIRECTION ( 'NONE',  ( 1.000000000000000000, 0.000000000000000000, 0.000000000000000000 ) ) ;
#23016=VERTEX_POINT ( 'NONE', #39205 ) ;
#23018=ADVANCED_FACE ( 'NONE', ( #14295 ), #36740, .F. ) ;
#23022=VECTOR ( 'NONE', #5872, 1000.000000000000000 ) ;
#23026=CARTESIAN_POINT ( 'NONE',  ( -4.248748702180636272, -26.64985754041175525, 6.800000000000000711 ) ) ;
#23027=VERTEX_POINT ( 'NONE', #23576 ) ;
#23029=ADVANCED_FACE ( 'NONE', ( #30580 ), #33258, .F. ) ;
#23030=ORIENTED_EDGE ( 'NONE', *, *, #35718, .F. ) ;
#23035=CARTESIAN_POINT ( 'NONE',  ( 3.551251297819357777, -26.64985754041175525, 6.800000000000000711 ) ) ;
#23043=CARTESIAN_POINT ( 'NONE',  ( -22.24874870218063450, -25.49307895267003587, 6.700000000000000178 ) ) ;
#23052=CIRCLE ( 'NONE', #22413, 0.1000000000000028644 ) ;
#23063=FACE_OUTER_BOUND ( 'NONE', #23672, .T. ) ;
#23066=CARTESIAN_POINT ( 'NONE',  ( 7.121324086407810228, -24.55319635012989110, 6.800000000000000711 ) ) ;
#23067=AXIS2_PLACEMENT_3D ( 'NONE', #6202, #12982, #31322 ) ;
#23068=DIRECTION ( 'NONE',  ( 1.000000000000000000, 0.000000000000000000, 0.000000000000000000 ) ) ;
#23072=VERTEX_POINT ( 'NONE', #21106 ) ;
#23077=EDGE_CURVE ( 'NONE', #14763, #32941, #10846, .T. ) ;
#23079=CIRCLE ( 'NONE', #4052, 0.1000000000000028644 ) ;
#23080=ADVANCED_FACE ( 'NONE', ( #38996 ), #7721, .F. ) ;
#23082=ORIENTED_EDGE ( 'NONE', *, *, #9858, .F. ) ;
#23089=ORIENTED_EDGE ( 'NONE', *, *, #38389, .T. ) ;
#23092=DIRECTION ( 'NONE',  ( 1.000000000000000000, 0.000000000000000000, 0.000000000000000000 ) ) ;
#23108=VECTOR ( 'NONE', #33765, 1000.000000000000000 ) ;
#23114=DIRECTION ( 'NONE',  ( -1.000000000000000000, 0.000000000000000000, 0.000000000000000000 ) ) ;
#23121=VERTEX_POINT ( 'NONE', #20271 ) ;
#23128=CYLINDRICAL_SURFACE ( 'NONE', #22566, 0.1000000000000028644 ) ;
#23129=EDGE_LOOP ( 'NONE', ( #5330, #6481, #38895, #34720 ) ) ;
#23142=CARTESIAN_POINT ( 'NONE',  ( -26.87867591359219333, -26.64985754041175525, 6.700000000000000178 ) ) ;
#23159=EDGE_CURVE ( 'NONE', #29402, #39054, #29746, .T. ) ;
#23160=FACE_OUTER_BOUND ( 'NONE', #39171, .T. ) ;
#23161=EDGE_CURVE ( 'NONE', #29464, #9354, #11430, .T. ) ;
#23163=LINE ( 'NONE', #17711, #22322 ) ;
#23174=DIRECTION ( 'NONE',  ( -0.000000000000000000, -0.000000000000000000, 1.000000000000000000 ) ) ;
#23183=EDGE_CURVE ( 'NONE', #30629, #16055, #40584, .T. ) ;
#23187=CARTESIAN_POINT ( 'NONE',  ( 1.021324086407808585, -24.55319635012989110, 6.800000000000000711 ) ) ;
#23191=AXIS2_PLACEMENT_3D ( 'NONE', #29550, #23174, #32257 ) ;
#23196=CARTESIAN_POINT ( 'NONE',  ( -13.07867591359219617, -26.64985754041175525, 6.700000000000000178 ) ) ;
#23210=LINE ( 'NONE', #29583, #30050 ) ;
#23211=EDGE_LOOP ( 'NONE', ( #37148, #27531, #3952, #24105 ) ) ;
#23214=VECTOR ( 'NONE', #11611, 1000.000000000000000 ) ;
#23215=DIRECTION ( 'NONE',  ( -0.000000000000000000, -0.000000000000000000, 1.000000000000000000 ) ) ;
#23224=DIRECTION ( 'NONE',  ( 1.241493069327139093E-16, -1.000000000000000000, 0.000000000000000000 ) ) ;
#23225=EDGE_LOOP ( 'NONE', ( #27612, #13388, #60, #28375 ) ) ;
#23228=ORIENTED_EDGE ( 'NONE', *, *, #37217, .T. ) ;
#23230=LINE ( 'NONE', #4305, #36514 ) ;
#23238=CARTESIAN_POINT ( 'NONE',  ( -16.87867591359218977, -26.64985754041175525, 6.800000000000000711 ) ) ;
#23240=DIRECTION ( 'NONE',  ( 0.000000000000000000, 0.000000000000000000, 1.000000000000000000 ) ) ;
#23242=EDGE_LOOP ( 'NONE', ( #1237, #450, #28272, #30492 ) ) ;
#23253=CARTESIAN_POINT ( 'NONE',  ( -8.248748702180632719, -26.64985754041175525, 6.800000000000000711 ) ) ;
#23254=ORIENTED_EDGE ( 'NONE', *, *, #25814, .T. ) ;
#23262=CARTESIAN_POINT ( 'NONE',  ( -16.24874870218063450, -25.49307895267003587, 6.700000000000000178 ) ) ;
#23264=ORIENTED_EDGE ( 'NONE', *, *, #36534, .F. ) ;
#23266=CARTESIAN_POINT ( 'NONE',  ( -0.9786759135921931918, -26.64985754041175525, 6.700000000000000178 ) ) ;
#23274=VECTOR ( 'NONE', #15463, 1000.000000000000000 ) ;
#23279=ORIENTED_EDGE ( 'NONE', *, *, #1739, .F. ) ;
#23282=CARTESIAN_POINT ( 'NONE',  ( 6.921324086407803833, -26.64985754041175525, 6.700000000000000178 ) ) ;
#23285=CARTESIAN_POINT ( 'NONE',  ( -32.44874870218063734, -26.64985754041175525, 6.700000000000000178 ) ) ;
#23289=CARTESIAN_POINT ( 'NONE',  ( -8.348748702180635917, -25.49307895267003587, 6.700000000000000178 ) ) ;
#23293=DIRECTION ( 'NONE',  ( 1.000000000000000000, 0.000000000000000000, 0.000000000000000000 ) ) ;
#23294=DIRECTION ( 'NONE',  ( 1.000000000000000000, 0.000000000000000000, 0.000000000000000000 ) ) ;
#23302=VECTOR ( 'NONE', #27652, 1000.000000000000000 ) ;
#23305=DIRECTION ( 'NONE',  ( 1.000000000000000000, -0.000000000000000000, 0.000000000000000000 ) ) ;
#23308=CARTESIAN_POINT ( 'NONE',  ( -38.97867591359219119, -26.64985754041175525, 6.800000000000000711 ) ) ;
#23311=CARTESIAN_POINT ( 'NONE',  ( -15.07867591359219439, -24.55319635012989110, 6.700000000000000178 ) ) ;
#23312=LINE ( 'NONE', #1699, #34934 ) ;
#23313=ORIENTED_EDGE ( 'NONE', *, *, #32984, .T. ) ;
#23320=VERTEX_POINT ( 'NONE', #38310 ) ;
#23329=VECTOR ( 'NONE', #39925, 1000.000000000000000 ) ;
#23331=CYLINDRICAL_SURFACE ( 'NONE', #37700, 0.1000000000000028644 ) ;
#23338=VERTEX_POINT ( 'NONE', #28861 ) ;
#23341=DIRECTION ( 'NONE',  ( -0.000000000000000000, -0.000000000000000000, 1.000000000000000000 ) ) ;
#23349=VECTOR ( 'NONE', #28364, 1000.000000000000000 ) ;
#23350=LINE ( 'NONE', #22959, #38739 ) ;
#23351=EDGE_CURVE ( 'NONE', #9750, #17194, #13205, .T. ) ;
#23352=ORIENTED_EDGE ( 'NONE', *, *, #16462, .F. ) ;
#23355=VECTOR ( 'NONE', #89, 1000.000000000000000 ) ;
#23356=DIRECTION ( 'NONE',  ( 0.000000000000000000, 0.000000000000000000, -1.000000000000000000 ) ) ;
#23358=CARTESIAN_POINT ( 'NONE',  ( -28.34874870218063947, -26.64985754041175525, 6.800000000000000711 ) ) ;
#23360=CARTESIAN_POINT ( 'NONE',  ( -24.34874870218063592, -26.64985754041175525, 6.700000000000000178 ) ) ;
#23369=EDGE_CURVE ( 'NONE', #2698, #10291, #33807, .T. ) ;
#23374=AXIS2_PLACEMENT_3D ( 'NONE', #3494, #6761, #16807 ) ;
#23381=VECTOR ( 'NONE', #13727, 1000.000000000000000 ) ;
#23388=ORIENTED_EDGE ( 'NONE', *, *, #14342, .T. ) ;
#23400=CARTESIAN_POINT ( 'NONE',  ( -2.978675913592195190, -26.64985754041175525, 6.700000000000000178 ) ) ;
#23402=AXIS2_PLACEMENT_3D ( 'NONE', #3243, #36968, #12464 ) ;
#23403=AXIS2_PLACEMENT_3D ( 'NONE', #29401, #35788, #6971 ) ;
#23405=CARTESIAN_POINT ( 'NONE',  ( 5.021324086407805254, -24.55319635012989110, 6.700000000000000178 ) ) ;
#23412=ORIENTED_EDGE ( 'NONE', *, *, #29011, .F. ) ;
#23419=ORIENTED_EDGE ( 'NONE', *, *, #23159, .T. ) ;
#23427=ADVANCED_FACE ( 'NONE', ( #11510 ), #11302, .T. ) ;
#23435=CYLINDRICAL_SURFACE ( 'NONE', #11083, 0.1000000000000028644 ) ;
#23437=AXIS2_PLACEMENT_3D ( 'NONE', #27719, #18037, #12058 ) ;
#23441=DIRECTION ( 'NONE',  ( 0.000000000000000000, 0.000000000000000000, 1.000000000000000000 ) ) ;
#23442=AXIS2_PLACEMENT_3D ( 'NONE', #31969, #10319, #16685 ) ;
#23445=EDGE_CURVE ( 'NONE', #40382, #33795, #17690, .T. ) ;
#23446=DIRECTION ( 'NONE',  ( 1.000000000000000000, 0.000000000000000000, 0.000000000000000000 ) ) ;
#23450=EDGE_LOOP ( 'NONE', ( #32935, #8464, #9882, #856 ) ) ;
#23458=ORIENTED_EDGE ( 'NONE', *, *, #33048, .F. ) ;
#23462=AXIS2_PLACEMENT_3D ( 'NONE', #28663, #6435, #469 ) ;
#23467=CIRCLE ( 'NONE', #4415, 0.1000000000000028644 ) ;
#23469=CIRCLE ( 'NONE', #19537, 0.1000000000000028644 ) ;
#23470=EDGE_CURVE ( 'NONE', #37250, #13245, #19337, .T. ) ;
#23476=ORIENTED_EDGE ( 'NONE', *, *, #8628, .T. ) ;
#23481=EDGE_CURVE ( 'NONE', #11841, #8794, #10910, .T. ) ;
#23486=CARTESIAN_POINT ( 'NONE',  ( -20.34874870218063947, -26.64985754041175525, 6.700000000000000178 ) ) ;
#23490=ORIENTED_EDGE ( 'NONE', *, *, #32049, .F. ) ;
#23502=FACE_OUTER_BOUND ( 'NONE', #12725, .T. ) ;
#23508=CARTESIAN_POINT ( 'NONE',  ( 11.65737507970504616, -38.28842912540938670, 6.800000000000000711 ) ) ;
#23515=FACE_OUTER_BOUND ( 'NONE', #19278, .T. ) ;
#23528=CARTESIAN_POINT ( 'NONE',  ( 3.021324086407803478, -24.55319635012989110, 6.700000000000000178 ) ) ;
#23536=EDGE_CURVE ( 'NONE', #26273, #29514, #18024, .T. ) ;
#23537=DIRECTION ( 'NONE',  ( -1.000000000000000000, 0.000000000000000000, 0.000000000000000000 ) ) ;
#23556=ORIENTED_EDGE ( 'NONE', *, *, #30019, .F. ) ;
#23562=PLANE ( 'NONE',  #7255 ) ;
#23564=CARTESIAN_POINT ( 'NONE',  ( -29.07867591359219617, -24.55319635012989110, 6.700000000000000178 ) ) ;
#23565=ORIENTED_EDGE ( 'NONE', *, *, #26189, .T. ) ;
#23571=CARTESIAN_POINT ( 'NONE',  ( -14.97867591359219119, -24.55319635012989110, 6.700000000000000178 ) ) ;
#23576=CARTESIAN_POINT ( 'NONE',  ( -10.44874870218064089, -26.64985754041175525, 6.700000000000000178 ) ) ;
#23577=ADVANCED_FACE ( 'NONE', ( #21620 ), #6385, .F. ) ;
#23598=DIRECTION ( 'NONE',  ( 1.000000000000000000, 0.000000000000000000, 0.000000000000000000 ) ) ;
#23600=DIRECTION ( 'NONE',  ( -0.000000000000000000, -0.000000000000000000, 1.000000000000000000 ) ) ;
#23602=EDGE_CURVE ( 'NONE', #1810, #12640, #25924, .T. ) ;
#23607=ADVANCED_FACE ( 'NONE', ( #34200 ), #28398, .F. ) ;
#23612=CARTESIAN_POINT ( 'NONE',  ( -21.07867591359219617, -26.64985754041175525, 6.800000000000000711 ) ) ;
#23620=ADVANCED_FACE ( 'NONE', ( #3121 ), #40136, .F. ) ;
#23646=CARTESIAN_POINT ( 'NONE',  ( -14.97867591359219119, -24.55319635012989110, 6.700000000000000178 ) ) ;
#23648=EDGE_CURVE ( 'NONE', #3677, #10008, #37251, .T. ) ;
#23649=DIRECTION ( 'NONE',  ( 0.000000000000000000, 0.000000000000000000, 1.000000000000000000 ) ) ;
#23652=EDGE_CURVE ( 'NONE', #12335, #20068, #37745, .T. ) ;
#23654=EDGE_CURVE ( 'NONE', #35786, #212, #35804, .T. ) ;
#23664=FACE_OUTER_BOUND ( 'NONE', #25351, .T. ) ;
#23667=EDGE_LOOP ( 'NONE', ( #6230, #15129, #3668, #19451 ) ) ;
#23672=EDGE_LOOP ( 'NONE', ( #20663, #18474, #8819, #2564 ) ) ;
#23675=CIRCLE ( 'NONE', #24994, 0.1000000000000028644 ) ;
#23680=CARTESIAN_POINT ( 'NONE',  ( -9.078675913592196167, -26.64985754041175525, 6.800000000000000711 ) ) ;
#23687=PLANE ( 'NONE',  #10428 ) ;
#23696=DIRECTION ( 'NONE',  ( 0.000000000000000000, 0.000000000000000000, -1.000000000000000000 ) ) ;
#23702=DIRECTION ( 'NONE',  ( 1.000000000000000000, 0.000000000000000000, 0.000000000000000000 ) ) ;
#23705=AXIS2_PLACEMENT_3D ( 'NONE', #17109, #32791, #13425 ) ;
#23711=ORIENTED_EDGE ( 'NONE', *, *, #38016, .T. ) ;
#23713=LINE ( 'NONE', #4987, #4863 ) ;
#23724=ORIENTED_EDGE ( 'NONE', *, *, #23654, .F. ) ;
#23726=AXIS2_PLACEMENT_3D ( 'NONE', #23289, #35859, #4563 ) ;
#23732=CIRCLE ( 'NONE', #34301, 0.1000000000000028644 ) ;
#23737=DIRECTION ( 'NONE',  ( 0.000000000000000000, 0.000000000000000000, 1.000000000000000000 ) ) ;
#23743=CYLINDRICAL_SURFACE ( 'NONE', #37418, 0.1000000000000028644 ) ;
#23748=CARTESIAN_POINT ( 'NONE',  ( -34.24874870218063450, -26.64985754041175525, 6.700000000000000178 ) ) ;
#23754=CARTESIAN_POINT ( 'NONE',  ( -10.24874870218063450, -26.64985754041175525, 6.700000000000000178 ) ) ;
#23756=VERTEX_POINT ( 'NONE', #4893 ) ;
#23757=LINE ( 'NONE', #8097, #39631 ) ;
#23767=ORIENTED_EDGE ( 'NONE', *, *, #37500, .F. ) ;
#23771=DIRECTION ( 'NONE',  ( 1.000000000000000000, 0.000000000000000000, -0.000000000000000000 ) ) ;
#23781=CYLINDRICAL_SURFACE ( 'NONE', #17522, 0.1000000000000028644 ) ;
#23782=DIRECTION ( 'NONE',  ( 1.000000000000000000, 0.000000000000000000, 0.000000000000000000 ) ) ;
#23790=EDGE_CURVE ( 'NONE', #31323, #22687, #36596, .T. ) ;
#23794=CARTESIAN_POINT ( 'NONE',  ( -24.34874870218063592, -25.49307895267003587, 6.700000000000000178 ) ) ;
#23797=CARTESIAN_POINT ( 'NONE',  ( -32.44874870218063734, -26.64985754041175525, 6.800000000000000711 ) ) ;
#23817=DIRECTION ( 'NONE',  ( -0.000000000000000000, -0.000000000000000000, 1.000000000000000000 ) ) ;
#23819=DIRECTION ( 'NONE',  ( 0.000000000000000000, 0.000000000000000000, 1.000000000000000000 ) ) ;
#23824=ORIENTED_EDGE ( 'NONE', *, *, #17451, .F. ) ;
#23826=CARTESIAN_POINT ( 'NONE',  ( 3.021324086407803478, -24.55319635012989110, 6.700000000000000178 ) ) ;
#23832=DIRECTION ( 'NONE',  ( 1.000000000000000000, -0.000000000000000000, 0.000000000000000000 ) ) ;
#23833=AXIS2_PLACEMENT_3D ( 'NONE', #36955, #1985, #23771 ) ;
#23840=FACE_OUTER_BOUND ( 'NONE', #16171, .T. ) ;
#23843=VECTOR ( 'NONE', #36396, 1000.000000000000000 ) ;
#23850=CARTESIAN_POINT ( 'NONE',  ( -18.44874870218064089, -26.64985754041175525, 6.700000000000000178 ) ) ;
#23852=DIRECTION ( 'NONE',  ( 1.000000000000000000, 0.000000000000000000, 0.000000000000000000 ) ) ;
#23853=ORIENTED_EDGE ( 'NONE', *, *, #28785, .F. ) ;
#23861=CARTESIAN_POINT ( 'NONE',  ( -14.44874870218064089, -26.64985754041175525, 6.700000000000000178 ) ) ;
#23866=ORIENTED_EDGE ( 'NONE', *, *, #30982, .F. ) ;
#23873=VERTEX_POINT ( 'NONE', #7973 ) ;
#23875=ADVANCED_FACE ( 'NONE', ( #33111 ), #30010, .F. ) ;
#23877=DIRECTION ( 'NONE',  ( -0.000000000000000000, -0.000000000000000000, 1.000000000000000000 ) ) ;
#23886=CYLINDRICAL_SURFACE ( 'NONE', #27064, 0.1000000000000028644 ) ;
#23888=CARTESIAN_POINT ( 'NONE',  ( -8.448748702180639114, -26.64985754041175525, 6.700000000000000178 ) ) ;
#23889=EDGE_CURVE ( 'NONE', #40280, #35786, #21575, .T. ) ;
#23895=VECTOR ( 'NONE', #26726, 1000.000000000000000 ) ;
#23896=CARTESIAN_POINT ( 'NONE',  ( -2.448748702180640446, -25.49307895267003587, 6.800000000000000711 ) ) ;
#23897=ORIENTED_EDGE ( 'NONE', *, *, #27186, .F. ) ;
#23907=LINE ( 'NONE', #8253, #23981 ) ;
#23910=DIRECTION ( 'NONE',  ( -0.000000000000000000, -0.000000000000000000, 1.000000000000000000 ) ) ;
#23915=AXIS2_PLACEMENT_3D ( 'NONE', #21144, #5490, #11643 ) ;
#23922=ADVANCED_FACE ( 'NONE', ( #27534 ), #40283, .F. ) ;
#23926=ORIENTED_EDGE ( 'NONE', *, *, #35718, .T. ) ;
#23928=AXIS2_PLACEMENT_3D ( 'NONE', #13848, #7869, #11340 ) ;
#23935=CARTESIAN_POINT ( 'NONE',  ( -10.97867591359219475, -24.55319635012989110, 6.700000000000000178 ) ) ;
#23945=DIRECTION ( 'NONE',  ( -0.000000000000000000, -0.000000000000000000, 1.000000000000000000 ) ) ;
#23949=VECTOR ( 'NONE', #35890, 1000.000000000000000 ) ;
#23950=FACE_OUTER_BOUND ( 'NONE', #16936, .T. ) ;
#23971=EDGE_CURVE ( 'NONE', #30400, #39064, #27469, .T. ) ;
#23973=LINE ( 'NONE', #33062, #15304 ) ;
#23974=AXIS2_PLACEMENT_3D ( 'NONE', #2777, #15303, #40406 ) ;
#23976=CARTESIAN_POINT ( 'NONE',  ( -6.448748702180637338, -25.49307895267003587, 6.700000000000000178 ) ) ;
#23981=VECTOR ( 'NONE', #5191, 1000.000000000000000 ) ;
#23984=EDGE_CURVE ( 'NONE', #33558, #26758, #17777, .T. ) ;
#23985=FACE_OUTER_BOUND ( 'NONE', #15932, .T. ) ;
#23986=FACE_OUTER_BOUND ( 'NONE', #40290, .T. ) ;
#23989=CARTESIAN_POINT ( 'NONE',  ( -3.078675913592197944, -24.55319635012989110, 6.700000000000000178 ) ) ;
#23992=CARTESIAN_POINT ( 'NONE',  ( -12.24874870218063627, -26.64985754041175525, 6.700000000000000178 ) ) ;
#23998=FACE_OUTER_BOUND ( 'NONE', #40319, .T. ) ;
#24005=VECTOR ( 'NONE', #4076, 1000.000000000000000 ) ;
#24007=ORIENTED_EDGE ( 'NONE', *, *, #13901, .T. ) ;
#24019=ADVANCED_FACE ( 'NONE', ( #1554 ), #17171, .F. ) ;
#24025=DIRECTION ( 'NONE',  ( 0.000000000000000000, 0.000000000000000000, 1.000000000000000000 ) ) ;
#24030=AXIS2_PLACEMENT_3D ( 'NONE', #27096, #5076, #33293 ) ;
#24032=CIRCLE ( 'NONE', #22750, 0.1000000000000028644 ) ;
#24038=FACE_OUTER_BOUND ( 'NONE', #27887, .T. ) ;
#24039=EDGE_LOOP ( 'NONE', ( #24892, #19749, #19280, #12941 ) ) ;
#24041=VECTOR ( 'NONE', #10719, 1000.000000000000000 ) ;
#24047=DIRECTION ( 'NONE',  ( -0.000000000000000000, -0.000000000000000000, 1.000000000000000000 ) ) ;
#24060=DIRECTION ( 'NONE',  ( 1.000000000000000000, 0.000000000000000000, 0.000000000000000000 ) ) ;
#24066=VERTEX_POINT ( 'NONE', #11191 ) ;
#24067=DIRECTION ( 'NONE',  ( -0.000000000000000000, -0.000000000000000000, 1.000000000000000000 ) ) ;
#24075=EDGE_LOOP ( 'NONE', ( #37134, #19691, #17113, #19686 ) ) ;
#24076=AXIS2_PLACEMENT_3D ( 'NONE', #11309, #10915, #26579 ) ;
#24077=CARTESIAN_POINT ( 'NONE',  ( 1.121324086407811338, -26.64985754041175525, 6.800000000000000711 ) ) ;
#24079=DIRECTION ( 'NONE',  ( 0.000000000000000000, 0.000000000000000000, 1.000000000000000000 ) ) ;
#24083=DIRECTION ( 'NONE',  ( -0.000000000000000000, -0.000000000000000000, 1.000000000000000000 ) ) ;
#24084=DIRECTION ( 'NONE',  ( 0.000000000000000000, 0.000000000000000000, 1.000000000000000000 ) ) ;
#24085=DIRECTION ( 'NONE',  ( 1.000000000000000000, 0.000000000000000000, -0.000000000000000000 ) ) ;
#24091=CARTESIAN_POINT ( 'NONE',  ( -34.87867591359218977, -26.64985754041175525, 6.800000000000000711 ) ) ;
#24093=CARTESIAN_POINT ( 'NONE',  ( -18.34874870218063947, -25.49307895267003587, 6.700000000000000178 ) ) ;
#24098=CIRCLE ( 'NONE', #2451, 0.1000000000000028644 ) ;
#24099=DIRECTION ( 'NONE',  ( -0.000000000000000000, -1.000000000000000000, -0.000000000000000000 ) ) ;
#24100=EDGE_CURVE ( 'NONE', #20712, #27773, #30783, .T. ) ;
#24105=ORIENTED_EDGE ( 'NONE', *, *, #1532, .T. ) ;
#24116=VERTEX_POINT ( 'NONE', #15109 ) ;
#24119=ORIENTED_EDGE ( 'NONE', *, *, #38344, .T. ) ;
#24131=AXIS2_PLACEMENT_3D ( 'NONE', #30830, #2639, #40072 ) ;
#24134=CIRCLE ( 'NONE', #3145, 0.1000000000000028644 ) ;
#24136=VECTOR ( 'NONE', #10596, 1000.000000000000000 ) ;
#24138=ORIENTED_EDGE ( 'NONE', *, *, #2167, .T. ) ;
#24144=FACE_OUTER_BOUND ( 'NONE', #19022, .T. ) ;
#24145=ORIENTED_EDGE ( 'NONE', *, *, #8628, .F. ) ;
#24147=EDGE_CURVE ( 'NONE', #32868, #31820, #27667, .T. ) ;
#24149=ORIENTED_EDGE ( 'NONE', *, *, #13729, .T. ) ;
#24151=CARTESIAN_POINT ( 'NONE',  ( -9.078675913592196167, -26.64985754041175525, 6.700000000000000178 ) ) ;
#24155=LINE ( 'NONE', #5428, #21352 ) ;
#24159=DIRECTION ( 'NONE',  ( 0.000000000000000000, 0.000000000000000000, 1.000000000000000000 ) ) ;
#24164=DIRECTION ( 'NONE',  ( 0.000000000000000000, 1.000000000000000000, 0.000000000000000000 ) ) ;
#24166=ORIENTED_EDGE ( 'NONE', *, *, #34503, .T. ) ;
#24167=EDGE_CURVE ( 'NONE', #17561, #29464, #33874, .T. ) ;
#24173=VECTOR ( 'NONE', #14738, 1000.000000000000000 ) ;
#24174=EDGE_CURVE ( 'NONE', #1835, #37531, #25252, .T. ) ;
#24185=ORIENTED_EDGE ( 'NONE', *, *, #39129, .T. ) ;
#24191=CARTESIAN_POINT ( 'NONE',  ( -0.9786759135921931918, -24.55319635012989110, 6.800000000000000711 ) ) ;
#24193=AXIS2_PLACEMENT_3D ( 'NONE', #7884, #17737, #33835 ) ;
#24202=PLANE ( 'NONE',  #7617 ) ;
#24204=DIRECTION ( 'NONE',  ( -1.000000000000000000, 0.000000000000000000, 0.000000000000000000 ) ) ;
#24214=EDGE_CURVE ( 'NONE', #36832, #4935, #2587, .T. ) ;
#24217=CARTESIAN_POINT ( 'NONE',  ( -25.07867591359219617, -24.55319635012989110, 6.700000000000000178 ) ) ;
#24221=CARTESIAN_POINT ( 'NONE',  ( -19.07867591359219972, -26.64985754041175525, 6.700000000000000178 ) ) ;
#24231=ORIENTED_EDGE ( 'NONE', *, *, #36221, .T. ) ;
#24236=LINE ( 'NONE', #36797, #36128 ) ;
#24244=DIRECTION ( 'NONE',  ( -0.000000000000000000, -0.000000000000000000, 1.000000000000000000 ) ) ;
#24247=DIRECTION ( 'NONE',  ( -0.000000000000000000, -0.000000000000000000, 1.000000000000000000 ) ) ;
#24248=ORIENTED_EDGE ( 'NONE', *, *, #4157, .T. ) ;
#24250=EDGE_CURVE ( 'NONE', #20163, #32142, #12631, .T. ) ;
#24253=EDGE_CURVE ( 'NONE', #33136, #32235, #38390, .T. ) ;
#24257=DIRECTION ( 'NONE',  ( -1.000000000000000000, 0.000000000000000000, 0.000000000000000000 ) ) ;
#24260=ADVANCED_FACE ( 'NONE', ( #6474 ), #21298, .T. ) ;
#24272=DIRECTION ( 'NONE',  ( -0.000000000000000000, -0.000000000000000000, 1.000000000000000000 ) ) ;
#24273=LINE ( 'NONE', #17877, #37574 ) ;
#24274=ORIENTED_EDGE ( 'NONE', *, *, #26030, .T. ) ;
#24275=CARTESIAN_POINT ( 'NONE',  ( -2.348748702180637693, -25.49307895267003587, 6.700000000000000178 ) ) ;
#24278=DIRECTION ( 'NONE',  ( -0.000000000000000000, -1.000000000000000000, -0.000000000000000000 ) ) ;
#24280=CARTESIAN_POINT ( 'NONE',  ( -10.44874870218064089, -25.49307895267003587, 6.700000000000000178 ) ) ;
#24281=ORIENTED_EDGE ( 'NONE', *, *, #35080, .T. ) ;
#24284=VERTEX_POINT ( 'NONE', #30985 ) ;
#24292=LINE ( 'NONE', #2912, #11221 ) ;
#24294=AXIS2_PLACEMENT_3D ( 'NONE', #32576, #19605, #32970 ) ;
#24296=ORIENTED_EDGE ( 'NONE', *, *, #20216, .F. ) ;
#24301=DIRECTION ( 'NONE',  ( -0.000000000000000000, -1.000000000000000000, -0.000000000000000000 ) ) ;
#24302=CARTESIAN_POINT ( 'NONE',  ( 1.551251297819356001, -25.49307895267003587, 6.800000000000000711 ) ) ;
#24309=CIRCLE ( 'NONE', #5900, 0.1000000000000028644 ) ;
#24323=CARTESIAN_POINT ( 'NONE',  ( 2.921324086407800280, -26.64985754041175525, 6.800000000000000711 ) ) ;
#24324=CARTESIAN_POINT ( 'NONE',  ( -10.87867591359219155, -26.64985754041175525, 6.800000000000000711 ) ) ;
#24326=LINE ( 'NONE', #15465, #13530 ) ;
#24328=VERTEX_POINT ( 'NONE', #19632 ) ;
#24334=CARTESIAN_POINT ( 'NONE',  ( -36.34874870218064302, -26.64985754041175525, 6.700000000000000178 ) ) ;
#24338=LINE ( 'NONE', #36902, #3967 ) ;
#24343=CIRCLE ( 'NONE', #27633, 0.1000000000000028644 ) ;
#24354=ORIENTED_EDGE ( 'NONE', *, *, #5402, .F. ) ;
#24355=DIRECTION ( 'NONE',  ( -0.000000000000000000, -0.000000000000000000, 1.000000000000000000 ) ) ;
#24371=ORIENTED_EDGE ( 'NONE', *, *, #37726, .T. ) ;
#24374=VECTOR ( 'NONE', #24164, 1000.000000000000000 ) ;
#24376=ORIENTED_EDGE ( 'NONE', *, *, #9115, .F. ) ;
#24384=CARTESIAN_POINT ( 'NONE',  ( -38.44874870218063734, -26.64985754041175525, 6.800000000000000711 ) ) ;
#24389=VERTEX_POINT ( 'NONE', #4401 ) ;
#24401=DIRECTION ( 'NONE',  ( 1.000000000000000000, 0.000000000000000000, 0.000000000000000000 ) ) ;
#24407=LINE ( 'NONE', #20909, #30708 ) ;
#24409=CYLINDRICAL_SURFACE ( 'NONE', #26850, 0.1000000000000028644 ) ;
#24415=AXIS2_PLACEMENT_3D ( 'NONE', #26576, #8835, #30479 ) ;
#24423=DIRECTION ( 'NONE',  ( -0.000000000000000000, -0.000000000000000000, 1.000000000000000000 ) ) ;
#24425=CARTESIAN_POINT ( 'NONE',  ( -18.97867591359219475, -24.55319635012989110, 6.800000000000000711 ) ) ;
#24426=DIRECTION ( 'NONE',  ( 1.000000000000000000, 0.000000000000000000, -0.000000000000000000 ) ) ;
#24427=VERTEX_POINT ( 'NONE', #19827 ) ;
#24429=DIRECTION ( 'NONE',  ( 0.000000000000000000, 0.000000000000000000, 1.000000000000000000 ) ) ;
#24446=ORIENTED_EDGE ( 'NONE', *, *, #23648, .T. ) ;
#24447=CARTESIAN_POINT ( 'NONE',  ( -7.078675913592194391, -26.64985754041175525, 6.700000000000000178 ) ) ;
#24448=ADVANCED_FACE ( 'NONE', ( #33616 ), #20823, .F. ) ;
#24451=LINE ( 'NONE', #36404, #20872 ) ;
#24457=DIRECTION ( 'NONE',  ( 0.000000000000000000, 1.000000000000000000, 0.000000000000000000 ) ) ;
#24462=FACE_OUTER_BOUND ( 'NONE', #24075, .T. ) ;
#24464=DIRECTION ( 'NONE',  ( 1.000000000000000000, 0.000000000000000000, 0.000000000000000000 ) ) ;
#24472=FACE_OUTER_BOUND ( 'NONE', #1020, .T. ) ;
#24473=VERTEX_POINT ( 'NONE', #5392 ) ;
#24478=ORIENTED_EDGE ( 'NONE', *, *, #2459, .T. ) ;
#24479=EDGE_LOOP ( 'NONE', ( #38654, #32330, #36398, #25963 ) ) ;
#24482=DIRECTION ( 'NONE',  ( -0.000000000000000000, -0.000000000000000000, 1.000000000000000000 ) ) ;
#24487=EDGE_CURVE ( 'NONE', #15795, #5705, #8252, .T. ) ;
#24496=EDGE_LOOP ( 'NONE', ( #5555, #2714, #5913, #15145 ) ) ;
#24503=EDGE_LOOP ( 'NONE', ( #5437, #20333, #25631, #4458 ) ) ;
#24507=DIRECTION ( 'NONE',  ( 0.000000000000000000, 0.000000000000000000, 1.000000000000000000 ) ) ;
#24508=CIRCLE ( 'NONE', #8059, 0.1000000000000028644 ) ;
#24512=CARTESIAN_POINT ( 'NONE',  ( -26.87867591359219333, -24.55319635012989110, 6.800000000000000711 ) ) ;
#24518=DIRECTION ( 'NONE',  ( 1.000000000000000000, 0.000000000000000000, 0.000000000000000000 ) ) ;
#24529=LINE ( 'NONE', #28220, #23274 ) ;
#24531=EDGE_LOOP ( 'NONE', ( #39249, #14197, #7491, #39298 ) ) ;
#24534=EDGE_LOOP ( 'NONE', ( #26636, #36342, #4546, #35122 ) ) ;
#24539=ORIENTED_EDGE ( 'NONE', *, *, #17053, .T. ) ;
#24551=EDGE_CURVE ( 'NONE', #39450, #408, #23713, .T. ) ;
#24557=DIRECTION ( 'NONE',  ( 0.000000000000000000, 1.000000000000000000, 0.000000000000000000 ) ) ;
#24562=DIRECTION ( 'NONE',  ( 1.000000000000000000, 0.000000000000000000, 0.000000000000000000 ) ) ;
#24569=DIRECTION ( 'NONE',  ( 1.000000000000000000, 0.000000000000000000, 0.000000000000000000 ) ) ;
#24573=CARTESIAN_POINT ( 'NONE',  ( -6.248748702180631831, -25.49307895267003587, 6.800000000000000711 ) ) ;
#24576=FACE_OUTER_BOUND ( 'NONE', #5663, .T. ) ;
#24582=CIRCLE ( 'NONE', #39698, 0.1000000000000028644 ) ;
#24587=DIRECTION ( 'NONE',  ( -0.000000000000000000, -0.000000000000000000, 1.000000000000000000 ) ) ;
#24588=CARTESIAN_POINT ( 'NONE',  ( -36.87867591359218977, -24.55319635012989110, 6.800000000000000711 ) ) ;
#24598=ORIENTED_EDGE ( 'NONE', *, *, #21424, .F. ) ;
#24599=DIRECTION ( 'NONE',  ( -0.000000000000000000, -0.000000000000000000, 1.000000000000000000 ) ) ;
#24600=EDGE_CURVE ( 'NONE', #6472, #5741, #21659, .T. ) ;
#24601=CARTESIAN_POINT ( 'NONE',  ( 1.021324086407808585, -26.64985754041175525, 6.700000000000000178 ) ) ;
#24602=ORIENTED_EDGE ( 'NONE', *, *, #22966, .F. ) ;
#24604=ORIENTED_EDGE ( 'NONE', *, *, #17137, .F. ) ;
#24608=AXIS2_PLACEMENT_3D ( 'NONE', #21886, #37314, #25382 ) ;
#24612=DIRECTION ( 'NONE',  ( -0.000000000000000000, -0.000000000000000000, 1.000000000000000000 ) ) ;
#24614=DIRECTION ( 'NONE',  ( 1.000000000000000000, 0.000000000000000000, 0.000000000000000000 ) ) ;
#24615=DIRECTION ( 'NONE',  ( 0.000000000000000000, 0.000000000000000000, -1.000000000000000000 ) ) ;
#24625=EDGE_CURVE ( 'NONE', #9053, #38495, #27614, .T. ) ;
#24629=DIRECTION ( 'NONE',  ( -0.000000000000000000, -0.000000000000000000, 1.000000000000000000 ) ) ;
#24631=ORIENTED_EDGE ( 'NONE', *, *, #37720, .F. ) ;
#24639=ORIENTED_EDGE ( 'NONE', *, *, #35999, .T. ) ;
#24649=EDGE_CURVE ( 'NONE', #20712, #21166, #24529, .T. ) ;
#24652=LINE ( 'NONE', #15378, #13027 ) ;
#24656=LINE ( 'NONE', #5312, #3200 ) ;
#24666=VECTOR ( 'NONE', #30287, 1000.000000000000000 ) ;
#24668=CARTESIAN_POINT ( 'NONE',  ( -5.078675913592192614, -26.64985754041175525, 6.700000000000000178 ) ) ;
#24669=DIRECTION ( 'NONE',  ( -0.000000000000000000, -0.000000000000000000, 1.000000000000000000 ) ) ;
#24671=DIRECTION ( 'NONE',  ( 0.000000000000000000, 0.000000000000000000, 1.000000000000000000 ) ) ;
#24673=ORIENTED_EDGE ( 'NONE', *, *, #30697, .T. ) ;
#24675=CARTESIAN_POINT ( 'NONE',  ( -38.97867591359219119, -26.64985754041175525, 6.700000000000000178 ) ) ;
#24684=CARTESIAN_POINT ( 'NONE',  ( -30.87867591359218977, -26.64985754041175525, 6.700000000000000178 ) ) ;
#24698=CARTESIAN_POINT ( 'NONE',  ( 0.9213240864078056092, -24.55319635012989110, 6.700000000000000178 ) ) ;
#24702=EDGE_CURVE ( 'NONE', #5611, #13148, #29400, .T. ) ;
#24704=DIRECTION ( 'NONE',  ( -1.273455763949465810E-16, 1.000000000000000000, 0.000000000000000000 ) ) ;
#24705=DIRECTION ( 'NONE',  ( 1.000000000000000000, -0.000000000000000000, 0.000000000000000000 ) ) ;
#24713=ORIENTED_EDGE ( 'NONE', *, *, #10577, .T. ) ;
#24728=ADVANCED_FACE ( 'NONE', ( #32698 ), #9902, .T. ) ;
#24731=DIRECTION ( 'NONE',  ( -0.000000000000000000, -1.000000000000000000, -0.000000000000000000 ) ) ;
#24735=AXIS2_PLACEMENT_3D ( 'NONE', #3379, #12803, #40191 ) ;
#24743=FACE_OUTER_BOUND ( 'NONE', #21214, .T. ) ;
#24757=VERTEX_POINT ( 'NONE', #19171 ) ;
#24772=CARTESIAN_POINT ( 'NONE',  ( 3.021324086407803478, -26.64985754041175525, 6.700000000000000178 ) ) ;
#24777=DIRECTION ( 'NONE',  ( 0.000000000000000000, 0.000000000000000000, 1.000000000000000000 ) ) ;
#24784=FACE_OUTER_BOUND ( 'NONE', #35197, .T. ) ;
#24794=EDGE_CURVE ( 'NONE', #18006, #30906, #9447, .T. ) ;
#24799=DIRECTION ( 'NONE',  ( -0.000000000000000000, -1.000000000000000000, -0.000000000000000000 ) ) ;
#24800=AXIS2_PLACEMENT_3D ( 'NONE', #36780, #8147, #8765 ) ;
#24805=ORIENTED_EDGE ( 'NONE', *, *, #24167, .F. ) ;
#24829=VECTOR ( 'NONE', #14442, 1000.000000000000000 ) ;
#24839=CARTESIAN_POINT ( 'NONE',  ( -0.2487487021806331078, -26.64985754041175525, 6.700000000000000178 ) ) ;
#24841=EDGE_CURVE ( 'NONE', #17923, #20627, #11426, .T. ) ;
#24842=LINE ( 'NONE', #24217, #8341 ) ;
#24846=EDGE_LOOP ( 'NONE', ( #38464, #36148, #10035, #8919 ) ) ;
#24850=CARTESIAN_POINT ( 'NONE',  ( -30.87867591359218977, -26.64985754041175525, 6.700000000000000178 ) ) ;
#24851=AXIS2_PLACEMENT_3D ( 'NONE', #33897, #2611, #24401 ) ;
#24858=FACE_OUTER_BOUND ( 'NONE', #22488, .T. ) ;
#24863=CARTESIAN_POINT ( 'NONE',  ( -44.23414840393349579, -30.38627270959228710, 6.000000000000000000 ) ) ;
#24864=LINE ( 'NONE', #37404, #17578 ) ;
#24867=VERTEX_POINT ( 'NONE', #24221 ) ;
#24869=EDGE_CURVE ( 'NONE', #25800, #27373, #11440, .T. ) ;
#24876=ORIENTED_EDGE ( 'NONE', *, *, #8051, .F. ) ;
#24877=VECTOR ( 'NONE', #33443, 1000.000000000000000 ) ;
#24892=ORIENTED_EDGE ( 'NONE', *, *, #23536, .T. ) ;
#24898=ORIENTED_EDGE ( 'NONE', *, *, #22801, .F. ) ;
#24900=ORIENTED_EDGE ( 'NONE', *, *, #1938, .T. ) ;
#24904=AXIS2_PLACEMENT_3D ( 'NONE', #22551, #721, #13671 ) ;
#24909=ORIENTED_EDGE ( 'NONE', *, *, #13724, .T. ) ;
#24920=AXIS2_PLACEMENT_3D ( 'NONE', #12153, #18534, #34225 ) ;
#24924=CARTESIAN_POINT ( 'NONE',  ( 1.651251297819358754, -25.49307895267003587, 6.700000000000000178 ) ) ;
#24938=ORIENTED_EDGE ( 'NONE', *, *, #34007, .T. ) ;
#24940=EDGE_CURVE ( 'NONE', #19582, #29208, #31640, .T. ) ;
#24945=ORIENTED_EDGE ( 'NONE', *, *, #543, .F. ) ;
#24951=CARTESIAN_POINT ( 'NONE',  ( -26.87867591359219333, -26.64985754041175525, 6.700000000000000178 ) ) ;
#24952=CARTESIAN_POINT ( 'NONE',  ( -24.87867591359218977, -24.55319635012989110, 6.700000000000000178 ) ) ;
#24958=CIRCLE ( 'NONE', #30201, 0.1000000000000028644 ) ;
#24963=DIRECTION ( 'NONE',  ( -0.000000000000000000, -0.000000000000000000, 1.000000000000000000 ) ) ;
#24966=FACE_OUTER_BOUND ( 'NONE', #23242, .T. ) ;
#24975=EDGE_CURVE ( 'NONE', #23320, #33375, #40465, .T. ) ;
#24990=DIRECTION ( 'NONE',  ( 0.000000000000000000, 1.000000000000000000, 0.000000000000000000 ) ) ;
#24991=CARTESIAN_POINT ( 'NONE',  ( -17.07867591359219617, -24.55319635012989110, 6.700000000000000178 ) ) ;
#24994=AXIS2_PLACEMENT_3D ( 'NONE', #3642, #9986, #21950 ) ;
#24999=VERTEX_POINT ( 'NONE', #28749 ) ;
#25001=DIRECTION ( 'NONE',  ( 0.000000000000000000, 0.000000000000000000, 1.000000000000000000 ) ) ;
#25004=VERTEX_POINT ( 'NONE', #28541 ) ;
#25006=CARTESIAN_POINT ( 'NONE',  ( -10.87867591359219155, -26.64985754041175525, 6.700000000000000178 ) ) ;
#25007=ORIENTED_EDGE ( 'NONE', *, *, #26001, .F. ) ;
#25017=AXIS2_PLACEMENT_3D ( 'NONE', #40407, #37329, #8296 ) ;
#25025=ORIENTED_EDGE ( 'NONE', *, *, #38813, .T. ) ;
#25026=EDGE_CURVE ( 'NONE', #21932, #31406, #19073, .T. ) ;
#25027=CARTESIAN_POINT ( 'NONE',  ( -8.878675913592189772, -26.64985754041175525, 6.800000000000000711 ) ) ;
#25034=DIRECTION ( 'NONE',  ( 1.000000000000000000, 0.000000000000000000, 0.000000000000000000 ) ) ;
#25038=AXIS2_PLACEMENT_3D ( 'NONE', #26999, #12154, #39547 ) ;
#25044=VERTEX_POINT ( 'NONE', #31036 ) ;
#25051=VECTOR ( 'NONE', #35277, 1000.000000000000000 ) ;
#25053=EDGE_LOOP ( 'NONE', ( #21241, #36432, #34635, #16540 ) ) ;
#25057=FACE_OUTER_BOUND ( 'NONE', #21630, .T. ) ;
#25062=DIRECTION ( 'NONE',  ( 1.000000000000000000, 0.000000000000000000, -0.000000000000000000 ) ) ;
#25065=VECTOR ( 'NONE', #20159, 1000.000000000000000 ) ;
#25067=CARTESIAN_POINT ( 'NONE',  ( -32.44874870218063734, -25.49307895267003587, 6.700000000000000178 ) ) ;
#25072=ORIENTED_EDGE ( 'NONE', *, *, #1739, .T. ) ;
#25077=VECTOR ( 'NONE', #7849, 1000.000000000000000 ) ;
#25098=DIRECTION ( 'NONE',  ( 1.000000000000000000, 0.000000000000000000, 0.000000000000000000 ) ) ;
#25101=LINE ( 'NONE', #22429, #4351 ) ;
#25102=ORIENTED_EDGE ( 'NONE', *, *, #2170, .F. ) ;
#25111=EDGE_LOOP ( 'NONE', ( #28025, #659, #18690, #15946 ) ) ;
#25113=CARTESIAN_POINT ( 'NONE',  ( -12.44874870218064267, -25.49307895267003587, 6.700000000000000178 ) ) ;
#25114=DIRECTION ( 'NONE',  ( 0.000000000000000000, 0.000000000000000000, 1.000000000000000000 ) ) ;
#25116=FACE_OUTER_BOUND ( 'NONE', #29954, .T. ) ;
#25120=VERTEX_POINT ( 'NONE', #14090 ) ;
#25142=ADVANCED_FACE ( 'NONE', ( #19875 ), #756, .F. ) ;
#25148=FACE_BOUND ( 'NONE', #23129, .T. ) ;
#25156=VERTEX_POINT ( 'NONE', #1368 ) ;
#25162=CARTESIAN_POINT ( 'NONE',  ( -6.878675913592188884, -24.55319635012989110, 6.800000000000000711 ) ) ;
#25165=VECTOR ( 'NONE', #7720, 1000.000000000000000 ) ;
#25166=ORIENTED_EDGE ( 'NONE', *, *, #30893, .F. ) ;
#25179=ORIENTED_EDGE ( 'NONE', *, *, #37726, .F. ) ;
#25181=DIRECTION ( 'NONE',  ( 0.000000000000000000, 0.000000000000000000, 1.000000000000000000 ) ) ;
#25186=PLANE ( 'NONE',  #8099 ) ;
#25187=CARTESIAN_POINT ( 'NONE',  ( -22.87867591359218977, -24.55319635012989110, 6.700000000000000178 ) ) ;
#25192=DIRECTION ( 'NONE',  ( 1.000000000000000000, 0.000000000000000000, 0.000000000000000000 ) ) ;
#25198=AXIS2_PLACEMENT_3D ( 'NONE', #1235, #11059, #23240 ) ;
#25200=LINE ( 'NONE', #37732, #37062 ) ;
#25201=CARTESIAN_POINT ( 'NONE',  ( -32.24874870218063450, -26.64985754041175525, 6.800000000000000711 ) ) ;
#25204=EDGE_CURVE ( 'NONE', #25800, #40638, #38199, .T. ) ;
#25208=ORIENTED_EDGE ( 'NONE', *, *, #31297, .T. ) ;
#25222=VERTEX_POINT ( 'NONE', #1763 ) ;
#25233=ORIENTED_EDGE ( 'NONE', *, *, #15704, .T. ) ;
#25241=DIRECTION ( 'NONE',  ( 0.000000000000000000, 0.000000000000000000, 1.000000000000000000 ) ) ;
#25251=EDGE_CURVE ( 'NONE', #39141, #14763, #14494, .T. ) ;
#25252=CIRCLE ( 'NONE', #12080, 0.1000000000000028644 ) ;
#25256=CARTESIAN_POINT ( 'NONE',  ( -11.07867591359219794, -24.55319635012989110, 6.700000000000000178 ) ) ;
#25258=ORIENTED_EDGE ( 'NONE', *, *, #19496, .F. ) ;
#25261=ADVANCED_FACE ( 'NONE', ( #14910 ), #14694, .F. ) ;
#25269=ORIENTED_EDGE ( 'NONE', *, *, #18030, .F. ) ;
#25271=AXIS2_PLACEMENT_3D ( 'NONE', #18716, #28184, #3119 ) ;
#25272=CARTESIAN_POINT ( 'NONE',  ( 7.121324086407810228, -24.55319635012989110, 6.700000000000000178 ) ) ;
#25277=VERTEX_POINT ( 'NONE', #30578 ) ;
#25288=VERTEX_POINT ( 'NONE', #7920 ) ;
#25294=CARTESIAN_POINT ( 'NONE',  ( -28.97867591359219475, -26.64985754041175525, 6.700000000000000178 ) ) ;
#25296=EDGE_LOOP ( 'NONE', ( #26515, #6483, #40128, #8370 ) ) ;
#25307=ORIENTED_EDGE ( 'NONE', *, *, #15714, .T. ) ;
#25314=EDGE_LOOP ( 'NONE', ( #26170, #33830, #13203, #16767 ) ) ;
#25319=VERTEX_POINT ( 'NONE', #5243 ) ;
#25322=CARTESIAN_POINT ( 'NONE',  ( -26.44874870218064089, -26.64985754041175525, 6.700000000000000178 ) ) ;
#25329=VERTEX_POINT ( 'NONE', #5451 ) ;
#25333=CARTESIAN_POINT ( 'NONE',  ( -0.8786759135921904385, -24.55319635012989110, 6.800000000000000711 ) ) ;
#25351=EDGE_LOOP ( 'NONE', ( #24539, #20231, #5341, #26979 ) ) ;
#25358=FACE_BOUND ( 'NONE', #5537, .T. ) ;
#25359=DIRECTION ( 'NONE',  ( 0.000000000000000000, 0.000000000000000000, 1.000000000000000000 ) ) ;
#25362=VECTOR ( 'NONE', #5442, 1000.000000000000000 ) ;
#25369=CARTESIAN_POINT ( 'NONE',  ( 5.651251297819362307, -26.64985754041175525, 6.700000000000000178 ) ) ;
#25375=CARTESIAN_POINT ( 'NONE',  ( -32.87867591359218977, -24.55319635012989110, 6.800000000000000711 ) ) ;
#25377=CARTESIAN_POINT ( 'NONE',  ( -38.87867591359218977, -26.64985754041175525, 6.800000000000000711 ) ) ;
#25380=ADVANCED_FACE ( 'NONE', ( #8106 ), #20674, .F. ) ;
#25382=DIRECTION ( 'NONE',  ( 1.000000000000000000, 0.000000000000000000, -0.000000000000000000 ) ) ;
#25388=PLANE ( 'NONE',  #5876 ) ;
#25393=DIRECTION ( 'NONE',  ( -0.000000000000000000, -0.000000000000000000, 1.000000000000000000 ) ) ;
#25396=DIRECTION ( 'NONE',  ( -0.000000000000000000, -0.000000000000000000, 1.000000000000000000 ) ) ;
#25409=DIRECTION ( 'NONE',  ( 0.000000000000000000, 0.000000000000000000, 1.000000000000000000 ) ) ;
#25414=VERTEX_POINT ( 'NONE', #24588 ) ;
#25417=LINE ( 'NONE', #9965, #5255 ) ;
#25418=CIRCLE ( 'NONE', #18916, 0.1000000000000028644 ) ;
#25426=VERTEX_POINT ( 'NONE', #15731 ) ;
#25429=EDGE_LOOP ( 'NONE', ( #232, #2329, #26745, #24604 ) ) ;
#25443=DIRECTION ( 'NONE',  ( 0.000000000000000000, 1.000000000000000000, 0.000000000000000000 ) ) ;
#25446=AXIS2_PLACEMENT_3D ( 'NONE', #32612, #13859, #16932 ) ;
#25448=AXIS2_PLACEMENT_3D ( 'NONE', #24675, #11891, #22418 ) ;
#25449=VECTOR ( 'NONE', #25396, 1000.000000000000000 ) ;
#25451=DIRECTION ( 'NONE',  ( 0.000000000000000000, 1.000000000000000000, 0.000000000000000000 ) ) ;
#25453=EDGE_CURVE ( 'NONE', #7986, #12843, #17910, .T. ) ;
#25458=ORIENTED_EDGE ( 'NONE', *, *, #28912, .F. ) ;
#25459=DIRECTION ( 'NONE',  ( 0.000000000000000000, 1.000000000000000000, 0.000000000000000000 ) ) ;
#25461=VERTEX_POINT ( 'NONE', #31185 ) ;
#25467=VECTOR ( 'NONE', #24244, 1000.000000000000000 ) ;
#25473=CIRCLE ( 'NONE', #21542, 0.1000000000000028644 ) ;
#25487=CARTESIAN_POINT ( 'NONE',  ( -1.078675913592196167, -26.64985754041175525, 6.800000000000000711 ) ) ;
#25488=EDGE_CURVE ( 'NONE', #20646, #12996, #21516, .T. ) ;
#25489=EDGE_CURVE ( 'NONE', #34205, #19079, #24508, .T. ) ;
#25497=ORIENTED_EDGE ( 'NONE', *, *, #29522, .F. ) ;
#25499=CARTESIAN_POINT ( 'NONE',  ( -24.97867591359219475, -24.55319635012989110, 6.700000000000000178 ) ) ;
#25506=CARTESIAN_POINT ( 'NONE',  ( 1.551251297819356001, -26.64985754041175525, 6.700000000000000178 ) ) ;
#25509=EDGE_LOOP ( 'NONE', ( #1606, #39045, #19964, #19661 ) ) ;
#25514=ORIENTED_EDGE ( 'NONE', *, *, #36865, .T. ) ;
#25515=ORIENTED_EDGE ( 'NONE', *, *, #38522, .T. ) ;
#25517=CARTESIAN_POINT ( 'NONE',  ( -42.83131703149249603, -32.06993018339340296, 6.800000000000000711 ) ) ;
#25519=VECTOR ( 'NONE', #11815, 1000.000000000000000 ) ;
#25521=CYLINDRICAL_SURFACE ( 'NONE', #11116, 0.1000000000000028644 ) ;
#25528=ORIENTED_EDGE ( 'NONE', *, *, #15704, .F. ) ;
#25529=AXIS2_PLACEMENT_3D ( 'NONE', #6141, #9412, #34577 ) ;
#25531=EDGE_CURVE ( 'NONE', #31915, #7027, #22127, .T. ) ;
#25533=LINE ( 'NONE', #5982, #39910 ) ;
#25548=CYLINDRICAL_SURFACE ( 'NONE', #21951, 0.1000000000000028644 ) ;
#25559=FACE_BOUND ( 'NONE', #20415, .T. ) ;
#25565=ORIENTED_EDGE ( 'NONE', *, *, #12175, .F. ) ;
#25566=ORIENTED_EDGE ( 'NONE', *, *, #14671, .T. ) ;
#25574=FACE_OUTER_BOUND ( 'NONE', #36958, .T. ) ;
#25576=CARTESIAN_POINT ( 'NONE',  ( -52.01549048184568846, -30.94667987854474234, 6.800000000000000711 ) ) ;
#25586=DIRECTION ( 'NONE',  ( 0.000000000000000000, 1.000000000000000000, 0.000000000000000000 ) ) ;
#25590=FACE_OUTER_BOUND ( 'NONE', #9535, .T. ) ;
#25595=DIRECTION ( 'NONE',  ( 0.000000000000000000, 0.000000000000000000, 1.000000000000000000 ) ) ;
#25597=CARTESIAN_POINT ( 'NONE',  ( 4.921324086407802056, -24.55319635012989110, 6.800000000000000711 ) ) ;
#25608=EDGE_LOOP ( 'NONE', ( #22336, #26486, #24166, #32383 ) ) ;
#25609=LINE ( 'NONE', #16330, #5041 ) ;
#25613=EDGE_LOOP ( 'NONE', ( #9471, #7444, #397, #24478 ) ) ;
#25619=VERTEX_POINT ( 'NONE', #38150 ) ;
#25620=VECTOR ( 'NONE', #19007, 1000.000000000000000 ) ;
#25629=VERTEX_POINT ( 'NONE', #26422 ) ;
#25631=ORIENTED_EDGE ( 'NONE', *, *, #32328, .F. ) ;
#25632=DIRECTION ( 'NONE',  ( 1.000000000000000000, 0.000000000000000000, 0.000000000000000000 ) ) ;
#25633=AXIS2_PLACEMENT_3D ( 'NONE', #11517, #14415, #11311 ) ;
#25656=CARTESIAN_POINT ( 'NONE',  ( -3.078675913592197944, -26.64985754041175525, 6.700000000000000178 ) ) ;
#25657=CARTESIAN_POINT ( 'NONE',  ( -24.44874870218064089, -25.49307895267003587, 6.700000000000000178 ) ) ;
#25659=CARTESIAN_POINT ( 'NONE',  ( -6.348748702180634140, -26.64985754041175525, 6.700000000000000178 ) ) ;
#25660=ORIENTED_EDGE ( 'NONE', *, *, #37274, .F. ) ;
#25661=ORIENTED_EDGE ( 'NONE', *, *, #12675, .F. ) ;
#25663=CYLINDRICAL_SURFACE ( 'NONE', #33234, 0.1000000000000028644 ) ;
#25669=PLANE ( 'NONE',  #19915 ) ;
#25674=EDGE_LOOP ( 'NONE', ( #5188, #24598, #4603, #17471 ) ) ;
#25676=VECTOR ( 'NONE', #11836, 1000.000000000000000 ) ;
#25691=LINE ( 'NONE', #39029, #2228 ) ;
#25695=ADVANCED_FACE ( 'NONE', ( #4405 ), #22536, .F. ) ;
#25706=AXIS2_PLACEMENT_3D ( 'NONE', #30774, #18802, #22721 ) ;
#25707=FACE_OUTER_BOUND ( 'NONE', #23450, .T. ) ;
#25708=ORIENTED_EDGE ( 'NONE', *, *, #351, .T. ) ;
#25710=ORIENTED_EDGE ( 'NONE', *, *, #35567, .T. ) ;
#25712=ADVANCED_FACE ( 'NONE', ( #16929 ), #23128, .F. ) ;
#25723=CARTESIAN_POINT ( 'NONE',  ( -24.97867591359219475, -26.64985754041175525, 6.700000000000000178 ) ) ;
#25727=ORIENTED_EDGE ( 'NONE', *, *, #20853, .F. ) ;
#25738=EDGE_LOOP ( 'NONE', ( #20692, #1535, #11230, #18212 ) ) ;
#25743=LINE ( 'NONE', #38284, #35219 ) ;
#25744=CARTESIAN_POINT ( 'NONE',  ( 11.65737507970504439, -32.06993018339339585, 6.000000000000000000 ) ) ;
#25765=FACE_BOUND ( 'NONE', #3772, .T. ) ;
#25771=ORIENTED_EDGE ( 'NONE', *, *, #24940, .F. ) ;
#25773=CARTESIAN_POINT ( 'NONE',  ( 3.551251297819357777, -26.64985754041175525, 6.700000000000000178 ) ) ;
#25774=PLANE ( 'NONE',  #39337 ) ;
#25789=VECTOR ( 'NONE', #35487, 1000.000000000000000 ) ;
#25791=LINE ( 'NONE', #7046, #25077 ) ;
#25794=DIRECTION ( 'NONE',  ( 0.000000000000000000, 0.000000000000000000, 1.000000000000000000 ) ) ;
#25800=VERTEX_POINT ( 'NONE', #1922 ) ;
#25803=VERTEX_POINT ( 'NONE', #11345 ) ;
#25811=CARTESIAN_POINT ( 'NONE',  ( -36.24874870218063450, -26.64985754041175525, 6.700000000000000178 ) ) ;
#25814=EDGE_CURVE ( 'NONE', #27970, #22388, #29899, .T. ) ;
#25815=ADVANCED_FACE ( 'NONE', ( #1714 ), #36686, .F. ) ;
#25816=DIRECTION ( 'NONE',  ( 1.000000000000000000, -0.000000000000000000, 0.000000000000000000 ) ) ;
#25818=EDGE_CURVE ( 'NONE', #19388, #13396, #11148, .T. ) ;
#25819=DIRECTION ( 'NONE',  ( 1.000000000000000000, 0.000000000000000000, 0.000000000000000000 ) ) ;
#25820=ORIENTED_EDGE ( 'NONE', *, *, #3448, .F. ) ;
#25831=LINE ( 'NONE', #28302, #17355 ) ;
#25833=VECTOR ( 'NONE', #10009, 1000.000000000000000 ) ;
#25844=DIRECTION ( 'NONE',  ( 1.000000000000000000, -0.000000000000000000, 0.000000000000000000 ) ) ;
#25847=FACE_OUTER_BOUND ( 'NONE', #1609, .T. ) ;
#25860=CARTESIAN_POINT ( 'NONE',  ( -14.87867591359218977, -26.64985754041175525, 6.700000000000000178 ) ) ;
#25863=ADVANCED_FACE ( 'NONE', ( #8466 ), #30310, .F. ) ;
#25868=AXIS2_PLACEMENT_3D ( 'NONE', #32718, #17427, #7583 ) ;
#25870=VERTEX_POINT ( 'NONE', #24952 ) ;
#25877=ORIENTED_EDGE ( 'NONE', *, *, #27060, .T. ) ;
#25889=FACE_OUTER_BOUND ( 'NONE', #18959, .T. ) ;
#25891=VERTEX_POINT ( 'NONE', #37488 ) ;
#25892=AXIS2_PLACEMENT_3D ( 'NONE', #23571, #11391, #33472 ) ;
#25897=ORIENTED_EDGE ( 'NONE', *, *, #21424, .T. ) ;
#25901=DIRECTION ( 'NONE',  ( -0.000000000000000000, -1.000000000000000000, -0.000000000000000000 ) ) ;
#25903=ORIENTED_EDGE ( 'NONE', *, *, #24975, .T. ) ;
#25905=CARTESIAN_POINT ( 'NONE',  ( -4.348748702180639469, -25.49307895267003587, 6.700000000000000178 ) ) ;
#25908=DIRECTION ( 'NONE',  ( 1.000000000000000000, 1.241493069327139093E-16, 0.000000000000000000 ) ) ;
#25909=EDGE_LOOP ( 'NONE', ( #12110, #34136, #34041, #38291 ) ) ;
#25912=AXIS2_PLACEMENT_3D ( 'NONE', #28812, #13159, #6783 ) ;
#25914=ORIENTED_EDGE ( 'NONE', *, *, #20688, .T. ) ;
#25917=FACE_OUTER_BOUND ( 'NONE', #36593, .T. ) ;
#25924=CIRCLE ( 'NONE', #31190, 0.1000000000000028644 ) ;
#25927=DIRECTION ( 'NONE',  ( 1.000000000000000000, 0.000000000000000000, 0.000000000000000000 ) ) ;
#25932=VERTEX_POINT ( 'NONE', #15880 ) ;
#25941=ORIENTED_EDGE ( 'NONE', *, *, #1875, .T. ) ;
#25944=VECTOR ( 'NONE', #529, 1000.000000000000000 ) ;
#25950=EDGE_CURVE ( 'NONE', #25461, #40182, #8716, .T. ) ;
#25951=DIRECTION ( 'NONE',  ( -0.000000000000000000, -0.000000000000000000, 1.000000000000000000 ) ) ;
#25953=ADVANCED_FACE ( 'NONE', ( #24743 ), #12384, .T. ) ;
#25954=VECTOR ( 'NONE', #3342, 1000.000000000000000 ) ;
#25963=ORIENTED_EDGE ( 'NONE', *, *, #9843, .T. ) ;
#25966=ORIENTED_EDGE ( 'NONE', *, *, #17697, .F. ) ;
#25967=FACE_BOUND ( 'NONE', #30506, .T. ) ;
#25969=VERTEX_POINT ( 'NONE', #31541 ) ;
#25973=VECTOR ( 'NONE', #39479, 1000.000000000000000 ) ;
#25979=PLANE ( 'NONE',  #15212 ) ;
#25992=PLANE ( 'NONE',  #4444 ) ;
#25997=DIRECTION ( 'NONE',  ( 0.000000000000000000, 0.000000000000000000, 1.000000000000000000 ) ) ;
#25999=CARTESIAN_POINT ( 'NONE',  ( -42.44874870218064444, -26.64985754041175525, 6.800000000000000711 ) ) ;
#26001=EDGE_CURVE ( 'NONE', #4425, #25619, #30936, .T. ) ;
#26005=AXIS2_PLACEMENT_3D ( 'NONE', #27156, #39709, #24060 ) ;
#26007=EDGE_LOOP ( 'NONE', ( #25515, #23866, #38449, #33537 ) ) ;
#26012=DIRECTION ( 'NONE',  ( 0.000000000000000000, 0.000000000000000000, 1.000000000000000000 ) ) ;
#26013=ORIENTED_EDGE ( 'NONE', *, *, #10457, .F. ) ;
#26030=EDGE_CURVE ( 'NONE', #27970, #37105, #40368, .T. ) ;
#26033=VECTOR ( 'NONE', #24587, 1000.000000000000000 ) ;
#26049=PLANE ( 'NONE',  #31477 ) ;
#26053=CARTESIAN_POINT ( 'NONE',  ( -28.44874870218064444, -26.64985754041175525, 6.700000000000000178 ) ) ;
#26055=CARTESIAN_POINT ( 'NONE',  ( -26.97867591359219475, -24.55319635012989110, 6.700000000000000178 ) ) ;
#26060=ORIENTED_EDGE ( 'NONE', *, *, #907, .T. ) ;
#26064=VECTOR ( 'NONE', #2798, 1000.000000000000000 ) ;
#26072=PLANE ( 'NONE',  #37985 ) ;
#26074=VECTOR ( 'NONE', #19798, 1000.000000000000000 ) ;
#26085=ORIENTED_EDGE ( 'NONE', *, *, #31768, .F. ) ;
#26086=DIRECTION ( 'NONE',  ( 1.000000000000000000, 0.000000000000000000, -0.000000000000000000 ) ) ;
#26090=MANIFOLD_SOLID_BREP ( 'Fillet14', #26858 ) ;
#26102=AXIS2_PLACEMENT_3D ( 'NONE', #986, #28777, #16997 ) ;
#26103=ORIENTED_EDGE ( 'NONE', *, *, #16813, .T. ) ;
#26104=EDGE_CURVE ( 'NONE', #33055, #27373, #8094, .T. ) ;
#26108=DIRECTION ( 'NONE',  ( 0.000000000000000000, 0.000000000000000000, 1.000000000000000000 ) ) ;
#26109=ORIENTED_EDGE ( 'NONE', *, *, #21958, .F. ) ;
#26118=PLANE ( 'NONE',  #18790 ) ;
#26120=LINE ( 'NONE', #406, #33398 ) ;
#26122=ORIENTED_EDGE ( 'NONE', *, *, #964, .T. ) ;
#26125=AXIS2_PLACEMENT_3D ( 'NONE', #12611, #7245, #37924 ) ;
#26128=ORIENTED_EDGE ( 'NONE', *, *, #34109, .T. ) ;
#26136=VERTEX_POINT ( 'NONE', #16282 ) ;
#26138=EDGE_LOOP ( 'NONE', ( #28368, #9035, #35698, #39323 ) ) ;
#26139=EDGE_CURVE ( 'NONE', #27725, #29312, #17285, .T. ) ;
#26142=CARTESIAN_POINT ( 'NONE',  ( -12.24874870218063627, -25.49307895267003587, 6.700000000000000178 ) ) ;
#26146=VERTEX_POINT ( 'NONE', #35252 ) ;
#26149=VECTOR ( 'NONE', #20538, 1000.000000000000000 ) ;
#26154=FACE_OUTER_BOUND ( 'NONE', #11699, .T. ) ;
#26162=VERTEX_POINT ( 'NONE', #32760 ) ;
#26163=ORIENTED_EDGE ( 'NONE', *, *, #22966, .T. ) ;
#26168=ORIENTED_EDGE ( 'NONE', *, *, #39201, .F. ) ;
#26170=ORIENTED_EDGE ( 'NONE', *, *, #26282, .T. ) ;
#26177=VECTOR ( 'NONE', #6938, 1000.000000000000000 ) ;
#26178=DIRECTION ( 'NONE',  ( -0.000000000000000000, -0.000000000000000000, 1.000000000000000000 ) ) ;
#26183=DIRECTION ( 'NONE',  ( 1.000000000000000000, -0.000000000000000000, 0.000000000000000000 ) ) ;
#26187=ORIENTED_EDGE ( 'NONE', *, *, #854, .T. ) ;
#26189=EDGE_CURVE ( 'NONE', #34939, #9457, #38907, .T. ) ;
#26192=DIRECTION ( 'NONE',  ( -0.000000000000000000, -1.000000000000000000, -0.000000000000000000 ) ) ;
#26205=CARTESIAN_POINT ( 'NONE',  ( 3.751251297819363728, -26.64985754041175525, 6.700000000000000178 ) ) ;
#26211=CARTESIAN_POINT ( 'NONE',  ( -16.34874870218063592, -26.64985754041175525, 6.700000000000000178 ) ) ;
#26218=CARTESIAN_POINT ( 'NONE',  ( 11.65737507970504616, -30.94667987854474234, 6.000000000000000000 ) ) ;
#26227=DIRECTION ( 'NONE',  ( 0.000000000000000000, 0.000000000000000000, 1.000000000000000000 ) ) ;
#26231=CYLINDRICAL_SURFACE ( 'NONE', #16030, 7.341749246864647915 ) ;
#26235=ADVANCED_FACE ( 'NONE', ( #35808 ), #30219, .F. ) ;
#26248=LINE ( 'NONE', #12861, #8125 ) ;
#26249=VECTOR ( 'NONE', #25443, 1000.000000000000000 ) ;
#26250=CARTESIAN_POINT ( 'NONE',  ( 5.551251297819359110, -26.64985754041175525, 6.700000000000000178 ) ) ;
#26257=PRODUCT ( 'Measuring Ruler', 'Measuring Ruler', '', ( #17991 ) ) ;
#26261=CIRCLE ( 'NONE', #1963, 6.781342077912186461 ) ;
#26269=ADVANCED_FACE ( 'NONE', ( #27125 ), #20138, .F. ) ;
#26272=CIRCLE ( 'NONE', #33509, 0.1000000000000028644 ) ;
#26273=VERTEX_POINT ( 'NONE', #7783 ) ;
#26276=EDGE_CURVE ( 'NONE', #9457, #26319, #19284, .T. ) ;
#26282=EDGE_CURVE ( 'NONE', #14626, #1980, #21908, .T. ) ;
#26301=VECTOR ( 'NONE', #37466, 1000.000000000000000 ) ;
#26306=CARTESIAN_POINT ( 'NONE',  ( -10.34874870218063769, -26.64985754041175525, 6.800000000000000711 ) ) ;
#26315=EDGE_LOOP ( 'NONE', ( #22384, #11441, #17664, #5195 ) ) ;
#26318=CARTESIAN_POINT ( 'NONE',  ( -8.248748702180632719, -26.64985754041175525, 6.700000000000000178 ) ) ;
#26319=VERTEX_POINT ( 'NONE', #33325 ) ;
#26321=ORIENTED_EDGE ( 'NONE', *, *, #7658, .F. ) ;
#26323=LINE ( 'NONE', #29410, #19418 ) ;
#26330=EDGE_CURVE ( 'NONE', #36632, #7986, #36599, .T. ) ;
#26343=CIRCLE ( 'NONE', #30295, 0.1000000000000028644 ) ;
#26349=VERTEX_POINT ( 'NONE', #5105 ) ;
#26356=DIRECTION ( 'NONE',  ( -0.000000000000000000, -0.000000000000000000, 1.000000000000000000 ) ) ;
#26359=CIRCLE ( 'NONE', #32304, 0.1000000000000028644 ) ;
#26362=ORIENTED_EDGE ( 'NONE', *, *, #11834, .T. ) ;
#26371=FACE_OUTER_BOUND ( 'NONE', #25296, .T. ) ;
#26388=CARTESIAN_POINT ( 'NONE',  ( -18.24874870218063450, -26.64985754041175525, 6.800000000000000711 ) ) ;
#26392=CARTESIAN_POINT ( 'NONE',  ( -25.07867591359219617, -26.64985754041175525, 6.800000000000000711 ) ) ;
#26393=CARTESIAN_POINT ( 'NONE',  ( -20.97867591359219475, -24.55319635012989110, 6.700000000000000178 ) ) ;
#26398=DIRECTION ( 'NONE',  ( 0.000000000000000000, 1.000000000000000000, 0.000000000000000000 ) ) ;
#26399=CARTESIAN_POINT ( 'NONE',  ( -32.97867591359219119, -24.55319635012989110, 6.700000000000000178 ) ) ;
#26404=DIRECTION ( 'NONE',  ( 0.000000000000000000, 0.000000000000000000, 1.000000000000000000 ) ) ;
#26406=CARTESIAN_POINT ( 'NONE',  ( -12.87867591359218977, -26.64985754041175525, 6.700000000000000178 ) ) ;
#26415=EDGE_CURVE ( 'NONE', #10273, #35786, #14156, .T. ) ;
#26417=LINE ( 'NONE', #35691, #22633 ) ;
#26422=CARTESIAN_POINT ( 'NONE',  ( -25.07867591359219617, -24.55319635012989110, 6.800000000000000711 ) ) ;
#26423=VERTEX_POINT ( 'NONE', #316 ) ;
#26427=AXIS2_PLACEMENT_3D ( 'NONE', #25723, #13352, #25927 ) ;
#26430=ORIENTED_EDGE ( 'NONE', *, *, #26139, .F. ) ;
#26437=LINE ( 'NONE', #22749, #7627 ) ;
#26439=CARTESIAN_POINT ( 'NONE',  ( -0.8786759135921904385, -26.64985754041175525, 6.800000000000000711 ) ) ;
#26442=ORIENTED_EDGE ( 'NONE', *, *, #40512, .F. ) ;
#26447=DIRECTION ( 'NONE',  ( -0.000000000000000000, -0.000000000000000000, 1.000000000000000000 ) ) ;
#26451=CARTESIAN_POINT ( 'NONE',  ( -14.34874870218063769, -25.49307895267003587, 6.800000000000000711 ) ) ;
#26458=EDGE_CURVE ( 'NONE', #3311, #30682, #21930, .T. ) ;
#26466=CARTESIAN_POINT ( 'NONE',  ( -24.24874870218063450, -26.64985754041175525, 6.700000000000000178 ) ) ;
#26467=FACE_OUTER_BOUND ( 'NONE', #12688, .T. ) ;
#26469=CARTESIAN_POINT ( 'NONE',  ( 1.751251297819361730, -25.49307895267003587, 6.800000000000000711 ) ) ;
#26470=ORIENTED_EDGE ( 'NONE', *, *, #11187, .F. ) ;
#26477=VERTEX_POINT ( 'NONE', #11184 ) ;
#26480=DIRECTION ( 'NONE',  ( -0.000000000000000000, -1.000000000000000000, -0.000000000000000000 ) ) ;
#26483=ORIENTED_EDGE ( 'NONE', *, *, #30765, .T. ) ;
#26485=VECTOR ( 'NONE', #2795, 1000.000000000000000 ) ;
#26486=ORIENTED_EDGE ( 'NONE', *, *, #29343, .T. ) ;
#26487=EDGE_CURVE ( 'NONE', #17020, #34298, #23757, .T. ) ;
#26499=EDGE_CURVE ( 'NONE', #26146, #23756, #28484, .T. ) ;
#26504=ADVANCED_FACE ( 'NONE', ( #27863 ), #6056, .T. ) ;
#26505=ORIENTED_EDGE ( 'NONE', *, *, #16777, .T. ) ;
#26506=CARTESIAN_POINT ( 'NONE',  ( -35.07867591359219972, -24.55319635012989110, 6.700000000000000178 ) ) ;
#26515=ORIENTED_EDGE ( 'NONE', *, *, #20958, .T. ) ;
#26516=LINE ( 'NONE', #26908, #22202 ) ;
#26525=LINE ( 'NONE', #17235, #20318 ) ;
#26531=VECTOR ( 'NONE', #21365, 1000.000000000000000 ) ;
#26536=CARTESIAN_POINT ( 'NONE',  ( -42.83131703149249603, -29.56993018339339940, 6.000000000000000000 ) ) ;
#26543=CARTESIAN_POINT ( 'NONE',  ( -38.24874870218063450, -26.64985754041175525, 6.700000000000000178 ) ) ;
#26548=CARTESIAN_POINT ( 'NONE',  ( -34.24874870218063450, -26.64985754041175525, 6.700000000000000178 ) ) ;
#26550=CARTESIAN_POINT ( 'NONE',  ( -51.01549048184568846, -30.38627270959228710, 6.000000000000000000 ) ) ;
#26557=VERTEX_POINT ( 'NONE', #30566 ) ;
#26565=LINE ( 'NONE', #36233, #37803 ) ;
#26576=CARTESIAN_POINT ( 'NONE',  ( -38.34874870218063592, -26.64985754041175525, 6.700000000000000178 ) ) ;
#26579=DIRECTION ( 'NONE',  ( 1.000000000000000000, 0.000000000000000000, 0.000000000000000000 ) ) ;
#26584=FACE_OUTER_BOUND ( 'NONE', #3309, .T. ) ;
#26593=VERTEX_POINT ( 'NONE', #9536 ) ;
#26594=CARTESIAN_POINT ( 'NONE',  ( -12.87867591359218977, -26.64985754041175525, 6.800000000000000711 ) ) ;
#26601=CYLINDRICAL_SURFACE ( 'NONE', #17774, 0.1000000000000028644 ) ;
#26609=CIRCLE ( 'NONE', #34544, 0.1000000000000028644 ) ;
#26610=VERTEX_POINT ( 'NONE', #18393 ) ;
#26616=CARTESIAN_POINT ( 'NONE',  ( -42.24874870218063450, -26.64985754041175525, 6.700000000000000178 ) ) ;
#26632=EDGE_LOOP ( 'NONE', ( #39310, #9461, #31230, #25566 ) ) ;
#26635=CARTESIAN_POINT ( 'NONE',  ( -12.24874870218063627, -25.49307895267003587, 6.800000000000000711 ) ) ;
#26636=ORIENTED_EDGE ( 'NONE', *, *, #30031, .F. ) ;
#26643=EDGE_CURVE ( 'NONE', #5611, #34412, #9132, .T. ) ;
#26654=AXIS2_PLACEMENT_3D ( 'NONE', #26864, #11197, #27073 ) ;
#26661=ORIENTED_EDGE ( 'NONE', *, *, #24167, .T. ) ;
#26664=CARTESIAN_POINT ( 'NONE',  ( -2.348748702180637693, -26.64985754041175525, 6.800000000000000711 ) ) ;
#26669=VECTOR ( 'NONE', #18900, 1000.000000000000000 ) ;
#26670=AXIS2_PLACEMENT_3D ( 'NONE', #34033, #30309, #34239 ) ;
#26679=FACE_OUTER_BOUND ( 'NONE', #19090, .T. ) ;
#26693=CARTESIAN_POINT ( 'NONE',  ( -32.34874870218063592, -26.64985754041175525, 6.800000000000000711 ) ) ;
#26694=CARTESIAN_POINT ( 'NONE',  ( -2.978675913592195190, -26.64985754041175525, 6.700000000000000178 ) ) ;
#26695=LINE ( 'NONE', #10824, #35244 ) ;
#26701=EDGE_CURVE ( 'NONE', #28895, #6408, #29297, .T. ) ;
#26702=DIRECTION ( 'NONE',  ( 1.000000000000000000, 0.000000000000000000, 0.000000000000000000 ) ) ;
#26715=ORIENTED_EDGE ( 'NONE', *, *, #2692, .F. ) ;
#26724=EDGE_CURVE ( 'NONE', #19656, #6556, #28482, .T. ) ;
#26726=DIRECTION ( 'NONE',  ( -1.000000000000000000, 0.000000000000000000, -2.891205793294675861E-16 ) ) ;
#26727=DIRECTION ( 'NONE',  ( 1.000000000000000000, 0.000000000000000000, 0.000000000000000000 ) ) ;
#26728=DIRECTION ( 'NONE',  ( 0.000000000000000000, 0.000000000000000000, 1.000000000000000000 ) ) ;
#26730=CARTESIAN_POINT ( 'NONE',  ( -23.07867591359219617, -26.64985754041175525, 6.700000000000000178 ) ) ;
#26735=ADVANCED_FACE ( 'NONE', ( #13236 ), #35092, .F. ) ;
#26738=LINE ( 'NONE', #17648, #25467 ) ;
#26743=EDGE_LOOP ( 'NONE', ( #801, #39985, #28182, #33162 ) ) ;
#26745=ORIENTED_EDGE ( 'NONE', *, *, #32427, .F. ) ;
#26749=DIRECTION ( 'NONE',  ( 0.000000000000000000, 0.000000000000000000, 1.000000000000000000 ) ) ;
#26754=FACE_OUTER_BOUND ( 'NONE', #40537, .T. ) ;
#26758=VERTEX_POINT ( 'NONE', #4000 ) ;
#26765=AXIS2_PLACEMENT_3D ( 'NONE', #36556, #26885, #5265 ) ;
#26767=EDGE_LOOP ( 'NONE', ( #4100, #30148, #7057, #19553 ) ) ;
#26788=FACE_OUTER_BOUND ( 'NONE', #27483, .T. ) ;
#26790=CARTESIAN_POINT ( 'NONE',  ( -8.348748702180635917, -26.64985754041175525, 6.700000000000000178 ) ) ;
#26797=ORIENTED_EDGE ( 'NONE', *, *, #5966, .T. ) ;
#26801=CARTESIAN_POINT ( 'NONE',  ( -51.21549048184568420, -30.38627270959228710, 4.000000000000000000 ) ) ;
#26803=CARTESIAN_POINT ( 'NONE',  ( -24.34874870218063592, -25.49307895267003587, 6.700000000000000178 ) ) ;
#26804=DIRECTION ( 'NONE',  ( -0.000000000000000000, -0.000000000000000000, 1.000000000000000000 ) ) ;
#26805=VERTEX_POINT ( 'NONE', #25597 ) ;
#26818=CARTESIAN_POINT ( 'NONE',  ( -28.34874870218063947, -25.49307895267003587, 6.700000000000000178 ) ) ;
#26830=EDGE_CURVE ( 'NONE', #32857, #10365, #28893, .T. ) ;
#26834=CARTESIAN_POINT ( 'NONE',  ( -20.97867591359219475, -26.64985754041175525, 6.700000000000000178 ) ) ;
#26842=ORIENTED_EDGE ( 'NONE', *, *, #36402, .T. ) ;
#26845=FACE_OUTER_BOUND ( 'NONE', #30700, .T. ) ;
#26848=DIRECTION ( 'NONE',  ( -1.000000000000000000, 0.000000000000000000, 0.000000000000000000 ) ) ;
#26850=AXIS2_PLACEMENT_3D ( 'NONE', #40442, #24612, #36966 ) ;
#26853=VERTEX_POINT ( 'NONE', #36471 ) ;
#26856=ORIENTED_EDGE ( 'NONE', *, *, #27061, .F. ) ;
#26858=CLOSED_SHELL ( 'NONE', ( #9063, #18448, #16738, #32611, #17858, #18261, #1701, #6589, #641, #14151, #39791, #9047, #17003, #9528, #18314, #13679, #32447, #27103, #1625, #554, #8285, #34618, #23607, #40383, #39025, #19494, #30255, #23029, #29164, #14120, #25953, #30500, #19310, #779, #35032, #4102, #38722, #18028, #13118, #6203, #10543, #29978, #21759, #857, #34434, #22242, #17504, #38096, #3362, #18965, #39005, #16802, #25261, #9956, #2762, #2399, #10182, #19266, #15867, #38388, #10314, #17695, #6675, #11299, #342, #12648, #13137, #34906, #40160, #35292, #172, #9629, #34075, #25712, #39481, #17795, #12615, #2634, #4031, #5922, #31253, #5223, #682, #23012, #12536, #33492, #7313, #25863, #34259, #17873, #27711, #30844, #17874, #14840, #39312, #24728, #29745, #9254, #18715, #29520, #21379, #16365, #1891, #34764, #8554, #30088, #9960, #5911, #23620, #5454, #40326, #32690, #7620, #4620, #5280, #10087, #23018, #21674, #40340, #21123, #23427, #25142, #36020, #34952, #29823, #1646, #21473, #32953, #13856, #15017, #2927, #23875, #37822, #2066, #13434, #37147, #12114, #2914, #25815, #33767, #37258, #33634, #26735, #33995, #36823, #36573, #30244, #7802, #23080, #32339, #9431, #10349, #25380, #28371, #11537, #38439, #35076, #38017, #16502, #25695, #32840, #5300, #29695, #26269, #8798, #30206, #39936, #26235, #33588, #2981, #33967, #5819, #29012, #19970, #39591, #7806, #34387, #33796, #38262, #19396, #37545, #6789, #33538, #27794, #23577, #31631, #1066, #33638, #6391, #5566, #15179, #39026, #14313, #1546, #17547, #10283, #7441, #37676, #24019, #22885, #31353, #4882, #11408, #7515, #34244, #20395, #30155, #19942, #20348, #39602, #39645, #20711, #27513, #18366, #20488, #33920, #36440, #7863, #26896, #17879, #24260, #24448, #8996, #9909, #19104, #26504, #14497, #1000, #23922, #5028, #20426, #9814, #16150, #33355, #32268, #17580, #15902, #13539, #38002, #17186, #6571, #28840, #20608, #18164, #29056, #14087, #29618, #14537, #9676, #7856, #13439, #9377, #33106, #36585, #32829, #35503, #27275, #12927, #2311, #17397, #14272, #1776, #40566, #39066, #4932, #12881, #31470 ) ) ;
#26863=DIRECTION ( 'NONE',  ( -1.000000000000000000, 0.000000000000000000, 0.000000000000000000 ) ) ;
#26864=CARTESIAN_POINT ( 'NONE',  ( -20.34874870218063947, -26.64985754041175525, 6.700000000000000178 ) ) ;
#26870=EDGE_LOOP ( 'NONE', ( #11646, #40164, #38652, #22670 ) ) ;
#26871=VECTOR ( 'NONE', #6516, 1000.000000000000000 ) ;
#26875=CARTESIAN_POINT ( 'NONE',  ( -28.87867591359218977, -26.64985754041175525, 6.700000000000000178 ) ) ;
#26878=ORIENTED_EDGE ( 'NONE', *, *, #33802, .F. ) ;
#26884=DIRECTION ( 'NONE',  ( 0.000000000000000000, 0.000000000000000000, 1.000000000000000000 ) ) ;
#26885=DIRECTION ( 'NONE',  ( 0.000000000000000000, 0.000000000000000000, 1.000000000000000000 ) ) ;
#26888=DIRECTION ( 'NONE',  ( 0.000000000000000000, 0.000000000000000000, -1.000000000000000000 ) ) ;
#26893=DIRECTION ( 'NONE',  ( 1.000000000000000000, 0.000000000000000000, 0.000000000000000000 ) ) ;
#26896=ADVANCED_FACE ( 'NONE', ( #20214 ), #7862, .F. ) ;
#26897=AXIS2_PLACEMENT_3D ( 'NONE', #4623, #8495, #11172 ) ;
#26905=VERTEX_POINT ( 'NONE', #20817 ) ;
#26908=CARTESIAN_POINT ( 'NONE',  ( -19.07867591359219972, -26.64985754041175525, 6.800000000000000711 ) ) ;
#26922=CARTESIAN_POINT ( 'NONE',  ( -3.078675913592197944, -26.64985754041175525, 6.700000000000000178 ) ) ;
#26924=DIRECTION ( 'NONE',  ( 0.000000000000000000, 0.000000000000000000, 1.000000000000000000 ) ) ;
#26927=ORIENTED_EDGE ( 'NONE', *, *, #12630, .T. ) ;
#26931=DIRECTION ( 'NONE',  ( -0.000000000000000000, -1.000000000000000000, -0.000000000000000000 ) ) ;
#26945=DIRECTION ( 'NONE',  ( 1.000000000000000000, 0.000000000000000000, 0.000000000000000000 ) ) ;
#26949=ORIENTED_EDGE ( 'NONE', *, *, #4214, .T. ) ;
#26950=EDGE_LOOP ( 'NONE', ( #6693, #7062, #11855, #34512 ) ) ;
#26957=ORIENTED_EDGE ( 'NONE', *, *, #5581, .F. ) ;
#26959=CARTESIAN_POINT ( 'NONE',  ( -8.448748702180639114, -25.49307895267003587, 6.700000000000000178 ) ) ;
#26963=CYLINDRICAL_SURFACE ( 'NONE', #27464, 0.1000000000000028644 ) ;
#26975=CARTESIAN_POINT ( 'NONE',  ( -34.34874870218063592, -26.64985754041175525, 6.700000000000000178 ) ) ;
#26979=ORIENTED_EDGE ( 'NONE', *, *, #29665, .T. ) ;
#26981=PLANE ( 'NONE',  #18828 ) ;
#26983=DIRECTION ( 'NONE',  ( 0.000000000000000000, 0.000000000000000000, -1.000000000000000000 ) ) ;
#26999=CARTESIAN_POINT ( 'NONE',  ( -22.34874870218063947, -26.64985754041175525, 6.800000000000000711 ) ) ;
#27001=AXIS2_PLACEMENT_3D ( 'NONE', #36323, #20256, #35929 ) ;
#27032=VECTOR ( 'NONE', #9425, 1000.000000000000000 ) ;
#27035=CYLINDRICAL_SURFACE ( 'NONE', #17608, 0.1000000000000028644 ) ;
#27040=ORIENTED_EDGE ( 'NONE', *, *, #11139, .T. ) ;
#27060=EDGE_CURVE ( 'NONE', #12640, #32941, #8863, .T. ) ;
#27061=EDGE_CURVE ( 'NONE', #26423, #31406, #35672, .T. ) ;
#27064=AXIS2_PLACEMENT_3D ( 'NONE', #24093, #30092, #11727 ) ;
#27065=EDGE_CURVE ( 'NONE', #38045, #17923, #5795, .T. ) ;
#27066=CARTESIAN_POINT ( 'NONE',  ( 6.921324086407803833, -24.55319635012989110, 6.700000000000000178 ) ) ;
#27072=ORIENTED_EDGE ( 'NONE', *, *, #38845, .T. ) ;
#27073=DIRECTION ( 'NONE',  ( 1.000000000000000000, 0.000000000000000000, 0.000000000000000000 ) ) ;
#27092=CARTESIAN_POINT ( 'NONE',  ( -28.34874870218063947, -25.49307895267003587, 6.700000000000000178 ) ) ;
#27096=CARTESIAN_POINT ( 'NONE',  ( -34.97867591359219830, -24.55319635012989110, 6.700000000000000178 ) ) ;
#27097=ORIENTED_EDGE ( 'NONE', *, *, #1751, .F. ) ;
#27101=FACE_OUTER_BOUND ( 'NONE', #1915, .T. ) ;
#27103=ADVANCED_FACE ( 'NONE', ( #6002 ), #18539, .F. ) ;
#27106=PLANE ( 'NONE',  #33361 ) ;
#27113=CARTESIAN_POINT ( 'NONE',  ( 3.751251297819363728, -25.49307895267003587, 6.700000000000000178 ) ) ;
#27118=ORIENTED_EDGE ( 'NONE', *, *, #5073, .T. ) ;
#27119=CARTESIAN_POINT ( 'NONE',  ( -38.97867591359219119, -26.64985754041175525, 6.700000000000000178 ) ) ;
#27123=FACE_OUTER_BOUND ( 'NONE', #13880, .T. ) ;
#27125=FACE_OUTER_BOUND ( 'NONE', #16202, .T. ) ;
#27126=EDGE_CURVE ( 'NONE', #30074, #2141, #18533, .T. ) ;
#27129=FACE_OUTER_BOUND ( 'NONE', #34231, .T. ) ;
#27132=DIRECTION ( 'NONE',  ( -1.000000000000000000, -1.241493069327139093E-16, 0.000000000000000000 ) ) ;
#27141=DIRECTION ( 'NONE',  ( 0.000000000000000000, 1.000000000000000000, 0.000000000000000000 ) ) ;
#27144=ORIENTED_EDGE ( 'NONE', *, *, #5773, .F. ) ;
#27146=AXIS2_PLACEMENT_3D ( 'NONE', #37292, #34650, #11956 ) ;
#27149=ORIENTED_EDGE ( 'NONE', *, *, #8779, .T. ) ;
#27154=CARTESIAN_POINT ( 'NONE',  ( -0.3487487021806359722, -25.49307895267003587, 6.700000000000000178 ) ) ;
#27156=CARTESIAN_POINT ( 'NONE',  ( -4.348748702180639469, -25.49307895267003587, 6.800000000000000711 ) ) ;
#27158=ORIENTED_EDGE ( 'NONE', *, *, #29433, .F. ) ;
#27177=CYLINDRICAL_SURFACE ( 'NONE', #745, 0.1000000000000028644 ) ;
#27184=PLANE ( 'NONE',  #8965 ) ;
#27185=EDGE_CURVE ( 'NONE', #11338, #31323, #34362, .T. ) ;
#27186=EDGE_CURVE ( 'NONE', #7892, #17923, #6617, .T. ) ;
#27191=AXIS2_PLACEMENT_3D ( 'NONE', #13250, #18818, #31391 ) ;
#27194=CYLINDRICAL_SURFACE ( 'NONE', #29890, 2.000000000000000000 ) ;
#27196=DIRECTION ( 'NONE',  ( 0.000000000000000000, 0.000000000000000000, 1.000000000000000000 ) ) ;
#27199=CYLINDRICAL_SURFACE ( 'NONE', #34256, 0.1000000000000028644 ) ;
#27210=LINE ( 'NONE', #24324, #24829 ) ;
#27211=DIRECTION ( 'NONE',  ( 0.000000000000000000, 1.000000000000000000, 0.000000000000000000 ) ) ;
#27219=ORIENTED_EDGE ( 'NONE', *, *, #31064, .T. ) ;
#27231=ORIENTED_EDGE ( 'NONE', *, *, #15249, .F. ) ;
#27233=CARTESIAN_POINT ( 'NONE',  ( -30.97867591359219119, -26.64985754041175525, 6.700000000000000178 ) ) ;
#27239=DIRECTION ( 'NONE',  ( -0.000000000000000000, -1.000000000000000000, -0.000000000000000000 ) ) ;
#27250=CARTESIAN_POINT ( 'NONE',  ( -10.87867591359219155, -26.64985754041175525, 6.700000000000000178 ) ) ;
#27251=AXIS2_PLACEMENT_3D ( 'NONE', #6698, #37756, #22354 ) ;
#27255=VECTOR ( 'NONE', #19570, 1000.000000000000000 ) ;
#27256=ORIENTED_EDGE ( 'NONE', *, *, #16275, .F. ) ;
#27257=CARTESIAN_POINT ( 'NONE',  ( -40.24874870218063450, -26.64985754041175525, 6.800000000000000711 ) ) ;
#27264=CARTESIAN_POINT ( 'NONE',  ( -52.01549048184568846, -38.28842912540938670, 4.800000000000000711 ) ) ;
#27272=AXIS2_PLACEMENT_3D ( 'NONE', #3193, #12816, #12207 ) ;
#27273=VECTOR ( 'NONE', #31265, 1000.000000000000000 ) ;
#27274=CARTESIAN_POINT ( 'NONE',  ( -30.34874870218063947, -25.49307895267003587, 6.700000000000000178 ) ) ;
#27275=ADVANCED_FACE ( 'NONE', ( #3749 ), #22274, .F. ) ;
#27292=PLANE ( 'NONE',  #30236 ) ;
#27299=ORIENTED_EDGE ( 'NONE', *, *, #12683, .F. ) ;
#27300=VECTOR ( 'NONE', #27141, 1000.000000000000000 ) ;
#27310=VERTEX_POINT ( 'NONE', #30249 ) ;
#27319=ORIENTED_EDGE ( 'NONE', *, *, #11270, .T. ) ;
#27324=DIRECTION ( 'NONE',  ( -1.000000000000000000, 0.000000000000000000, 0.000000000000000000 ) ) ;
#27329=DIRECTION ( 'NONE',  ( 1.000000000000000000, 0.000000000000000000, -0.000000000000000000 ) ) ;
#27330=EDGE_CURVE ( 'NONE', #1874, #30074, #4543, .T. ) ;
#27331=VECTOR ( 'NONE', #13133, 1000.000000000000000 ) ;
#27340=ORIENTED_EDGE ( 'NONE', *, *, #6152, .F. ) ;
#27342=VECTOR ( 'NONE', #6029, 1000.000000000000000 ) ;
#27347=CARTESIAN_POINT ( 'NONE',  ( -4.448748702180642667, -25.49307895267003587, 6.700000000000000178 ) ) ;
#27353=ORIENTED_EDGE ( 'NONE', *, *, #14302, .T. ) ;
#27359=CARTESIAN_POINT ( 'NONE',  ( -45.33131703149249603, -29.56993018339339940, 6.800000000000000711 ) ) ;
#27361=FACE_OUTER_BOUND ( 'NONE', #36299, .T. ) ;
#27362=ORIENTED_EDGE ( 'NONE', *, *, #14827, .F. ) ;
#27370=VECTOR ( 'NONE', #6840, 1000.000000000000000 ) ;
#27372=CARTESIAN_POINT ( 'NONE',  ( -19.07867591359219972, -24.55319635012989110, 6.700000000000000178 ) ) ;
#27373=VERTEX_POINT ( 'NONE', #5134 ) ;
#27382=CARTESIAN_POINT ( 'NONE',  ( -16.24874870218063450, -26.64985754041175525, 6.800000000000000711 ) ) ;
#27397=DIRECTION ( 'NONE',  ( 0.000000000000000000, 0.000000000000000000, 1.000000000000000000 ) ) ;
#27414=CARTESIAN_POINT ( 'NONE',  ( -30.44874870218064089, -25.49307895267003587, 6.700000000000000178 ) ) ;
#27416=ORIENTED_EDGE ( 'NONE', *, *, #24551, .T. ) ;
#27435=AXIS2_PLACEMENT_3D ( 'NONE', #22779, #7513, #16567 ) ;
#27447=DIRECTION ( 'NONE',  ( -0.000000000000000000, -0.000000000000000000, 1.000000000000000000 ) ) ;
#27459=AXIS2_PLACEMENT_3D ( 'NONE', #17852, #21171, #27542 ) ;
#27460=CARTESIAN_POINT ( 'NONE',  ( 7.021324086407807030, -24.55319635012989110, 6.700000000000000178 ) ) ;
#27463=CARTESIAN_POINT ( 'NONE',  ( -36.34874870218064302, -26.64985754041175525, 6.700000000000000178 ) ) ;
#27464=AXIS2_PLACEMENT_3D ( 'NONE', #36042, #39926, #30058 ) ;
#27469=LINE ( 'NONE', #27066, #12047 ) ;
#27477=ORIENTED_EDGE ( 'NONE', *, *, #15336, .F. ) ;
#27483=EDGE_LOOP ( 'NONE', ( #930, #1056, #36044, #36988 ) ) ;
#27490=VECTOR ( 'NONE', #36156, 1000.000000000000000 ) ;
#27501=DIRECTION ( 'NONE',  ( -0.000000000000000000, -0.000000000000000000, 1.000000000000000000 ) ) ;
#27502=DIRECTION ( 'NONE',  ( -0.000000000000000000, -1.000000000000000000, -0.000000000000000000 ) ) ;
#27506=PLANE ( 'NONE',  #6611 ) ;
#27507=DIRECTION ( 'NONE',  ( 0.000000000000000000, 1.000000000000000000, 0.000000000000000000 ) ) ;
#27513=ADVANCED_FACE ( 'NONE', ( #2769 ), #40607, .F. ) ;
#27514=DIRECTION ( 'NONE',  ( 1.000000000000000000, 0.000000000000000000, 0.000000000000000000 ) ) ;
#27516=EDGE_CURVE ( 'NONE', #36422, #21009, #18857, .T. ) ;
#27526=ORIENTED_EDGE ( 'NONE', *, *, #9592, .T. ) ;
#27531=ORIENTED_EDGE ( 'NONE', *, *, #7153, .F. ) ;
#27533=CIRCLE ( 'NONE', #9790, 0.1000000000000028644 ) ;
#27534=FACE_OUTER_BOUND ( 'NONE', #848, .T. ) ;
#27535=CARTESIAN_POINT ( 'NONE',  ( -18.97867591359219475, -26.64985754041175525, 6.700000000000000178 ) ) ;
#27542=DIRECTION ( 'NONE',  ( 1.000000000000000000, 0.000000000000000000, 0.000000000000000000 ) ) ;
#27546=ORIENTED_EDGE ( 'NONE', *, *, #23077, .T. ) ;
#27547=FACE_OUTER_BOUND ( 'NONE', #12261, .T. ) ;
#27549=CARTESIAN_POINT ( 'NONE',  ( -2.248748702180634940, -25.49307895267003587, 6.700000000000000178 ) ) ;
#27551=CARTESIAN_POINT ( 'NONE',  ( 0.9213240864078056092, -26.64985754041175525, 6.700000000000000178 ) ) ;
#27553=LINE ( 'NONE', #14570, #13653 ) ;
#27558=ORIENTED_EDGE ( 'NONE', *, *, #19769, .T. ) ;
#27559=VERTEX_POINT ( 'NONE', #16809 ) ;
#27568=EDGE_CURVE ( 'NONE', #5299, #21616, #29776, .T. ) ;
#27570=EDGE_CURVE ( 'NONE', #9241, #37233, #23469, .T. ) ;
#27575=ORIENTED_EDGE ( 'NONE', *, *, #236, .F. ) ;
#27581=CARTESIAN_POINT ( 'NONE',  ( -53.21549048184568420, -30.38627270959228710, -4.152976064860135708 ) ) ;
#27598=ORIENTED_EDGE ( 'NONE', *, *, #28704, .F. ) ;
#27604=CARTESIAN_POINT ( 'NONE',  ( -6.348748702180634140, -25.49307895267003587, 6.800000000000000711 ) ) ;
#27606=CARTESIAN_POINT ( 'NONE',  ( -34.87867591359218977, -24.55319635012989110, 6.800000000000000711 ) ) ;
#27612=ORIENTED_EDGE ( 'NONE', *, *, #3654, .F. ) ;
#27614=LINE ( 'NONE', #49, #31836 ) ;
#27615=EDGE_CURVE ( 'NONE', #6790, #5705, #23210, .T. ) ;
#27618=PLANE ( 'NONE',  #35246 ) ;
#27629=DIRECTION ( 'NONE',  ( 1.000000000000000000, -0.000000000000000000, 0.000000000000000000 ) ) ;
#27632=ORIENTED_EDGE ( 'NONE', *, *, #1378, .T. ) ;
#27633=AXIS2_PLACEMENT_3D ( 'NONE', #33079, #29772, #2202 ) ;
#27638=LINE ( 'NONE', #21683, #19799 ) ;
#27652=DIRECTION ( 'NONE',  ( -0.000000000000000000, -0.000000000000000000, 1.000000000000000000 ) ) ;
#27664=CIRCLE ( 'NONE', #31622, 0.1000000000000028644 ) ;
#27666=LINE ( 'NONE', #40417, #16029 ) ;
#27667=LINE ( 'NONE', #295, #12743 ) ;
#27682=DIRECTION ( 'NONE',  ( 0.000000000000000000, 0.000000000000000000, 1.000000000000000000 ) ) ;
#27692=LINE ( 'NONE', #21330, #39325 ) ;
#27695=CARTESIAN_POINT ( 'NONE',  ( 0.9213240864078056092, -26.64985754041175525, 6.700000000000000178 ) ) ;
#27696=EDGE_CURVE ( 'NONE', #26593, #5299, #34672, .T. ) ;
#27699=EDGE_CURVE ( 'NONE', #33227, #7215, #1086, .T. ) ;
#27701=AXIS2_PLACEMENT_3D ( 'NONE', #32770, #35461, #17283 ) ;
#27704=ORIENTED_EDGE ( 'NONE', *, *, #26030, .F. ) ;
#27709=LINE ( 'NONE', #12886, #8224 ) ;
#27711=ADVANCED_FACE ( 'NONE', ( #10921 ), #8031, .T. ) ;
#27717=CARTESIAN_POINT ( 'NONE',  ( -8.348748702180635917, -26.64985754041175525, 6.800000000000000711 ) ) ;
#27719=CARTESIAN_POINT ( 'NONE',  ( -40.97867591359219119, -26.64985754041175525, 6.700000000000000178 ) ) ;
#27720=ORIENTED_EDGE ( 'NONE', *, *, #39453, .F. ) ;
#27725=VERTEX_POINT ( 'NONE', #1287 ) ;
#27726=EDGE_CURVE ( 'NONE', #25277, #35446, #22899, .T. ) ;
#27728=AXIS2_PLACEMENT_3D ( 'NONE', #33113, #27324, #26728 ) ;
#27729=DIRECTION ( 'NONE',  ( -1.000000000000000000, 0.000000000000000000, 0.000000000000000000 ) ) ;
#27733=PLANE ( 'NONE',  #35997 ) ;
#27737=EDGE_CURVE ( 'NONE', #10898, #19388, #38562, .T. ) ;
#27748=EDGE_CURVE ( 'NONE', #15627, #28082, #32577, .T. ) ;
#27755=DIRECTION ( 'NONE',  ( -0.000000000000000000, -0.000000000000000000, 1.000000000000000000 ) ) ;
#27765=PLANE ( 'NONE',  #4322 ) ;
#27766=ORIENTED_EDGE ( 'NONE', *, *, #14302, .F. ) ;
#27773=VERTEX_POINT ( 'NONE', #39124 ) ;
#27777=EDGE_LOOP ( 'NONE', ( #40216, #37246, #20847, #7521 ) ) ;
#27778=CARTESIAN_POINT ( 'NONE',  ( -20.87867591359218977, -26.64985754041175525, 6.700000000000000178 ) ) ;
#27781=CARTESIAN_POINT ( 'NONE',  ( -12.44874870218064267, -26.64985754041175525, 6.800000000000000711 ) ) ;
#27788=ORIENTED_EDGE ( 'NONE', *, *, #5864, .F. ) ;
#27794=ADVANCED_FACE ( 'NONE', ( #26584 ), #13824, .F. ) ;
#27802=DIRECTION ( 'NONE',  ( -0.000000000000000000, -0.000000000000000000, 1.000000000000000000 ) ) ;
#27826=CARTESIAN_POINT ( 'NONE',  ( 3.751251297819363728, -26.64985754041175525, 6.800000000000000711 ) ) ;
#27834=VECTOR ( 'NONE', #39567, 1000.000000000000000 ) ;
#27841=DIRECTION ( 'NONE',  ( -0.000000000000000000, -0.000000000000000000, 1.000000000000000000 ) ) ;
#27851=DIRECTION ( 'NONE',  ( -0.000000000000000000, -0.000000000000000000, 1.000000000000000000 ) ) ;
#27853=PLANE ( 'NONE',  #35168 ) ;
#27855=LINE ( 'NONE', #34476, #23355 ) ;
#27858=DIRECTION ( 'NONE',  ( 1.000000000000000000, 0.000000000000000000, 0.000000000000000000 ) ) ;
#27860=CARTESIAN_POINT ( 'NONE',  ( -26.44874870218064089, -26.64985754041175525, 6.800000000000000711 ) ) ;
#27862=ORIENTED_EDGE ( 'NONE', *, *, #5582, .T. ) ;
#27863=FACE_OUTER_BOUND ( 'NONE', #13098, .T. ) ;
#27865=AXIS2_PLACEMENT_3D ( 'NONE', #32802, #35492, #1709 ) ;
#27866=ORIENTED_EDGE ( 'NONE', *, *, #12820, .T. ) ;
#27868=DIRECTION ( 'NONE',  ( -0.000000000000000000, -1.000000000000000000, -0.000000000000000000 ) ) ;
#27870=LINE ( 'NONE', #17988, #38623 ) ;
#27887=EDGE_LOOP ( 'NONE', ( #14245, #18036, #3945, #21877 ) ) ;
#27892=CARTESIAN_POINT ( 'NONE',  ( -53.21549048184568420, -30.38627270959228710, 4.000000000000000000 ) ) ;
#27918=EDGE_CURVE ( 'NONE', #38404, #29405, #3478, .T. ) ;
#27922=VECTOR ( 'NONE', #27502, 1000.000000000000000 ) ;
#27927=CARTESIAN_POINT ( 'NONE',  ( 2.921324086407800280, -26.64985754041175525, 6.700000000000000178 ) ) ;
#27930=EDGE_LOOP ( 'NONE', ( #21292, #20542, #7179, #36739 ) ) ;
#27936=CARTESIAN_POINT ( 'NONE',  ( -29.07867591359219617, -26.64985754041175525, 6.700000000000000178 ) ) ;
#27940=VERTEX_POINT ( 'NONE', #31460 ) ;
#27948=CARTESIAN_POINT ( 'NONE',  ( -0.2487487021806331078, -26.64985754041175525, 6.800000000000000711 ) ) ;
#27949=ORIENTED_EDGE ( 'NONE', *, *, #4869, .F. ) ;
#27952=VECTOR ( 'NONE', #7773, 1000.000000000000000 ) ;
#27963=ORIENTED_EDGE ( 'NONE', *, *, #2853, .T. ) ;
#27965=DIRECTION ( 'NONE',  ( 1.000000000000000000, 0.000000000000000000, 0.000000000000000000 ) ) ;
#27970=VERTEX_POINT ( 'NONE', #22601 ) ;
#27974=EDGE_CURVE ( 'NONE', #5793, #30874, #29173, .T. ) ;
#27982=AXIS2_PLACEMENT_3D ( 'NONE', #35985, #1605, #38249 ) ;
#27986=DIRECTION ( 'NONE',  ( 0.000000000000000000, 0.000000000000000000, -1.000000000000000000 ) ) ;
#27989=ORIENTED_EDGE ( 'NONE', *, *, #1104, .T. ) ;
#27996=ORIENTED_EDGE ( 'NONE', *, *, #21970, .F. ) ;
#28007=LINE ( 'NONE', #21437, #22068 ) ;
#28010=DIRECTION ( 'NONE',  ( 0.000000000000000000, 0.000000000000000000, 1.000000000000000000 ) ) ;
#28012=ORIENTED_EDGE ( 'NONE', *, *, #20688, .F. ) ;
#28015=EDGE_LOOP ( 'NONE', ( #1528, #36675, #37777, #7225 ) ) ;
#28025=ORIENTED_EDGE ( 'NONE', *, *, #13576, .T. ) ;
#28042=EDGE_LOOP ( 'NONE', ( #37078, #18709, #14238, #37293 ) ) ;
#28043=CARTESIAN_POINT ( 'NONE',  ( -32.34874870218063592, -25.49307895267003587, 6.800000000000000711 ) ) ;
#28059=PLANE ( 'NONE',  #35438 ) ;
#28062=VECTOR ( 'NONE', #24599, 1000.000000000000000 ) ;
#28071=CARTESIAN_POINT ( 'NONE',  ( -14.24874870218063450, -26.64985754041175525, 6.700000000000000178 ) ) ;
#28077=PLANE ( 'NONE',  #28677 ) ;
#28082=VERTEX_POINT ( 'NONE', #38221 ) ;
#28087=ORIENTED_EDGE ( 'NONE', *, *, #25026, .T. ) ;
#28093=CARTESIAN_POINT ( 'NONE',  ( -18.44874870218064089, -26.64985754041175525, 6.700000000000000178 ) ) ;
#28097=ORIENTED_EDGE ( 'NONE', *, *, #1532, .F. ) ;
#28130=ORIENTED_EDGE ( 'NONE', *, *, #39302, .T. ) ;
#28131=CARTESIAN_POINT ( 'NONE',  ( -42.44874870218064444, -25.49307895267003587, 6.700000000000000178 ) ) ;
#28132=EDGE_CURVE ( 'NONE', #17194, #2391, #16239, .T. ) ;
#28136=AXIS2_PLACEMENT_3D ( 'NONE', #16859, #13582, #33350 ) ;
#28138=DIRECTION ( 'NONE',  ( 0.000000000000000000, 0.000000000000000000, 1.000000000000000000 ) ) ;
#28141=DIRECTION ( 'NONE',  ( 1.000000000000000000, 0.000000000000000000, 0.000000000000000000 ) ) ;
#28146=ORIENTED_EDGE ( 'NONE', *, *, #34910, .F. ) ;
#28154=VERTEX_POINT ( 'NONE', #16993 ) ;
#28155=FACE_OUTER_BOUND ( 'NONE', #19503, .T. ) ;
#28161=FACE_OUTER_BOUND ( 'NONE', #18853, .T. ) ;
#28164=EDGE_CURVE ( 'NONE', #22409, #13396, #2452, .T. ) ;
#28166=ORIENTED_EDGE ( 'NONE', *, *, #39181, .F. ) ;
#28179=EDGE_LOOP ( 'NONE', ( #20218, #35226, #23458, #5363 ) ) ;
#28182=ORIENTED_EDGE ( 'NONE', *, *, #37239, .T. ) ;
#28184=DIRECTION ( 'NONE',  ( -0.000000000000000000, -0.000000000000000000, 1.000000000000000000 ) ) ;
#28186=PLANE ( 'NONE',  #32178 ) ;
#28202=VECTOR ( 'NONE', #37001, 1000.000000000000000 ) ;
#28205=CARTESIAN_POINT ( 'NONE',  ( -28.97867591359219475, -24.55319635012989110, 6.800000000000000711 ) ) ;
#28211=VERTEX_POINT ( 'NONE', #18838 ) ;
#28213=CARTESIAN_POINT ( 'NONE',  ( -38.24874870218063450, -26.64985754041175525, 6.700000000000000178 ) ) ;
#28220=CARTESIAN_POINT ( 'NONE',  ( -20.24874870218063805, -26.64985754041175525, 6.700000000000000178 ) ) ;
#28225=FACE_BOUND ( 'NONE', #14233, .T. ) ;
#28230=DIRECTION ( 'NONE',  ( 0.000000000000000000, 0.000000000000000000, -1.000000000000000000 ) ) ;
#28263=FACE_OUTER_BOUND ( 'NONE', #5147, .T. ) ;
#28268=PLANE ( 'NONE',  #8312 ) ;
#28270=AXIS2_PLACEMENT_3D ( 'NONE', #8069, #17527, #11759 ) ;
#28272=ORIENTED_EDGE ( 'NONE', *, *, #3330, .T. ) ;
#28275=EDGE_CURVE ( 'NONE', #13485, #21972, #11821, .T. ) ;
#28279=ORIENTED_EDGE ( 'NONE', *, *, #9333, .T. ) ;
#28281=DIRECTION ( 'NONE',  ( 0.000000000000000000, 0.000000000000000000, 1.000000000000000000 ) ) ;
#28283=DIRECTION ( 'NONE',  ( 0.000000000000000000, 0.000000000000000000, 1.000000000000000000 ) ) ;
#28284=VERTEX_POINT ( 'NONE', #25027 ) ;
#28287=ORIENTED_EDGE ( 'NONE', *, *, #18209, .F. ) ;
#28292=CARTESIAN_POINT ( 'NONE',  ( -7.078675913592194391, -24.55319635012989110, 6.700000000000000178 ) ) ;
#28302=CARTESIAN_POINT ( 'NONE',  ( -11.07867591359219794, -26.64985754041175525, 6.700000000000000178 ) ) ;
#28309=CARTESIAN_POINT ( 'NONE',  ( -54.01549048184568846, -30.38627270959228710, -4.152976064860135708 ) ) ;
#28315=DIRECTION ( 'NONE',  ( 0.000000000000000000, 0.000000000000000000, 1.000000000000000000 ) ) ;
#28319=AXIS2_PLACEMENT_3D ( 'NONE', #228, #9891, #13184 ) ;
#28326=EDGE_LOOP ( 'NONE', ( #16737, #27362, #11241, #4842 ) ) ;
#28331=AXIS2_PLACEMENT_3D ( 'NONE', #2768, #15294, #30135 ) ;
#28333=VERTEX_POINT ( 'NONE', #13467 ) ;
#28341=ORIENTED_EDGE ( 'NONE', *, *, #10410, .T. ) ;
#28347=ORIENTED_EDGE ( 'NONE', *, *, #7073, .T. ) ;
#28355=EDGE_LOOP ( 'NONE', ( #15691, #12846, #18862, #11818 ) ) ;
#28356=LINE ( 'NONE', #3474, #22886 ) ;
#28364=DIRECTION ( 'NONE',  ( 0.000000000000000000, 1.000000000000000000, 0.000000000000000000 ) ) ;
#28365=ORIENTED_EDGE ( 'NONE', *, *, #28912, .T. ) ;
#28368=ORIENTED_EDGE ( 'NONE', *, *, #30981, .T. ) ;
#28371=ADVANCED_FACE ( 'NONE', ( #7292 ), #15952, .F. ) ;
#28375=ORIENTED_EDGE ( 'NONE', *, *, #7794, .F. ) ;
#28381=CARTESIAN_POINT ( 'NONE',  ( -28.87867591359219333, -26.64985754041175525, 6.800000000000000711 ) ) ;
#28382=CARTESIAN_POINT ( 'NONE',  ( -42.24874870218063450, -26.64985754041175525, 6.800000000000000711 ) ) ;
#28384=DIRECTION ( 'NONE',  ( 1.000000000000000000, 0.000000000000000000, 0.000000000000000000 ) ) ;
#28387=VECTOR ( 'NONE', #29017, 1000.000000000000000 ) ;
#28397=LINE ( 'NONE', #25322, #5534 ) ;
#28398=PLANE ( 'NONE',  #13421 ) ;
#28399=DIRECTION ( 'NONE',  ( 0.000000000000000000, 0.000000000000000000, 1.000000000000000000 ) ) ;
#28400=FACE_OUTER_BOUND ( 'NONE', #8210, .T. ) ;
#28407=VERTEX_POINT ( 'NONE', #26250 ) ;
#28412=ORIENTED_EDGE ( 'NONE', *, *, #22520, .F. ) ;
#28416=EDGE_CURVE ( 'NONE', #29405, #28154, #13625, .T. ) ;
#28425=ORIENTED_EDGE ( 'NONE', *, *, #36472, .F. ) ;
#28426=ORIENTED_EDGE ( 'NONE', *, *, #27748, .F. ) ;
#28428=DIRECTION ( 'NONE',  ( -1.000000000000000000, 0.000000000000000000, 0.000000000000000000 ) ) ;
#28431=ORIENTED_EDGE ( 'NONE', *, *, #3762, .T. ) ;
#28435=CARTESIAN_POINT ( 'NONE',  ( -5.078675913592192614, -24.55319635012989110, 6.700000000000000178 ) ) ;
#28437=FACE_BOUND ( 'NONE', #5334, .T. ) ;
#28455=EDGE_CURVE ( 'NONE', #39647, #37652, #19050, .T. ) ;
#28467=DIRECTION ( 'NONE',  ( 0.000000000000000000, 1.000000000000000000, 0.000000000000000000 ) ) ;
#28468=CARTESIAN_POINT ( 'NONE',  ( -18.44874870218064089, -25.49307895267003587, 6.800000000000000711 ) ) ;
#28482=LINE ( 'NONE', #22526, #25789 ) ;
#28484=CIRCLE ( 'NONE', #10709, 0.1000000000000028644 ) ;
#28500=DIRECTION ( 'NONE',  ( -0.000000000000000000, -0.000000000000000000, 1.000000000000000000 ) ) ;
#28508=VERTEX_POINT ( 'NONE', #28514 ) ;
#28510=ORIENTED_EDGE ( 'NONE', *, *, #12845, .F. ) ;
#28514=CARTESIAN_POINT ( 'NONE',  ( -40.87867591359218977, -26.64985754041175525, 6.800000000000000711 ) ) ;
#28528=CYLINDRICAL_SURFACE ( 'NONE', #2718, 0.1000000000000028644 ) ;
#28534=CARTESIAN_POINT ( 'NONE',  ( -6.448748702180637338, -26.64985754041175525, 6.700000000000000178 ) ) ;
#28541=CARTESIAN_POINT ( 'NONE',  ( -3.078675913592197944, -24.55319635012989110, 6.800000000000000711 ) ) ;
#28542=CARTESIAN_POINT ( 'NONE',  ( 4.921324086407802056, -26.64985754041175525, 6.800000000000000711 ) ) ;
#28543=VERTEX_POINT ( 'NONE', #3835 ) ;
#28544=LINE ( 'NONE', #35152, #39953 ) ;
#28548=ORIENTED_EDGE ( 'NONE', *, *, #17090, .T. ) ;
#28553=ORIENTED_EDGE ( 'NONE', *, *, #33410, .F. ) ;
#28554=EDGE_LOOP ( 'NONE', ( #21090, #203, #1752, #8299 ) ) ;
#28557=CIRCLE ( 'NONE', #325, 2.500000000000002220 ) ;
#28558=DIRECTION ( 'NONE',  ( -0.000000000000000000, -0.000000000000000000, 1.000000000000000000 ) ) ;
#28562=CARTESIAN_POINT ( 'NONE',  ( -32.44874870218063734, -25.49307895267003587, 6.700000000000000178 ) ) ;
#28566=ORIENTED_EDGE ( 'NONE', *, *, #23481, .F. ) ;
#28571=CARTESIAN_POINT ( 'NONE',  ( 11.65737507970504439, -32.06993018339339585, 6.800000000000000711 ) ) ;
#28575=DIRECTION ( 'NONE',  ( 1.000000000000000000, 0.000000000000000000, 0.000000000000000000 ) ) ;
#28579=EDGE_LOOP ( 'NONE', ( #19335, #31105, #5521, #3881 ) ) ;
#28595=VECTOR ( 'NONE', #1173, 1000.000000000000000 ) ;
#28598=ORIENTED_EDGE ( 'NONE', *, *, #29977, .F. ) ;
#28603=EDGE_LOOP ( 'NONE', ( #9977, #12355, #11488, #1858 ) ) ;
#28607=EDGE_CURVE ( 'NONE', #32868, #3311, #5017, .T. ) ;
#28610=DIRECTION ( 'NONE',  ( 1.000000000000000000, -0.000000000000000000, 0.000000000000000000 ) ) ;
#28620=ORIENTED_EDGE ( 'NONE', *, *, #10418, .T. ) ;
#28621=LINE ( 'NONE', #37868, #31380 ) ;
#28631=DIRECTION ( 'NONE',  ( -0.000000000000000000, -0.000000000000000000, 1.000000000000000000 ) ) ;
#28639=DIRECTION ( 'NONE',  ( 0.000000000000000000, 0.000000000000000000, 1.000000000000000000 ) ) ;
#28646=( NAMED_UNIT ( * ) SI_UNIT ( $, .STERADIAN. ) SOLID_ANGLE_UNIT ( ) );
#28647=EDGE_LOOP ( 'NONE', ( #34791, #4900, #24805, #31293 ) ) ;
#28648=FACE_BOUND ( 'NONE', #23225, .T. ) ;
#28649=( NAMED_UNIT ( * ) SI_UNIT ( $, .STERADIAN. ) SOLID_ANGLE_UNIT ( ) );
#28657=ORIENTED_EDGE ( 'NONE', *, *, #19980, .T. ) ;
#28663=CARTESIAN_POINT ( 'NONE',  ( -14.34874870218063769, -26.64985754041175525, 6.700000000000000178 ) ) ;
#28665=EDGE_CURVE ( 'NONE', #23338, #39035, #15620, .T. ) ;
#28670=DIRECTION ( 'NONE',  ( 0.000000000000000000, 0.000000000000000000, 1.000000000000000000 ) ) ;
#28673=CARTESIAN_POINT ( 'NONE',  ( -34.97867591359219830, -26.64985754041175525, 6.700000000000000178 ) ) ;
#28677=AXIS2_PLACEMENT_3D ( 'NONE', #3414, #32003, #9754 ) ;
#28679=LINE ( 'NONE', #3787, #8443 ) ;
#28685=EDGE_CURVE ( 'NONE', #38999, #16562, #18226, .T. ) ;
#28700=ORIENTED_EDGE ( 'NONE', *, *, #22004, .F. ) ;
#28701=DIRECTION ( 'NONE',  ( 0.000000000000000000, 0.000000000000000000, -1.000000000000000000 ) ) ;
#28704=EDGE_CURVE ( 'NONE', #31282, #29781, #29531, .T. ) ;
#28712=VECTOR ( 'NONE', #35464, 1000.000000000000000 ) ;
#28713=DIRECTION ( 'NONE',  ( -0.000000000000000000, -1.000000000000000000, -0.000000000000000000 ) ) ;
#28717=DIRECTION ( 'NONE',  ( 1.000000000000000000, 0.000000000000000000, 0.000000000000000000 ) ) ;
#28723=EDGE_LOOP ( 'NONE', ( #18681, #15514, #38074, #11374 ) ) ;
#28729=DIRECTION ( 'NONE',  ( 1.000000000000000000, 0.000000000000000000, 0.000000000000000000 ) ) ;
#28732=CARTESIAN_POINT ( 'NONE',  ( -21.07867591359219617, -26.64985754041175525, 6.700000000000000178 ) ) ;
#28735=CARTESIAN_POINT ( 'NONE',  ( -24.87867591359218977, -26.64985754041175525, 6.700000000000000178 ) ) ;
#28746=ORIENTED_EDGE ( 'NONE', *, *, #9799, .T. ) ;
#28749=CARTESIAN_POINT ( 'NONE',  ( 5.121324086407808451, -24.55319635012989110, 6.800000000000000711 ) ) ;
#28752=DIRECTION ( 'NONE',  ( -0.000000000000000000, -0.000000000000000000, 1.000000000000000000 ) ) ;
#28760=ORIENTED_EDGE ( 'NONE', *, *, #4934, .T. ) ;
#28764=CIRCLE ( 'NONE', #24800, 0.1000000000000028644 ) ;
#28766=AXIS2_PLACEMENT_3D ( 'NONE', #24772, #27447, #2767 ) ;
#28777=DIRECTION ( 'NONE',  ( 0.000000000000000000, 0.000000000000000000, 1.000000000000000000 ) ) ;
#28785=EDGE_CURVE ( 'NONE', #13485, #40691, #25473, .T. ) ;
#28792=CIRCLE ( 'NONE', #24851, 0.1000000000000028644 ) ;
#28800=VECTOR ( 'NONE', #22438, 1000.000000000000000 ) ;
#28802=ORIENTED_EDGE ( 'NONE', *, *, #25489, .T. ) ;
#28812=CARTESIAN_POINT ( 'NONE',  ( 11.65737507970504616, -30.94667987854474234, 6.800000000000000711 ) ) ;
#28815=FACE_OUTER_BOUND ( 'NONE', #17739, .T. ) ;
#28816=CARTESIAN_POINT ( 'NONE',  ( -7.078675913592194391, -26.64985754041175525, 6.700000000000000178 ) ) ;
#28820=ORIENTED_EDGE ( 'NONE', *, *, #23889, .F. ) ;
#28825=DIRECTION ( 'NONE',  ( 1.000000000000000000, 0.000000000000000000, 0.000000000000000000 ) ) ;
#28830=VECTOR ( 'NONE', #1152, 1000.000000000000000 ) ;
#28835=DIRECTION ( 'NONE',  ( 0.000000000000000000, 0.000000000000000000, 1.000000000000000000 ) ) ;
#28839=PLANE ( 'NONE',  #23067 ) ;
#28840=ADVANCED_FACE ( 'NONE', ( #40604 ), #34467, .F. ) ;
#28842=EDGE_LOOP ( 'NONE', ( #34032, #18975, #39506, #22651 ) ) ;
#28851=ORIENTED_EDGE ( 'NONE', *, *, #27568, .T. ) ;
#28856=CIRCLE ( 'NONE', #13745, 0.1000000000000028644 ) ;
#28861=CARTESIAN_POINT ( 'NONE',  ( -42.24874870218063450, -25.49307895267003587, 6.700000000000000178 ) ) ;
#28876=DIRECTION ( 'NONE',  ( 1.000000000000000000, 0.000000000000000000, 0.000000000000000000 ) ) ;
#28881=CARTESIAN_POINT ( 'NONE',  ( -24.97867591359219475, -26.64985754041175525, 6.700000000000000178 ) ) ;
#28887=AXIS2_PLACEMENT_3D ( 'NONE', #4766, #29879, #36460 ) ;
#28891=ORIENTED_EDGE ( 'NONE', *, *, #23445, .T. ) ;
#28893=LINE ( 'NONE', #35290, #11287 ) ;
#28895=VERTEX_POINT ( 'NONE', #15086 ) ;
#28901=CARTESIAN_POINT ( 'NONE',  ( -2.348748702180637693, -25.49307895267003587, 6.700000000000000178 ) ) ;
#28906=DIRECTION ( 'NONE',  ( 0.000000000000000000, 0.000000000000000000, 1.000000000000000000 ) ) ;
#28912=EDGE_CURVE ( 'NONE', #9101, #6453, #510, .T. ) ;
#28920=DIRECTION ( 'NONE',  ( 0.000000000000000000, 0.000000000000000000, 1.000000000000000000 ) ) ;
#28928=CARTESIAN_POINT ( 'NONE',  ( -8.348748702180635917, -26.64985754041175525, 6.700000000000000178 ) ) ;
#28940=LINE ( 'NONE', #38589, #30832 ) ;
#28948=CARTESIAN_POINT ( 'NONE',  ( 5.651251297819362307, -25.49307895267003587, 6.800000000000000711 ) ) ;
#28956=AXIS2_PLACEMENT_3D ( 'NONE', #9366, #38183, #32038 ) ;
#28962=DIRECTION ( 'NONE',  ( -0.000000000000000000, -0.000000000000000000, 1.000000000000000000 ) ) ;
#28992=CARTESIAN_POINT ( 'NONE',  ( -38.44874870218063734, -26.64985754041175525, 6.700000000000000178 ) ) ;
#29000=LINE ( 'NONE', #17019, #8905 ) ;
#29001=ORIENTED_EDGE ( 'NONE', *, *, #30981, .F. ) ;
#29009=ORIENTED_EDGE ( 'NONE', *, *, #13822, .T. ) ;
#29010=ORIENTED_EDGE ( 'NONE', *, *, #18030, .T. ) ;
#29011=EDGE_CURVE ( 'NONE', #4935, #36016, #24134, .T. ) ;
#29012=ADVANCED_FACE ( 'NONE', ( #35472 ), #19005, .F. ) ;
#29017=DIRECTION ( 'NONE',  ( -0.000000000000000000, -0.000000000000000000, 1.000000000000000000 ) ) ;
#29039=CARTESIAN_POINT ( 'NONE',  ( 5.021324086407805254, -26.64985754041175525, 6.800000000000000711 ) ) ;
#29041=AXIS2_PLACEMENT_3D ( 'NONE', #20768, #33364, #20562 ) ;
#29044=EDGE_LOOP ( 'NONE', ( #32254, #13251, #20140, #27149 ) ) ;
#29049=ORIENTED_EDGE ( 'NONE', *, *, #5523, .F. ) ;
#29053=FACE_BOUND ( 'NONE', #35117, .T. ) ;
#29055=ORIENTED_EDGE ( 'NONE', *, *, #29741, .F. ) ;
#29056=ADVANCED_FACE ( 'NONE', ( #3583 ), #25992, .F. ) ;
#29076=LINE ( 'NONE', #35869, #17473 ) ;
#29083=CARTESIAN_POINT ( 'NONE',  ( -39.07867591359219261, -26.64985754041175525, 6.800000000000000711 ) ) ;
#29111=ORIENTED_EDGE ( 'NONE', *, *, #36561, .F. ) ;
#29125=CARTESIAN_POINT ( 'NONE',  ( -22.87867591359218977, -24.55319635012989110, 6.700000000000000178 ) ) ;
#29127=AXIS2_PLACEMENT_3D ( 'NONE', #27274, #39416, #36348 ) ;
#29130=DIRECTION ( 'NONE',  ( -0.000000000000000000, -0.000000000000000000, 1.000000000000000000 ) ) ;
#29134=DIRECTION ( 'NONE',  ( 0.000000000000000000, 0.000000000000000000, 1.000000000000000000 ) ) ;
#29137=PLANE ( 'NONE',  #13194 ) ;
#29149=VERTEX_POINT ( 'NONE', #10526 ) ;
#29156=ORIENTED_EDGE ( 'NONE', *, *, #25453, .T. ) ;
#29163=LINE ( 'NONE', #3875, #6112 ) ;
#29164=ADVANCED_FACE ( 'NONE', ( #1293 ), #13831, .F. ) ;
#29171=ORIENTED_EDGE ( 'NONE', *, *, #37500, .T. ) ;
#29173=LINE ( 'NONE', #38024, #35344 ) ;
#29174=AXIS2_PLACEMENT_3D ( 'NONE', #5890, #18426, #2819 ) ;
#29177=FACE_OUTER_BOUND ( 'NONE', #35328, .T. ) ;
#29180=DIRECTION ( 'NONE',  ( 1.000000000000000000, 0.000000000000000000, 0.000000000000000000 ) ) ;
#29188=VERTEX_POINT ( 'NONE', #15443 ) ;
#29199=ORIENTED_EDGE ( 'NONE', *, *, #33812, .F. ) ;
#29204=VERTEX_POINT ( 'NONE', #21224 ) ;
#29206=DIRECTION ( 'NONE',  ( -0.000000000000000000, -0.000000000000000000, 1.000000000000000000 ) ) ;
#29208=VERTEX_POINT ( 'NONE', #24302 ) ;
#29210=DIRECTION ( 'NONE',  ( 1.000000000000000000, 0.000000000000000000, -0.000000000000000000 ) ) ;
#29212=VECTOR ( 'NONE', #7921, 1000.000000000000000 ) ;
#29215=DIRECTION ( 'NONE',  ( 1.000000000000000000, 0.000000000000000000, 0.000000000000000000 ) ) ;
#29240=CARTESIAN_POINT ( 'NONE',  ( -42.83131703149249603, -27.06993018339339585, 6.000000000000000000 ) ) ;
#29253=ORIENTED_EDGE ( 'NONE', *, *, #26189, .F. ) ;
#29264=VECTOR ( 'NONE', #2573, 1000.000000000000000 ) ;
#29266=CARTESIAN_POINT ( 'NONE',  ( 1.651251297819358754, -25.49307895267003587, 6.800000000000000711 ) ) ;
#29270=FACE_OUTER_BOUND ( 'NONE', #4677, .T. ) ;
#29291=CYLINDRICAL_SURFACE ( 'NONE', #18459, 0.1000000000000028644 ) ;
#29297=LINE ( 'NONE', #1111, #8682 ) ;
#29300=FACE_BOUND ( 'NONE', #38400, .T. ) ;
#29311=CARTESIAN_POINT ( 'NONE',  ( -36.87867591359218977, -26.64985754041175525, 6.700000000000000178 ) ) ;
#29312=VERTEX_POINT ( 'NONE', #3338 ) ;
#29340=ORIENTED_EDGE ( 'NONE', *, *, #14720, .T. ) ;
#29343=EDGE_CURVE ( 'NONE', #17770, #1874, #35227, .T. ) ;
#29348=AXIS2_PLACEMENT_3D ( 'NONE', #24850, #8360, #33520 ) ;
#29356=VERTEX_POINT ( 'NONE', #9685 ) ;
#29375=LINE ( 'NONE', #7146, #12925 ) ;
#29380=CARTESIAN_POINT ( 'NONE',  ( -32.24874870218063450, -26.64985754041175525, 6.700000000000000178 ) ) ;
#29381=AXIS2_PLACEMENT_3D ( 'NONE', #25006, #25816, #34704 ) ;
#29383=AXIS2_PLACEMENT_3D ( 'NONE', #33497, #20491, #23782 ) ;
#29392=DIRECTION ( 'NONE',  ( 0.000000000000000000, 0.000000000000000000, 1.000000000000000000 ) ) ;
#29394=EDGE_CURVE ( 'NONE', #4265, #20273, #22055, .T. ) ;
#29400=LINE ( 'NONE', #3359, #33804 ) ;
#29401=CARTESIAN_POINT ( 'NONE',  ( -6.878675913592188884, -26.64985754041175525, 6.700000000000000178 ) ) ;
#29402=VERTEX_POINT ( 'NONE', #6610 ) ;
#29403=DIRECTION ( 'NONE',  ( 0.000000000000000000, 1.000000000000000000, 0.000000000000000000 ) ) ;
#29405=VERTEX_POINT ( 'NONE', #19365 ) ;
#29410=CARTESIAN_POINT ( 'NONE',  ( -14.44874870218064089, -26.64985754041175525, 6.800000000000000711 ) ) ;
#29414=EDGE_LOOP ( 'NONE', ( #37459, #20996, #22289, #25903 ) ) ;
#29415=VECTOR ( 'NONE', #14846, 1000.000000000000000 ) ;
#29420=DIRECTION ( 'NONE',  ( 1.000000000000000000, 0.000000000000000000, 0.000000000000000000 ) ) ;
#29430=DIRECTION ( 'NONE',  ( 0.000000000000000000, 0.000000000000000000, 1.000000000000000000 ) ) ;
#29433=EDGE_CURVE ( 'NONE', #38404, #1672, #15863, .T. ) ;
#29438=DIRECTION ( 'NONE',  ( 0.000000000000000000, 0.000000000000000000, 1.000000000000000000 ) ) ;
#29442=DIRECTION ( 'NONE',  ( 0.000000000000000000, 0.000000000000000000, 1.000000000000000000 ) ) ;
#29444=CARTESIAN_POINT ( 'NONE',  ( -26.24874870218063450, -26.64985754041175525, 6.700000000000000178 ) ) ;
#29445=EDGE_CURVE ( 'NONE', #29149, #39054, #37667, .T. ) ;
#29454=CARTESIAN_POINT ( 'NONE',  ( -32.34874870218063592, -26.64985754041175525, 6.700000000000000178 ) ) ;
#29458=ORIENTED_EDGE ( 'NONE', *, *, #30973, .T. ) ;
#29464=VERTEX_POINT ( 'NONE', #16064 ) ;
#29466=DIRECTION ( 'NONE',  ( 1.000000000000000000, -0.000000000000000000, 0.000000000000000000 ) ) ;
#29472=DIRECTION ( 'NONE',  ( 0.000000000000000000, 0.000000000000000000, 1.000000000000000000 ) ) ;
#29479=EDGE_CURVE ( 'NONE', #10139, #32700, #30778, .T. ) ;
#29491=AXIS2_PLACEMENT_3D ( 'NONE', #23826, #20537, #8174 ) ;
#29494=DIRECTION ( 'NONE',  ( 1.000000000000000000, 0.000000000000000000, 0.000000000000000000 ) ) ;
#29495=ORIENTED_EDGE ( 'NONE', *, *, #24174, .T. ) ;
#29506=LINE ( 'NONE', #20618, #37853 ) ;
#29514=VERTEX_POINT ( 'NONE', #26548 ) ;
#29517=CARTESIAN_POINT ( 'NONE',  ( -8.248748702180632719, -26.64985754041175525, 6.700000000000000178 ) ) ;
#29520=ADVANCED_FACE ( 'NONE', ( #23840 ), #5126, .F. ) ;
#29521=LINE ( 'NONE', #10373, #14201 ) ;
#29522=EDGE_CURVE ( 'NONE', #24427, #5530, #11007, .T. ) ;
#29531=LINE ( 'NONE', #13878, #22198 ) ;
#29538=CARTESIAN_POINT ( 'NONE',  ( 5.121324086407808451, -26.64985754041175525, 6.700000000000000178 ) ) ;
#29542=ORIENTED_EDGE ( 'NONE', *, *, #34503, .F. ) ;
#29547=ORIENTED_EDGE ( 'NONE', *, *, #2406, .T. ) ;
#29550=CARTESIAN_POINT ( 'NONE',  ( -22.34874870218063947, -26.64985754041175525, 6.700000000000000178 ) ) ;
#29553=ORIENTED_EDGE ( 'NONE', *, *, #24649, .F. ) ;
#29558=CARTESIAN_POINT ( 'NONE',  ( -16.87867591359218977, -26.64985754041175525, 6.700000000000000178 ) ) ;
#29564=ORIENTED_EDGE ( 'NONE', *, *, #13822, .F. ) ;
#29565=LINE ( 'NONE', #39220, #27490 ) ;
#29567=ORIENTED_EDGE ( 'NONE', *, *, #7328, .F. ) ;
#29570=EDGE_CURVE ( 'NONE', #1634, #22687, #33424, .T. ) ;
#29582=CARTESIAN_POINT ( 'NONE',  ( -10.87867591359219155, -24.55319635012989110, 6.700000000000000178 ) ) ;
#29583=CARTESIAN_POINT ( 'NONE',  ( -4.248748702180636272, -25.49307895267003587, 6.700000000000000178 ) ) ;
#29597=DIRECTION ( 'NONE',  ( 1.000000000000000000, -0.000000000000000000, 0.000000000000000000 ) ) ;
#29611=ORIENTED_EDGE ( 'NONE', *, *, #6814, .F. ) ;
#29616=VECTOR ( 'NONE', #36873, 1000.000000000000000 ) ;
#29618=ADVANCED_FACE ( 'NONE', ( #24462 ), #21595, .F. ) ;
#29619=CARTESIAN_POINT ( 'NONE',  ( -44.23414840393349579, -23.60493063168010153, 6.000000000000000000 ) ) ;
#29624=DIRECTION ( 'NONE',  ( -1.000000000000000000, 0.000000000000000000, 0.000000000000000000 ) ) ;
#29628=DIRECTION ( 'NONE',  ( -0.000000000000000000, -1.000000000000000000, -0.000000000000000000 ) ) ;
#29635=DIRECTION ( 'NONE',  ( -0.000000000000000000, -0.000000000000000000, 1.000000000000000000 ) ) ;
#29636=CIRCLE ( 'NONE', #14487, 0.1000000000000028644 ) ;
#29646=VERTEX_POINT ( 'NONE', #39907 ) ;
#29647=CIRCLE ( 'NONE', #28331, 0.1000000000000028644 ) ;
#29659=CARTESIAN_POINT ( 'NONE',  ( -51.21549048184568420, -38.28842912540938670, 6.000000000000000000 ) ) ;
#29665=EDGE_CURVE ( 'NONE', #14626, #37912, #27553, .T. ) ;
#29674=ORIENTED_EDGE ( 'NONE', *, *, #38567, .F. ) ;
#29679=DIRECTION ( 'NONE',  ( 1.000000000000000000, 0.000000000000000000, 0.000000000000000000 ) ) ;
#29690=ORIENTED_EDGE ( 'NONE', *, *, #16673, .T. ) ;
#29695=ADVANCED_FACE ( 'NONE', ( #2471 ), #12095, .F. ) ;
#29698=ORIENTED_EDGE ( 'NONE', *, *, #35409, .F. ) ;
#29704=AXIS2_PLACEMENT_3D ( 'NONE', #22444, #28610, #27986 ) ;
#29714=EDGE_CURVE ( 'NONE', #26905, #28895, #16928, .T. ) ;
#29724=ORIENTED_EDGE ( 'NONE', *, *, #7770, .F. ) ;
#29740=VECTOR ( 'NONE', #15309, 1000.000000000000000 ) ;
#29741=EDGE_CURVE ( 'NONE', #5741, #28543, #14573, .T. ) ;
#29745=ADVANCED_FACE ( 'NONE', ( #23664 ), #26963, .F. ) ;
#29746=LINE ( 'NONE', #1558, #29212 ) ;
#29747=DIRECTION ( 'NONE',  ( 0.000000000000000000, 0.000000000000000000, 1.000000000000000000 ) ) ;
#29748=ORIENTED_EDGE ( 'NONE', *, *, #37145, .T. ) ;
#29751=CYLINDRICAL_SURFACE ( 'NONE', #40105, 0.1000000000000028644 ) ;
#29754=DIRECTION ( 'NONE',  ( 0.000000000000000000, 0.000000000000000000, -1.000000000000000000 ) ) ;
#29757=FACE_OUTER_BOUND ( 'NONE', #26767, .T. ) ;
#29760=ORIENTED_EDGE ( 'NONE', *, *, #11518, .T. ) ;
#29761=CARTESIAN_POINT ( 'NONE',  ( -20.44874870218064444, -26.64985754041175525, 6.700000000000000178 ) ) ;
#29770=LINE ( 'NONE', #7076, #20598 ) ;
#29772=DIRECTION ( 'NONE',  ( 0.000000000000000000, 0.000000000000000000, 1.000000000000000000 ) ) ;
#29773=AXIS2_PLACEMENT_3D ( 'NONE', #33319, #5101, #17632 ) ;
#29775=CARTESIAN_POINT ( 'NONE',  ( -26.24874870218063450, -26.64985754041175525, 6.700000000000000178 ) ) ;
#29776=LINE ( 'NONE', #14324, #482 ) ;
#29781=VERTEX_POINT ( 'NONE', #26469 ) ;
#29804=AXIS2_PLACEMENT_3D ( 'NONE', #32478, #13737, #32878 ) ;
#29809=CARTESIAN_POINT ( 'NONE',  ( -10.24874870218063450, -25.49307895267003587, 6.700000000000000178 ) ) ;
#29812=ORIENTED_EDGE ( 'NONE', *, *, #5823, .T. ) ;
#29821=DIRECTION ( 'NONE',  ( -0.000000000000000000, -0.000000000000000000, -1.000000000000000000 ) ) ;
#29823=ADVANCED_FACE ( 'NONE', ( #9090 ), #2954, .F. ) ;
#29827=CARTESIAN_POINT ( 'NONE',  ( -22.34874870218063947, -26.64985754041175525, 6.700000000000000178 ) ) ;
#29828=DIRECTION ( 'NONE',  ( 0.000000000000000000, 0.000000000000000000, 1.000000000000000000 ) ) ;
#29834=AXIS2_PLACEMENT_3D ( 'NONE', #34859, #6635, #31747 ) ;
#29840=DIRECTION ( 'NONE',  ( 0.000000000000000000, 1.000000000000000000, 0.000000000000000000 ) ) ;
#29842=EDGE_CURVE ( 'NONE', #19316, #1269, #22226, .T. ) ;
#29845=ORIENTED_EDGE ( 'NONE', *, *, #27737, .T. ) ;
#29847=ORIENTED_EDGE ( 'NONE', *, *, #39545, .F. ) ;
#29849=VECTOR ( 'NONE', #9097, 1000.000000000000000 ) ;
#29850=SHAPE_REPRESENTATION_RELATIONSHIP ( 'NONE' , 'NONE' ,  #39533, #22994 ) ;
#29858=FACE_OUTER_BOUND ( 'NONE', #35236, .T. ) ;
#29860=DIRECTION ( 'NONE',  ( 0.000000000000000000, 1.000000000000000000, 0.000000000000000000 ) ) ;
#29873=CARTESIAN_POINT ( 'NONE',  ( -0.2487487021806331078, -25.49307895267003587, 6.700000000000000178 ) ) ;
#29875=VECTOR ( 'NONE', #26356, 1000.000000000000000 ) ;
#29879=DIRECTION ( 'NONE',  ( -1.000000000000000000, 0.000000000000000000, 0.000000000000000000 ) ) ;
#29884=FACE_OUTER_BOUND ( 'NONE', #38969, .T. ) ;
#29885=ORIENTED_EDGE ( 'NONE', *, *, #34007, .F. ) ;
#29887=DIRECTION ( 'NONE',  ( 1.000000000000000000, 0.000000000000000000, 0.000000000000000000 ) ) ;
#29890=AXIS2_PLACEMENT_3D ( 'NONE', #26801, #5579, #2517 ) ;
#29895=EDGE_CURVE ( 'NONE', #21734, #301, #33381, .T. ) ;
#29899=LINE ( 'NONE', #11547, #21876 ) ;
#29903=VECTOR ( 'NONE', #12168, 1000.000000000000000 ) ;
#29922=CIRCLE ( 'NONE', #16775, 0.1000000000000028644 ) ;
#29926=CARTESIAN_POINT ( 'NONE',  ( -30.87867591359218977, -24.55319635012989110, 6.700000000000000178 ) ) ;
#29931=PLANE ( 'NONE',  #18072 ) ;
#29934=DIRECTION ( 'NONE',  ( -0.000000000000000000, -0.000000000000000000, 1.000000000000000000 ) ) ;
#29936=ORIENTED_EDGE ( 'NONE', *, *, #30824, .T. ) ;
#29939=ORIENTED_EDGE ( 'NONE', *, *, #39181, .T. ) ;
#29942=EDGE_CURVE ( 'NONE', #2870, #4585, #9446, .T. ) ;
#29943=EDGE_CURVE ( 'NONE', #37531, #1662, #15221, .T. ) ;
#29945=PLANE ( 'NONE',  #16898 ) ;
#29949=DIRECTION ( 'NONE',  ( -0.000000000000000000, 1.000000000000000000, -0.000000000000000000 ) ) ;
#29950=VECTOR ( 'NONE', #23600, 1000.000000000000000 ) ;
#29951=AXIS2_PLACEMENT_3D ( 'NONE', #31283, #34796, #37434 ) ;
#29953=ORIENTED_EDGE ( 'NONE', *, *, #10637, .T. ) ;
#29954=EDGE_LOOP ( 'NONE', ( #27072, #20565, #38110, #9223 ) ) ;
#29960=VECTOR ( 'NONE', #18859, 1000.000000000000000 ) ;
#29977=EDGE_CURVE ( 'NONE', #10008, #25619, #32314, .T. ) ;
#29978=ADVANCED_FACE ( 'NONE', ( #20523 ), #30212, .F. ) ;
#29986=CIRCLE ( 'NONE', #17502, 0.1000000000000028644 ) ;
#29987=ORIENTED_EDGE ( 'NONE', *, *, #19032, .F. ) ;
#29997=DIRECTION ( 'NONE',  ( 0.000000000000000000, 0.000000000000000000, 1.000000000000000000 ) ) ;
#30005=DIRECTION ( 'NONE',  ( 0.000000000000000000, 0.000000000000000000, 1.000000000000000000 ) ) ;
#30009=DIRECTION ( 'NONE',  ( 0.000000000000000000, 0.000000000000000000, 1.000000000000000000 ) ) ;
#30010=CYLINDRICAL_SURFACE ( 'NONE', #30474, 0.1000000000000028644 ) ;
#30012=DIRECTION ( 'NONE',  ( 1.000000000000000000, -0.000000000000000000, 0.000000000000000000 ) ) ;
#30014=DIRECTION ( 'NONE',  ( -1.000000000000000000, 0.000000000000000000, 0.000000000000000000 ) ) ;
#30018=LINE ( 'NONE', #1836, #17809 ) ;
#30019=EDGE_CURVE ( 'NONE', #24473, #160, #36296, .T. ) ;
#30028=PLANE ( 'NONE',  #4287 ) ;
#30030=CARTESIAN_POINT ( 'NONE',  ( 11.65737507970504439, -29.56993018339339940, 6.800000000000000711 ) ) ;
#30031=EDGE_CURVE ( 'NONE', #39661, #25969, #18949, .T. ) ;
#30044=ORIENTED_EDGE ( 'NONE', *, *, #33332, .T. ) ;
#30050=VECTOR ( 'NONE', #39436, 1000.000000000000000 ) ;
#30053=ORIENTED_EDGE ( 'NONE', *, *, #6804, .T. ) ;
#30058=DIRECTION ( 'NONE',  ( 1.000000000000000000, 0.000000000000000000, 0.000000000000000000 ) ) ;
#30074=VERTEX_POINT ( 'NONE', #25162 ) ;
#30075=DIRECTION ( 'NONE',  ( 0.000000000000000000, 1.000000000000000000, 0.000000000000000000 ) ) ;
#30078=CARTESIAN_POINT ( 'NONE',  ( -41.07867591359219972, -26.64985754041175525, 6.700000000000000178 ) ) ;
#30087=AXIS2_PLACEMENT_3D ( 'NONE', #17426, #30014, #26924 ) ;
#30088=ADVANCED_FACE ( 'NONE', ( #24966 ), #34452, .T. ) ;
#30092=DIRECTION ( 'NONE',  ( -0.000000000000000000, -0.000000000000000000, 1.000000000000000000 ) ) ;
#30105=CARTESIAN_POINT ( 'NONE',  ( 1.121324086407811338, -26.64985754041175525, 6.700000000000000178 ) ) ;
#30112=FACE_OUTER_BOUND ( 'NONE', #9476, .T. ) ;
#30114=ORIENTED_EDGE ( 'NONE', *, *, #16102, .T. ) ;
#30119=ORIENTED_EDGE ( 'NONE', *, *, #33012, .F. ) ;
#30125=CARTESIAN_POINT ( 'NONE',  ( -9.078675913592196167, -24.55319635012989110, 6.800000000000000711 ) ) ;
#30135=DIRECTION ( 'NONE',  ( 1.000000000000000000, 0.000000000000000000, 0.000000000000000000 ) ) ;
#30140=DIRECTION ( 'NONE',  ( 0.000000000000000000, 0.000000000000000000, 1.000000000000000000 ) ) ;
#30141=FACE_OUTER_BOUND ( 'NONE', #12144, .T. ) ;
#30148=ORIENTED_EDGE ( 'NONE', *, *, #15482, .F. ) ;
#30154=DIRECTION ( 'NONE',  ( -0.000000000000000000, -1.000000000000000000, -0.000000000000000000 ) ) ;
#30155=ADVANCED_FACE ( 'NONE', ( #8562 ), #33709, .F. ) ;
#30160=EDGE_LOOP ( 'NONE', ( #32820, #29055, #20876, #19774 ) ) ;
#30174=EDGE_CURVE ( 'NONE', #15627, #8458, #12889, .T. ) ;
#30179=DIRECTION ( 'NONE',  ( 0.000000000000000000, 0.000000000000000000, 1.000000000000000000 ) ) ;
#30183=CARTESIAN_POINT ( 'NONE',  ( -30.87867591359218977, -26.64985754041175525, 6.700000000000000178 ) ) ;
#30188=VECTOR ( 'NONE', #28467, 1000.000000000000000 ) ;
#30197=DIRECTION ( 'NONE',  ( 1.000000000000000000, 0.000000000000000000, 0.000000000000000000 ) ) ;
#30200=VERTEX_POINT ( 'NONE', #3858 ) ;
#30201=AXIS2_PLACEMENT_3D ( 'NONE', #6933, #22396, #10419 ) ;
#30202=ORIENTED_EDGE ( 'NONE', *, *, #13623, .F. ) ;
#30206=ADVANCED_FACE ( 'NONE', ( #36681 ), #21047, .T. ) ;
#30212=CYLINDRICAL_SURFACE ( 'NONE', #1216, 0.1000000000000028644 ) ;
#30218=DIRECTION ( 'NONE',  ( -0.000000000000000000, -0.000000000000000000, 1.000000000000000000 ) ) ;
#30219=PLANE ( 'NONE',  #25198 ) ;
#30222=CYLINDRICAL_SURFACE ( 'NONE', #40619, 2.000000000000000000 ) ;
#30236=AXIS2_PLACEMENT_3D ( 'NONE', #11833, #24204, #12255 ) ;
#30244=ADVANCED_FACE ( 'NONE', ( #19782 ), #13390, .F. ) ;
#30249=CARTESIAN_POINT ( 'NONE',  ( -1.078675913592196167, -26.64985754041175525, 6.800000000000000711 ) ) ;
#30251=CARTESIAN_POINT ( 'NONE',  ( 0.000000000000000000, -30.38627270959228710, 0.000000000000000000 ) ) ;
#30254=EDGE_LOOP ( 'NONE', ( #5423, #27788, #26321, #796 ) ) ;
#30255=ADVANCED_FACE ( 'NONE', ( #26371 ), #13731, .F. ) ;
#30257=LINE ( 'NONE', #12893, #12802 ) ;
#30269=EDGE_LOOP ( 'NONE', ( #3303, #13722, #10070, #18453 ) ) ;
#30282=CIRCLE ( 'NONE', #38184, 0.1000000000000028644 ) ;
#30287=DIRECTION ( 'NONE',  ( 0.000000000000000000, 1.000000000000000000, 0.000000000000000000 ) ) ;
#30288=DIRECTION ( 'NONE',  ( -0.000000000000000000, -1.000000000000000000, -0.000000000000000000 ) ) ;
#30291=DIRECTION ( 'NONE',  ( 1.000000000000000000, 0.000000000000000000, 0.000000000000000000 ) ) ;
#30295=AXIS2_PLACEMENT_3D ( 'NONE', #39088, #10885, #3946 ) ;
#30296=ORIENTED_EDGE ( 'NONE', *, *, #4514, .T. ) ;
#30303=EDGE_LOOP ( 'NONE', ( #3257, #34199, #37266, #35094 ) ) ;
#30309=DIRECTION ( 'NONE',  ( -0.000000000000000000, -0.000000000000000000, -1.000000000000000000 ) ) ;
#30310=PLANE ( 'NONE',  #33721 ) ;
#30319=CARTESIAN_POINT ( 'NONE',  ( 7.121324086407810228, -26.64985754041175525, 6.700000000000000178 ) ) ;
#30328=VERTEX_POINT ( 'NONE', #7340 ) ;
#30336=CARTESIAN_POINT ( 'NONE',  ( -18.87867591359219333, -24.55319635012989110, 6.700000000000000178 ) ) ;
#30352=CARTESIAN_POINT ( 'NONE',  ( -18.87867591359219333, -24.55319635012989110, 6.800000000000000711 ) ) ;
#30353=CARTESIAN_POINT ( 'NONE',  ( -18.24874870218063450, -26.64985754041175525, 6.700000000000000178 ) ) ;
#30362=DIRECTION ( 'NONE',  ( -1.000000000000000000, 0.000000000000000000, 0.000000000000000000 ) ) ;
#30363=VECTOR ( 'NONE', #19340, 1000.000000000000000 ) ;
#30365=DIRECTION ( 'NONE',  ( 0.000000000000000000, 1.000000000000000000, 0.000000000000000000 ) ) ;
#30372=DIRECTION ( 'NONE',  ( 0.000000000000000000, 0.000000000000000000, -1.000000000000000000 ) ) ;
#30377=CARTESIAN_POINT ( 'NONE',  ( -30.87867591359218977, -26.64985754041175525, 6.700000000000000178 ) ) ;
#30395=LINE ( 'NONE', #2621, #36816 ) ;
#30396=AXIS2_PLACEMENT_3D ( 'NONE', #31733, #36424, #17459 ) ;
#30398=DIRECTION ( 'NONE',  ( 0.000000000000000000, 1.000000000000000000, 0.000000000000000000 ) ) ;
#30400=VERTEX_POINT ( 'NONE', #22806 ) ;
#30406=LINE ( 'NONE', #11853, #31179 ) ;
#30411=ORIENTED_EDGE ( 'NONE', *, *, #6055, .F. ) ;
#30418=VECTOR ( 'NONE', #20829, 1000.000000000000000 ) ;
#30422=DIRECTION ( 'NONE',  ( -0.000000000000000000, -0.000000000000000000, 1.000000000000000000 ) ) ;
#30426=LINE ( 'NONE', #14975, #21158 ) ;
#30430=DIRECTION ( 'NONE',  ( 0.000000000000000000, 0.000000000000000000, -1.000000000000000000 ) ) ;
#30436=CARTESIAN_POINT ( 'NONE',  ( -40.87867591359218977, -26.64985754041175525, 6.700000000000000178 ) ) ;
#30449=VECTOR ( 'NONE', #24067, 1000.000000000000000 ) ;
#30464=CARTESIAN_POINT ( 'NONE',  ( -22.44874870218064089, -25.49307895267003587, 6.800000000000000711 ) ) ;
#30474=AXIS2_PLACEMENT_3D ( 'NONE', #12073, #8581, #21776 ) ;
#30475=CARTESIAN_POINT ( 'NONE',  ( -26.44874870218064089, -25.49307895267003587, 6.800000000000000711 ) ) ;
#30479=DIRECTION ( 'NONE',  ( 1.000000000000000000, 0.000000000000000000, 0.000000000000000000 ) ) ;
#30483=EDGE_CURVE ( 'NONE', #5741, #21149, #1783, .T. ) ;
#30492=ORIENTED_EDGE ( 'NONE', *, *, #25488, .T. ) ;
#30495=CIRCLE ( 'NONE', #29804, 0.1000000000000028644 ) ;
#30496=PLANE ( 'NONE',  #28887 ) ;
#30500=ADVANCED_FACE ( 'NONE', ( #23985 ), #23781, .F. ) ;
#30501=CARTESIAN_POINT ( 'NONE',  ( -14.34874870218063769, -25.49307895267003587, 6.700000000000000178 ) ) ;
#30503=FACE_OUTER_BOUND ( 'NONE', #30905, .T. ) ;
#30506=EDGE_LOOP ( 'NONE', ( #30802, #33987, #21109, #22635 ) ) ;
#30515=FACE_OUTER_BOUND ( 'NONE', #30303, .T. ) ;
#30525=FACE_OUTER_BOUND ( 'NONE', #26743, .T. ) ;
#30533=VECTOR ( 'NONE', #23945, 1000.000000000000000 ) ;
#30535=AXIS2_PLACEMENT_3D ( 'NONE', #9660, #21417, #6175 ) ;
#30542=CARTESIAN_POINT ( 'NONE',  ( -2.448748702180640446, -26.64985754041175525, 6.700000000000000178 ) ) ;
#30544=EDGE_CURVE ( 'NONE', #14576, #36371, #24407, .T. ) ;
#30555=CARTESIAN_POINT ( 'NONE',  ( -12.34874870218063947, -26.64985754041175525, 6.700000000000000178 ) ) ;
#30560=DIRECTION ( 'NONE',  ( 1.000000000000000000, 0.000000000000000000, -0.000000000000000000 ) ) ;
#30564=EDGE_LOOP ( 'NONE', ( #29458, #10190, #21339, #26163 ) ) ;
#30566=CARTESIAN_POINT ( 'NONE',  ( -1.078675913592196167, -24.55319635012989110, 6.700000000000000178 ) ) ;
#30570=ORIENTED_EDGE ( 'NONE', *, *, #35999, .F. ) ;
#30574=DIRECTION ( 'NONE',  ( -0.000000000000000000, -1.000000000000000000, -0.000000000000000000 ) ) ;
#30578=CARTESIAN_POINT ( 'NONE',  ( -16.44874870218064089, -25.49307895267003587, 6.800000000000000711 ) ) ;
#30580=FACE_OUTER_BOUND ( 'NONE', #18449, .T. ) ;
#30582=EDGE_LOOP ( 'NONE', ( #14583, #12548, #32528, #3819 ) ) ;
#30589=VECTOR ( 'NONE', #12516, 1000.000000000000000 ) ;
#30592=LINE ( 'NONE', #26875, #25519 ) ;
#30619=CARTESIAN_POINT ( 'NONE',  ( -0.2487487021806331078, -26.64985754041175525, 6.700000000000000178 ) ) ;
#30629=VERTEX_POINT ( 'NONE', #18841 ) ;
#30630=FACE_OUTER_BOUND ( 'NONE', #15352, .T. ) ;
#30636=CARTESIAN_POINT ( 'NONE',  ( 3.021324086407803478, -26.64985754041175525, 6.700000000000000178 ) ) ;
#30640=CARTESIAN_POINT ( 'NONE',  ( -23.07867591359219617, -26.64985754041175525, 6.800000000000000711 ) ) ;
#30644=EDGE_LOOP ( 'NONE', ( #13202, #10571, #24248, #1343 ) ) ;
#30647=AXIS2_PLACEMENT_3D ( 'NONE', #26318, #29597, #19923 ) ;
#30654=CYLINDRICAL_SURFACE ( 'NONE', #387, 2.499999999999996891 ) ;
#30655=VECTOR ( 'NONE', #40386, 1000.000000000000000 ) ;
#30667=ORIENTED_EDGE ( 'NONE', *, *, #6059, .T. ) ;
#30674=ORIENTED_EDGE ( 'NONE', *, *, #33012, .T. ) ;
#30680=AXIS2_PLACEMENT_3D ( 'NONE', #20935, #5291, #18450 ) ;
#30682=VERTEX_POINT ( 'NONE', #34825 ) ;
#30688=CARTESIAN_POINT ( 'NONE',  ( -13.07867591359219617, -26.64985754041175525, 6.800000000000000711 ) ) ;
#30689=EDGE_LOOP ( 'NONE', ( #15008, #29611, #31542, #6100 ) ) ;
#30695=ORIENTED_EDGE ( 'NONE', *, *, #11932, .T. ) ;
#30697=EDGE_CURVE ( 'NONE', #1634, #7170, #25533, .T. ) ;
#30700=EDGE_LOOP ( 'NONE', ( #21024, #4441, #27340, #9140 ) ) ;
#30708=VECTOR ( 'NONE', #2410, 1000.000000000000000 ) ;
#30714=CARTESIAN_POINT ( 'NONE',  ( -8.448748702180639114, -25.49307895267003587, 6.700000000000000178 ) ) ;
#30731=CARTESIAN_POINT ( 'NONE',  ( -22.24874870218063450, -26.64985754041175525, 6.700000000000000178 ) ) ;
#30732=CARTESIAN_POINT ( 'NONE',  ( -13.07867591359219617, -26.64985754041175525, 6.700000000000000178 ) ) ;
#30744=AXIS2_PLACEMENT_3D ( 'NONE', #35448, #9485, #3553 ) ;
#30761=VERTEX_POINT ( 'NONE', #25333 ) ;
#30765=EDGE_CURVE ( 'NONE', #26557, #29356, #28621, .T. ) ;
#30767=DIRECTION ( 'NONE',  ( 1.000000000000000000, 0.000000000000000000, 0.000000000000000000 ) ) ;
#30771=LINE ( 'NONE', #6461, #37155 ) ;
#30774=CARTESIAN_POINT ( 'NONE',  ( -0.9786759135921931918, -26.64985754041175525, 6.700000000000000178 ) ) ;
#30776=ORIENTED_EDGE ( 'NONE', *, *, #19392, .F. ) ;
#30778=CIRCLE ( 'NONE', #5129, 0.1000000000000028644 ) ;
#30782=CARTESIAN_POINT ( 'NONE',  ( -12.97867591359219297, -24.55319635012989110, 6.700000000000000178 ) ) ;
#30783=LINE ( 'NONE', #21912, #33119 ) ;
#30787=EDGE_CURVE ( 'NONE', #22121, #29149, #40547, .T. ) ;
#30789=ORIENTED_EDGE ( 'NONE', *, *, #16135, .F. ) ;
#30795=LINE ( 'NONE', #21314, #23022 ) ;
#30798=EDGE_CURVE ( 'NONE', #31282, #19582, #33354, .T. ) ;
#30802=ORIENTED_EDGE ( 'NONE', *, *, #2836, .F. ) ;
#30814=FACE_OUTER_BOUND ( 'NONE', #35931, .T. ) ;
#30815=CARTESIAN_POINT ( 'NONE',  ( -2.448748702180640446, -26.64985754041175525, 6.800000000000000711 ) ) ;
#30820=ORIENTED_EDGE ( 'NONE', *, *, #29942, .T. ) ;
#30824=EDGE_CURVE ( 'NONE', #10798, #7879, #6186, .T. ) ;
#30830=CARTESIAN_POINT ( 'NONE',  ( -20.34874870218063947, -25.49307895267003587, 6.700000000000000178 ) ) ;
#30832=VECTOR ( 'NONE', #13693, 1000.000000000000000 ) ;
#30834=LINE ( 'NONE', #34346, #12922 ) ;
#30840=VERTEX_POINT ( 'NONE', #26142 ) ;
#30843=CARTESIAN_POINT ( 'NONE',  ( -26.34874870218063947, -25.49307895267003587, 6.800000000000000711 ) ) ;
#30844=ADVANCED_FACE ( 'NONE', ( #7193 ), #1435, .F. ) ;
#30848=CARTESIAN_POINT ( 'NONE',  ( -10.87867591359219155, -26.64985754041175525, 6.700000000000000178 ) ) ;
#30860=ORIENTED_EDGE ( 'NONE', *, *, #116, .T. ) ;
#30868=DIRECTION ( 'NONE',  ( 0.000000000000000000, 0.000000000000000000, 1.000000000000000000 ) ) ;
#30873=AXIS2_PLACEMENT_3D ( 'NONE', #11661, #11456, #20949 ) ;
#30874=VERTEX_POINT ( 'NONE', #22852 ) ;
#30880=ORIENTED_EDGE ( 'NONE', *, *, #23369, .F. ) ;
#30893=EDGE_CURVE ( 'NONE', #39054, #14484, #19532, .T. ) ;
#30896=DIRECTION ( 'NONE',  ( -1.000000000000000000, 0.000000000000000000, 0.000000000000000000 ) ) ;
#30905=EDGE_LOOP ( 'NONE', ( #9275, #1651, #16036, #11735 ) ) ;
#30906=VERTEX_POINT ( 'NONE', #38877 ) ;
#30918=EDGE_CURVE ( 'NONE', #8794, #6524, #20834, .T. ) ;
#30919=CARTESIAN_POINT ( 'NONE',  ( -28.34874870218063947, -26.64985754041175525, 6.700000000000000178 ) ) ;
#30927=DIRECTION ( 'NONE',  ( 1.000000000000000000, 0.000000000000000000, 0.000000000000000000 ) ) ;
#30936=LINE ( 'NONE', #5605, #4825 ) ;
#30946=DIRECTION ( 'NONE',  ( -0.000000000000000000, -0.000000000000000000, 1.000000000000000000 ) ) ;
#30947=FACE_OUTER_BOUND ( 'NONE', #40506, .T. ) ;
#30951=AXIS2_PLACEMENT_3D ( 'NONE', #22161, #12875, #31830 ) ;
#30958=LINE ( 'NONE', #18371, #423 ) ;
#30959=CARTESIAN_POINT ( 'NONE',  ( -12.97867591359219297, -26.64985754041175525, 6.700000000000000178 ) ) ;
#30965=DIRECTION ( 'NONE',  ( 0.000000000000000000, 0.000000000000000000, 1.000000000000000000 ) ) ;
#30968=CARTESIAN_POINT ( 'NONE',  ( -2.248748702180634940, -26.64985754041175525, 6.700000000000000178 ) ) ;
#30969=FACE_OUTER_BOUND ( 'NONE', #38707, .T. ) ;
#30971=PLANE ( 'NONE',  #23974 ) ;
#30973=EDGE_CURVE ( 'NONE', #38905, #37912, #4127, .T. ) ;
#30979=EDGE_LOOP ( 'NONE', ( #7506, #25660, #17229, #10937 ) ) ;
#30981=EDGE_CURVE ( 'NONE', #20273, #8305, #37941, .T. ) ;
#30982=EDGE_CURVE ( 'NONE', #35369, #24328, #14558, .T. ) ;
#30985=CARTESIAN_POINT ( 'NONE',  ( 3.121324086407806231, -24.55319635012989110, 6.700000000000000178 ) ) ;
#30996=EDGE_LOOP ( 'NONE', ( #6579, #17263, #40110, #28657 ) ) ;
#31017=CARTESIAN_POINT ( 'NONE',  ( -28.87867591359218977, -24.55319635012989110, 6.700000000000000178 ) ) ;
#31024=EDGE_CURVE ( 'NONE', #31748, #11338, #24451, .T. ) ;
#31036=CARTESIAN_POINT ( 'NONE',  ( 7.121324086407810228, -26.64985754041175525, 6.800000000000000711 ) ) ;
#31048=DIRECTION ( 'NONE',  ( 1.000000000000000000, 0.000000000000000000, 0.000000000000000000 ) ) ;
#31049=DIRECTION ( 'NONE',  ( -0.000000000000000000, -0.000000000000000000, -1.000000000000000000 ) ) ;
#31063=FACE_OUTER_BOUND ( 'NONE', #4393, .T. ) ;
#31064=EDGE_CURVE ( 'NONE', #36848, #28284, #26738, .T. ) ;
#31072=EDGE_CURVE ( 'NONE', #21009, #10798, #36203, .T. ) ;
#31081=CARTESIAN_POINT ( 'NONE',  ( -2.348748702180637693, -26.64985754041175525, 6.700000000000000178 ) ) ;
#31087=ORIENTED_EDGE ( 'NONE', *, *, #37145, .F. ) ;
#31090=EDGE_LOOP ( 'NONE', ( #33771, #3042, #38563, #37649 ) ) ;
#31101=ORIENTED_EDGE ( 'NONE', *, *, #13147, .F. ) ;
#31104=DIRECTION ( 'NONE',  ( -0.000000000000000000, -1.000000000000000000, -0.000000000000000000 ) ) ;
#31105=ORIENTED_EDGE ( 'NONE', *, *, #25251, .F. ) ;
#31112=DIRECTION ( 'NONE',  ( 0.000000000000000000, 1.000000000000000000, 0.000000000000000000 ) ) ;
#31121=ORIENTED_EDGE ( 'NONE', *, *, #23984, .T. ) ;
#31126=ORIENTED_EDGE ( 'NONE', *, *, #15565, .T. ) ;
#31133=ORIENTED_EDGE ( 'NONE', *, *, #38854, .F. ) ;
#31138=ORIENTED_EDGE ( 'NONE', *, *, #10830, .F. ) ;
#31147=ORIENTED_EDGE ( 'NONE', *, *, #4301, .F. ) ;
#31161=EDGE_LOOP ( 'NONE', ( #30296, #2787, #6815, #6596 ) ) ;
#31164=DIRECTION ( 'NONE',  ( -0.000000000000000000, -1.000000000000000000, -0.000000000000000000 ) ) ;
#31171=PLANE ( 'NONE',  #2325 ) ;
#31173=CARTESIAN_POINT ( 'NONE',  ( -30.24874870218063450, -25.49307895267003587, 6.700000000000000178 ) ) ;
#31175=EDGE_CURVE ( 'NONE', #37024, #22121, #22207, .T. ) ;
#31179=VECTOR ( 'NONE', #33516, 1000.000000000000000 ) ;
#31181=DIRECTION ( 'NONE',  ( 1.000000000000000000, 0.000000000000000000, 0.000000000000000000 ) ) ;
#31182=DIRECTION ( 'NONE',  ( 0.000000000000000000, 1.000000000000000000, 0.000000000000000000 ) ) ;
#31184=CARTESIAN_POINT ( 'NONE',  ( -15.07867591359219439, -26.64985754041175525, 6.800000000000000711 ) ) ;
#31185=CARTESIAN_POINT ( 'NONE',  ( -29.07867591359219617, -26.64985754041175525, 6.800000000000000711 ) ) ;
#31186=ORIENTED_EDGE ( 'NONE', *, *, #26330, .F. ) ;
#31188=DIRECTION ( 'NONE',  ( 1.000000000000000000, 0.000000000000000000, 0.000000000000000000 ) ) ;
#31190=AXIS2_PLACEMENT_3D ( 'NONE', #34403, #12124, #5766 ) ;
#31191=ORIENTED_EDGE ( 'NONE', *, *, #264, .F. ) ;
#31203=ORIENTED_EDGE ( 'NONE', *, *, #3448, .T. ) ;
#31208=VECTOR ( 'NONE', #9353, 1000.000000000000000 ) ;
#31212=CARTESIAN_POINT ( 'NONE',  ( 5.551251297819359110, -26.64985754041175525, 6.800000000000000711 ) ) ;
#31217=VECTOR ( 'NONE', #14830, 1000.000000000000000 ) ;
#31227=FACE_OUTER_BOUND ( 'NONE', #40318, .T. ) ;
#31230=ORIENTED_EDGE ( 'NONE', *, *, #8779, .F. ) ;
#31236=LINE ( 'NONE', #12275, #24173 ) ;
#31243=CIRCLE ( 'NONE', #13474, 0.1000000000000028644 ) ;
#31244=DIRECTION ( 'NONE',  ( -0.000000000000000000, -1.000000000000000000, -0.000000000000000000 ) ) ;
#31246=PLANE ( 'NONE',  #19067 ) ;
#31253=ADVANCED_FACE ( 'NONE', ( #15389 ), #34365, .T. ) ;
#31258=CARTESIAN_POINT ( 'NONE',  ( -54.01549048184568846, -30.38627270959228710, -4.152976064860135708 ) ) ;
#31265=DIRECTION ( 'NONE',  ( -0.000000000000000000, -0.000000000000000000, 1.000000000000000000 ) ) ;
#31269=AXIS2_PLACEMENT_3D ( 'NONE', #12094, #24671, #37223 ) ;
#31275=AXIS2_PLACEMENT_3D ( 'NONE', #34335, #6106, #18642 ) ;
#31277=ORIENTED_EDGE ( 'NONE', *, *, #24649, .T. ) ;
#31282=VERTEX_POINT ( 'NONE', #6749 ) ;
#31283=CARTESIAN_POINT ( 'NONE',  ( 1.651251297819358754, -26.64985754041175525, 6.700000000000000178 ) ) ;
#31285=ORIENTED_EDGE ( 'NONE', *, *, #14775, .F. ) ;
#31286=CARTESIAN_POINT ( 'NONE',  ( 6.921324086407803833, -26.64985754041175525, 6.800000000000000711 ) ) ;
#31290=ORIENTED_EDGE ( 'NONE', *, *, #34809, .T. ) ;
#31293=ORIENTED_EDGE ( 'NONE', *, *, #12675, .T. ) ;
#31297=EDGE_CURVE ( 'NONE', #36016, #10099, #8380, .T. ) ;
#31299=DIRECTION ( 'NONE',  ( 1.000000000000000000, 0.000000000000000000, 0.000000000000000000 ) ) ;
#31301=CARTESIAN_POINT ( 'NONE',  ( -18.87867591359219333, -26.64985754041175525, 6.700000000000000178 ) ) ;
#31310=CARTESIAN_POINT ( 'NONE',  ( -38.87867591359218977, -26.64985754041175525, 6.800000000000000711 ) ) ;
#31320=CARTESIAN_POINT ( 'NONE',  ( -20.44874870218064444, -25.49307895267003587, 6.700000000000000178 ) ) ;
#31322=DIRECTION ( 'NONE',  ( 1.000000000000000000, 0.000000000000000000, -0.000000000000000000 ) ) ;
#31323=VERTEX_POINT ( 'NONE', #11870 ) ;
#31324=ORIENTED_EDGE ( 'NONE', *, *, #30174, .T. ) ;
#31334=VECTOR ( 'NONE', #30075, 1000.000000000000000 ) ;
#31335=FACE_BOUND ( 'NONE', #19764, .T. ) ;
#31345=DIRECTION ( 'NONE',  ( -0.000000000000000000, -0.000000000000000000, 1.000000000000000000 ) ) ;
#31350=EDGE_CURVE ( 'NONE', #30840, #6772, #20955, .T. ) ;
#31352=LINE ( 'NONE', #31556, #27342 ) ;
#31353=ADVANCED_FACE ( 'NONE', ( #27129 ), #5512, .T. ) ;
#31369=LINE ( 'NONE', #12617, #20018 ) ;
#31377=VERTEX_POINT ( 'NONE', #24447 ) ;
#31380=VECTOR ( 'NONE', #12352, 1000.000000000000000 ) ;
#31388=ORIENTED_EDGE ( 'NONE', *, *, #31680, .T. ) ;
#31390=FACE_OUTER_BOUND ( 'NONE', #6614, .T. ) ;
#31391=DIRECTION ( 'NONE',  ( 1.000000000000000000, 0.000000000000000000, 0.000000000000000000 ) ) ;
#31405=CARTESIAN_POINT ( 'NONE',  ( -18.87867591359219333, -26.64985754041175525, 6.700000000000000178 ) ) ;
#31406=VERTEX_POINT ( 'NONE', #14760 ) ;
#31408=DIRECTION ( 'NONE',  ( -0.000000000000000000, -0.000000000000000000, 1.000000000000000000 ) ) ;
#31427=ORIENTED_EDGE ( 'NONE', *, *, #10369, .T. ) ;
#31431=CARTESIAN_POINT ( 'NONE',  ( -51.01549048184568846, -30.38627270959228710, 6.000000000000000000 ) ) ;
#31440=CARTESIAN_POINT ( 'NONE',  ( -38.24874870218063450, -25.49307895267003587, 6.700000000000000178 ) ) ;
#31451=EDGE_CURVE ( 'NONE', #38171, #2784, #24656, .T. ) ;
#31454=CARTESIAN_POINT ( 'NONE',  ( -41.07867591359219972, -26.64985754041175525, 6.700000000000000178 ) ) ;
#31457=CARTESIAN_POINT ( 'NONE',  ( -20.97867591359219475, -26.64985754041175525, 6.700000000000000178 ) ) ;
#31458=ORIENTED_EDGE ( 'NONE', *, *, #7328, .T. ) ;
#31460=CARTESIAN_POINT ( 'NONE',  ( -29.07867591359219617, -26.64985754041175525, 6.700000000000000178 ) ) ;
#31467=CARTESIAN_POINT ( 'NONE',  ( -42.83131703149249603, -27.06993018339339585, 6.800000000000000711 ) ) ;
#31470=ADVANCED_FACE ( 'NONE', ( #17642 ), #30222, .T. ) ;
#31471=CARTESIAN_POINT ( 'NONE',  ( -32.87867591359218977, -26.64985754041175525, 6.800000000000000711 ) ) ;
#31477=AXIS2_PLACEMENT_3D ( 'NONE', #23748, #10583, #23356 ) ;
#31481=CARTESIAN_POINT ( 'NONE',  ( -22.44874870218064089, -26.64985754041175525, 6.800000000000000711 ) ) ;
#31495=ORIENTED_EDGE ( 'NONE', *, *, #7264, .F. ) ;
#31498=EDGE_CURVE ( 'NONE', #1835, #33795, #28356, .T. ) ;
#31499=DIRECTION ( 'NONE',  ( 1.000000000000000000, 0.000000000000000000, 0.000000000000000000 ) ) ;
#31500=CARTESIAN_POINT ( 'NONE',  ( 1.551251297819356001, -26.64985754041175525, 6.800000000000000711 ) ) ;
#31501=LINE ( 'NONE', #28816, #30363 ) ;
#31506=DIRECTION ( 'NONE',  ( 0.000000000000000000, 0.000000000000000000, -1.000000000000000000 ) ) ;
#31518=CARTESIAN_POINT ( 'NONE',  ( -36.44874870218064444, -25.49307895267003587, 6.700000000000000178 ) ) ;
#31525=ORIENTED_EDGE ( 'NONE', *, *, #25026, .F. ) ;
#31533=ORIENTED_EDGE ( 'NONE', *, *, #30544, .T. ) ;
#31535=DIRECTION ( 'NONE',  ( 0.000000000000000000, 0.000000000000000000, 1.000000000000000000 ) ) ;
#31540=FACE_BOUND ( 'NONE', #3872, .T. ) ;
#31541=CARTESIAN_POINT ( 'NONE',  ( -26.24874870218063450, -26.64985754041175525, 6.800000000000000711 ) ) ;
#31542=ORIENTED_EDGE ( 'NONE', *, *, #35743, .F. ) ;
#31556=CARTESIAN_POINT ( 'NONE',  ( -39.07867591359219261, -26.64985754041175525, 6.700000000000000178 ) ) ;
#31568=LINE ( 'NONE', #3391, #30188 ) ;
#31577=DIRECTION ( 'NONE',  ( 1.000000000000000000, 0.000000000000000000, 0.000000000000000000 ) ) ;
#31579=EDGE_CURVE ( 'NONE', #7170, #14656, #6546, .T. ) ;
#31592=ORIENTED_EDGE ( 'NONE', *, *, #33802, .T. ) ;
#31595=CARTESIAN_POINT ( 'NONE',  ( -26.44874870218064089, -26.64985754041175525, 6.800000000000000711 ) ) ;
#31598=ORIENTED_EDGE ( 'NONE', *, *, #20853, .T. ) ;
#31604=AXIS2_PLACEMENT_3D ( 'NONE', #33801, #5179, #17710 ) ;
#31614=CARTESIAN_POINT ( 'NONE',  ( -34.34874870218063592, -25.49307895267003587, 6.700000000000000178 ) ) ;
#31622=AXIS2_PLACEMENT_3D ( 'NONE', #35880, #39342, #20012 ) ;
#31623=CYLINDRICAL_SURFACE ( 'NONE', #30951, 0.1000000000000028644 ) ;
#31631=ADVANCED_FACE ( 'NONE', ( #12295 ), #18888, .T. ) ;
#31640=LINE ( 'NONE', #21971, #14056 ) ;
#31643=LINE ( 'NONE', #3263, #32743 ) ;
#31647=EDGE_LOOP ( 'NONE', ( #32924, #19912, #860, #37863 ) ) ;
#31658=DIRECTION ( 'NONE',  ( -1.000000000000000000, 0.000000000000000000, 0.000000000000000000 ) ) ;
#31680=EDGE_CURVE ( 'NONE', #21394, #11548, #16588, .T. ) ;
#31688=CARTESIAN_POINT ( 'NONE',  ( -6.878675913592188884, -26.64985754041175525, 6.700000000000000178 ) ) ;
#31694=CYLINDRICAL_SURFACE ( 'NONE', #19475, 0.1000000000000028644 ) ;
#31702=CARTESIAN_POINT ( 'NONE',  ( -32.24874870218063450, -26.64985754041175525, 6.700000000000000178 ) ) ;
#31708=ORIENTED_EDGE ( 'NONE', *, *, #15249, .T. ) ;
#31711=LINE ( 'NONE', #18518, #38751 ) ;
#31712=DIRECTION ( 'NONE',  ( 0.000000000000000000, 0.000000000000000000, -1.000000000000000000 ) ) ;
#31715=EDGE_LOOP ( 'NONE', ( #3627, #28598, #2124, #15622 ) ) ;
#31725=CARTESIAN_POINT ( 'NONE',  ( -28.44874870218064444, -26.64985754041175525, 6.700000000000000178 ) ) ;
#31726=CARTESIAN_POINT ( 'NONE',  ( -23.07867591359219617, -26.64985754041175525, 6.700000000000000178 ) ) ;
#31728=EDGE_CURVE ( 'NONE', #26477, #40182, #29565, .T. ) ;
#31729=ORIENTED_EDGE ( 'NONE', *, *, #36326, .F. ) ;
#31733=CARTESIAN_POINT ( 'NONE',  ( -42.34874870218063592, -26.64985754041175525, 6.700000000000000178 ) ) ;
#31740=FACE_BOUND ( 'NONE', #14863, .T. ) ;
#31747=DIRECTION ( 'NONE',  ( 0.000000000000000000, 0.000000000000000000, 1.000000000000000000 ) ) ;
#31748=VERTEX_POINT ( 'NONE', #7140 ) ;
#31752=DIRECTION ( 'NONE',  ( 1.000000000000000000, 0.000000000000000000, 0.000000000000000000 ) ) ;
#31757=EDGE_LOOP ( 'NONE', ( #19922, #29674, #26856, #287 ) ) ;
#31758=CARTESIAN_POINT ( 'NONE',  ( -12.24874870218063627, -26.64985754041175525, 6.700000000000000178 ) ) ;
#31768=EDGE_CURVE ( 'NONE', #35369, #14571, #28792, .T. ) ;
#31774=CARTESIAN_POINT ( 'NONE',  ( -42.24874870218063450, -26.64985754041175525, 6.700000000000000178 ) ) ;
#31779=AXIS2_PLACEMENT_3D ( 'NONE', #21773, #18881, #34152 ) ;
#31783=ORIENTED_EDGE ( 'NONE', *, *, #37990, .T. ) ;
#31788=CARTESIAN_POINT ( 'NONE',  ( -26.87867591359219333, -26.64985754041175525, 6.800000000000000711 ) ) ;
#31795=PLANE ( 'NONE',  #29381 ) ;
#31807=EDGE_LOOP ( 'NONE', ( #37357, #9846, #6067, #39793 ) ) ;
#31813=CARTESIAN_POINT ( 'NONE',  ( -30.34874870218063947, -25.49307895267003587, 6.700000000000000178 ) ) ;
#31814=ORIENTED_EDGE ( 'NONE', *, *, #2356, .T. ) ;
#31819=CARTESIAN_POINT ( 'NONE',  ( -30.24874870218063450, -26.64985754041175525, 6.700000000000000178 ) ) ;
#31820=VERTEX_POINT ( 'NONE', #7893 ) ;
#31827=DIRECTION ( 'NONE',  ( 0.000000000000000000, 0.000000000000000000, 1.000000000000000000 ) ) ;
#31830=DIRECTION ( 'NONE',  ( 1.000000000000000000, 0.000000000000000000, 0.000000000000000000 ) ) ;
#31836=VECTOR ( 'NONE', #37081, 1000.000000000000000 ) ;
#31837=CARTESIAN_POINT ( 'NONE',  ( -0.2487487021806331078, -25.49307895267003587, 6.700000000000000178 ) ) ;
#31844=ORIENTED_EDGE ( 'NONE', *, *, #12933, .F. ) ;
#31853=AXIS2_PLACEMENT_3D ( 'NONE', #17422, #27729, #14971 ) ;
#31855=CARTESIAN_POINT ( 'NONE',  ( -14.34874870218063769, -26.64985754041175525, 6.700000000000000178 ) ) ;
#31859=EDGE_LOOP ( 'NONE', ( #21416, #13646, #4248, #221 ) ) ;
#31883=CARTESIAN_POINT ( 'NONE',  ( -26.97867591359219475, -26.64985754041175525, 6.700000000000000178 ) ) ;
#31900=ORIENTED_EDGE ( 'NONE', *, *, #22261, .F. ) ;
#31904=ORIENTED_EDGE ( 'NONE', *, *, #7349, .T. ) ;
#31905=EDGE_LOOP ( 'NONE', ( #38650, #31495, #9875, #806 ) ) ;
#31914=ORIENTED_EDGE ( 'NONE', *, *, #29741, .T. ) ;
#31915=VERTEX_POINT ( 'NONE', #8490 ) ;
#31933=CARTESIAN_POINT ( 'NONE',  ( -4.878675913592187108, -24.55319635012989110, 6.800000000000000711 ) ) ;
#31934=CARTESIAN_POINT ( 'NONE',  ( -2.448748702180640446, -26.64985754041175525, 6.700000000000000178 ) ) ;
#31937=DIRECTION ( 'NONE',  ( 1.000000000000000000, 0.000000000000000000, 0.000000000000000000 ) ) ;
#31938=ORIENTED_EDGE ( 'NONE', *, *, #21970, .T. ) ;
#31944=AXIS2_PLACEMENT_3D ( 'NONE', #21176, #23832, #40100 ) ;
#31945=VERTEX_POINT ( 'NONE', #36509 ) ;
#31951=FACE_BOUND ( 'NONE', #24534, .T. ) ;
#31955=VECTOR ( 'NONE', #12048, 1000.000000000000000 ) ;
#31959=CARTESIAN_POINT ( 'NONE',  ( -28.24874870218063805, -26.64985754041175525, 6.700000000000000178 ) ) ;
#31969=CARTESIAN_POINT ( 'NONE',  ( -4.348748702180639469, -26.64985754041175525, 6.700000000000000178 ) ) ;
#31970=DIRECTION ( 'NONE',  ( 0.000000000000000000, -1.000000000000000000, 0.000000000000000000 ) ) ;
#31974=LINE ( 'NONE', #477, #18962 ) ;
#31979=AXIS2_PLACEMENT_3D ( 'NONE', #27092, #33077, #39638 ) ;
#31989=AXIS2_PLACEMENT_3D ( 'NONE', #28673, #9515, #18570 ) ;
#31993=ORIENTED_EDGE ( 'NONE', *, *, #23183, .T. ) ;
#32001=EDGE_CURVE ( 'NONE', #23756, #11841, #32184, .T. ) ;
#32003=DIRECTION ( 'NONE',  ( -1.000000000000000000, 0.000000000000000000, 0.000000000000000000 ) ) ;
#32008=CARTESIAN_POINT ( 'NONE',  ( 5.021324086407805254, -24.55319635012989110, 6.800000000000000711 ) ) ;
#32011=ORIENTED_EDGE ( 'NONE', *, *, #31024, .F. ) ;
#32024=LINE ( 'NONE', #31405, #25944 ) ;
#32030=ORIENTED_EDGE ( 'NONE', *, *, #13387, .F. ) ;
#32038=DIRECTION ( 'NONE',  ( 0.000000000000000000, 0.000000000000000000, -1.000000000000000000 ) ) ;
#32040=DIRECTION ( 'NONE',  ( 0.000000000000000000, 1.000000000000000000, 0.000000000000000000 ) ) ;
#32049=EDGE_CURVE ( 'NONE', #4500, #21616, #16500, .T. ) ;
#32050=CIRCLE ( 'NONE', #484, 0.1000000000000028644 ) ;
#32053=ORIENTED_EDGE ( 'NONE', *, *, #12883, .T. ) ;
#32058=LINE ( 'NONE', #3863, #14139 ) ;
#32060=PLANE ( 'NONE',  #5690 ) ;
#32062=EDGE_LOOP ( 'NONE', ( #17412, #21579, #4907, #2465 ) ) ;
#32070=LINE ( 'NONE', #13111, #4485 ) ;
#32077=CIRCLE ( 'NONE', #1825, 0.1000000000000028644 ) ;
#32097=LINE ( 'NONE', #3901, #18095 ) ;
#32101=DIRECTION ( 'NONE',  ( -1.000000000000000000, 0.000000000000000000, 0.000000000000000000 ) ) ;
#32108=ORIENTED_EDGE ( 'NONE', *, *, #36271, .T. ) ;
#32110=PLANE ( 'NONE',  #5662 ) ;
#32121=CARTESIAN_POINT ( 'NONE',  ( -6.348748702180634140, -26.64985754041175525, 6.700000000000000178 ) ) ;
#32123=VECTOR ( 'NONE', #39008, 1000.000000000000000 ) ;
#32126=CARTESIAN_POINT ( 'NONE',  ( -4.248748702180636272, -25.49307895267003587, 6.800000000000000711 ) ) ;
#32139=EDGE_LOOP ( 'NONE', ( #18298, #1174, #12599, #21981 ) ) ;
#32142=VERTEX_POINT ( 'NONE', #2670 ) ;
#32147=CARTESIAN_POINT ( 'NONE',  ( -42.24874870218063450, -26.64985754041175525, 6.800000000000000711 ) ) ;
#32150=CARTESIAN_POINT ( 'NONE',  ( -12.97867591359219297, -26.64985754041175525, 6.700000000000000178 ) ) ;
#32153=ORIENTED_EDGE ( 'NONE', *, *, #13097, .F. ) ;
#32159=EDGE_CURVE ( 'NONE', #20726, #34939, #33179, .T. ) ;
#32160=ORIENTED_EDGE ( 'NONE', *, *, #15855, .T. ) ;
#32163=ORIENTED_EDGE ( 'NONE', *, *, #22057, .T. ) ;
#32164=FACE_BOUND ( 'NONE', #21051, .T. ) ;
#32169=ORIENTED_EDGE ( 'NONE', *, *, #35632, .T. ) ;
#32178=AXIS2_PLACEMENT_3D ( 'NONE', #19136, #30896, #28399 ) ;
#32184=LINE ( 'NONE', #16901, #14990 ) ;
#32185=CARTESIAN_POINT ( 'NONE',  ( -34.97867591359219830, -26.64985754041175525, 6.800000000000000711 ) ) ;
#32190=DIRECTION ( 'NONE',  ( 0.000000000000000000, 0.000000000000000000, 1.000000000000000000 ) ) ;
#32204=FACE_OUTER_BOUND ( 'NONE', #37819, .T. ) ;
#32214=ORIENTED_EDGE ( 'NONE', *, *, #12515, .T. ) ;
#32221=CARTESIAN_POINT ( 'NONE',  ( -4.978675913592189417, -26.64985754041175525, 6.700000000000000178 ) ) ;
#32231=CARTESIAN_POINT ( 'NONE',  ( -16.34874870218063592, -25.49307895267003587, 6.700000000000000178 ) ) ;
#32235=VERTEX_POINT ( 'NONE', #19513 ) ;
#32242=EDGE_CURVE ( 'NONE', #38497, #15627, #563, .T. ) ;
#32254=ORIENTED_EDGE ( 'NONE', *, *, #33048, .T. ) ;
#32257=DIRECTION ( 'NONE',  ( 1.000000000000000000, 0.000000000000000000, 0.000000000000000000 ) ) ;
#32262=CIRCLE ( 'NONE', #25017, 0.1000000000000028644 ) ;
#32267=ORIENTED_EDGE ( 'NONE', *, *, #17105, .F. ) ;
#32268=ADVANCED_FACE ( 'NONE', ( #25889 ), #34371, .F. ) ;
#32289=EDGE_CURVE ( 'NONE', #29356, #27310, #12921, .T. ) ;
#32296=LINE ( 'NONE', #17212, #13508 ) ;
#32303=ORIENTED_EDGE ( 'NONE', *, *, #3163, .F. ) ;
#32304=AXIS2_PLACEMENT_3D ( 'NONE', #32150, #28010, #40557 ) ;
#32306=ORIENTED_EDGE ( 'NONE', *, *, #16362, .T. ) ;
#32310=DIRECTION ( 'NONE',  ( 1.000000000000000000, -0.000000000000000000, 0.000000000000000000 ) ) ;
#32314=LINE ( 'NONE', #817, #34760 ) ;
#32315=AXIS2_PLACEMENT_3D ( 'NONE', #20718, #39243, #24426 ) ;
#32328=EDGE_CURVE ( 'NONE', #2177, #24757, #30495, .T. ) ;
#32330=ORIENTED_EDGE ( 'NONE', *, *, #36524, .F. ) ;
#32339=ADVANCED_FACE ( 'NONE', ( #7547 ), #10825, .F. ) ;
#32344=DIRECTION ( 'NONE',  ( 0.000000000000000000, 1.000000000000000000, 0.000000000000000000 ) ) ;
#32359=DIRECTION ( 'NONE',  ( 0.000000000000000000, 0.000000000000000000, 1.000000000000000000 ) ) ;
#32369=ORIENTED_EDGE ( 'NONE', *, *, #20263, .T. ) ;
#32370=CYLINDRICAL_SURFACE ( 'NONE', #24076, 0.1000000000000028644 ) ;
#32373=CARTESIAN_POINT ( 'NONE',  ( -53.21549048184568420, -30.38627270959228710, 6.000000000000000000 ) ) ;
#32383=ORIENTED_EDGE ( 'NONE', *, *, #3800, .T. ) ;
#32386=EDGE_CURVE ( 'NONE', #12201, #18006, #29770, .T. ) ;
#32407=VERTEX_POINT ( 'NONE', #6685 ) ;
#32410=DIRECTION ( 'NONE',  ( -0.000000000000000000, -0.000000000000000000, 1.000000000000000000 ) ) ;
#32422=VECTOR ( 'NONE', #22192, 1000.000000000000000 ) ;
#32424=DIRECTION ( 'NONE',  ( -0.000000000000000000, -0.000000000000000000, 1.000000000000000000 ) ) ;
#32427=EDGE_CURVE ( 'NONE', #3771, #16635, #16655, .T. ) ;
#32430=PLANE ( 'NONE',  #13038 ) ;
#32437=LINE ( 'NONE', #339, #3261 ) ;
#32439=ORIENTED_EDGE ( 'NONE', *, *, #26643, .T. ) ;
#32442=AXIS2_PLACEMENT_3D ( 'NONE', #40250, #28315, #24614 ) ;
#32447=ADVANCED_FACE ( 'NONE', ( #15736 ), #19233, .F. ) ;
#32454=CARTESIAN_POINT ( 'NONE',  ( -22.24874870218063450, -25.49307895267003587, 6.700000000000000178 ) ) ;
#32459=DIRECTION ( 'NONE',  ( 0.000000000000000000, 0.000000000000000000, -1.000000000000000000 ) ) ;
#32473=CARTESIAN_POINT ( 'NONE',  ( -12.97867591359219297, -24.55319635012989110, 6.800000000000000711 ) ) ;
#32475=DIRECTION ( 'NONE',  ( 0.000000000000000000, 0.000000000000000000, 1.000000000000000000 ) ) ;
#32476=PLANE ( 'NONE',  #4911 ) ;
#32478=CARTESIAN_POINT ( 'NONE',  ( -40.34874870218063592, -26.64985754041175525, 6.700000000000000178 ) ) ;
#32479=VECTOR ( 'NONE', #21563, 1000.000000000000000 ) ;
#32483=CARTESIAN_POINT ( 'NONE',  ( 4.921324086407802056, -24.55319635012989110, 6.700000000000000178 ) ) ;
#32484=ORIENTED_EDGE ( 'NONE', *, *, #23654, .T. ) ;
#32498=AXIS2_PLACEMENT_3D ( 'NONE', #26218, #38748, #20017 ) ;
#32499=VECTOR ( 'NONE', #37045, 1000.000000000000000 ) ;
#32511=CARTESIAN_POINT ( 'NONE',  ( -32.44874870218063734, -25.49307895267003587, 6.800000000000000711 ) ) ;
#32528=ORIENTED_EDGE ( 'NONE', *, *, #34855, .F. ) ;
#32532=VECTOR ( 'NONE', #22106, 1000.000000000000000 ) ;
#32543=ORIENTED_EDGE ( 'NONE', *, *, #20044, .T. ) ;
#32556=( LENGTH_UNIT ( ) NAMED_UNIT ( * ) SI_UNIT ( .MILLI., .METRE. ) );
#32565=EDGE_LOOP ( 'NONE', ( #28130, #17670, #9278, #19175 ) ) ;
#32572=ORIENTED_EDGE ( 'NONE', *, *, #39130, .T. ) ;
#32576=CARTESIAN_POINT ( 'NONE',  ( -16.97867591359219475, -24.55319635012989110, 6.700000000000000178 ) ) ;
#32577=LINE ( 'NONE', #32972, #6377 ) ;
#32592=EDGE_CURVE ( 'NONE', #31945, #25222, #16935, .T. ) ;
#32593=DIRECTION ( 'NONE',  ( 1.000000000000000000, 0.000000000000000000, 0.000000000000000000 ) ) ;
#32594=VECTOR ( 'NONE', #19081, 1000.000000000000000 ) ;
#32595=ORIENTED_EDGE ( 'NONE', *, *, #916, .T. ) ;
#32609=ORIENTED_EDGE ( 'NONE', *, *, #29943, .T. ) ;
#32611=ADVANCED_FACE ( 'NONE', ( #7878 ), #26231, .T. ) ;
#32612=CARTESIAN_POINT ( 'NONE',  ( -42.83131703149249603, -27.06993018339339585, 6.800000000000000711 ) ) ;
#32623=AXIS2_PLACEMENT_3D ( 'NONE', #23794, #11429, #7753 ) ;
#32624=DIRECTION ( 'NONE',  ( 0.000000000000000000, 1.000000000000000000, 0.000000000000000000 ) ) ;
#32625=AXIS2_PLACEMENT_3D ( 'NONE', #31081, #6161, #9030 ) ;
#32627=FACE_OUTER_BOUND ( 'NONE', #34944, .T. ) ;
#32630=ORIENTED_EDGE ( 'NONE', *, *, #28665, .F. ) ;
#32641=DIRECTION ( 'NONE',  ( 0.000000000000000000, 0.000000000000000000, -1.000000000000000000 ) ) ;
#32656=ORIENTED_EDGE ( 'NONE', *, *, #5391, .T. ) ;
#32658=CARTESIAN_POINT ( 'NONE',  ( -51.21549048184567710, -30.94667987854474234, 6.000000000000000000 ) ) ;
#32667=DIRECTION ( 'NONE',  ( 1.000000000000000000, -0.000000000000000000, 0.000000000000000000 ) ) ;
#32681=EDGE_CURVE ( 'NONE', #26319, #1142, #10752, .T. ) ;
#32686=FACE_OUTER_BOUND ( 'NONE', #19501, .T. ) ;
#32690=ADVANCED_FACE ( 'NONE', ( #11351 ), #23331, .F. ) ;
#32694=FACE_OUTER_BOUND ( 'NONE', #23667, .T. ) ;
#32698=FACE_OUTER_BOUND ( 'NONE', #20259, .T. ) ;
#32700=VERTEX_POINT ( 'NONE', #4602 ) ;
#32702=AXIS2_PLACEMENT_3D ( 'NONE', #29454, #16668, #38703 ) ;
#32703=VERTEX_POINT ( 'NONE', #29311 ) ;
#32704=ORIENTED_EDGE ( 'NONE', *, *, #4157, .F. ) ;
#32705=EDGE_CURVE ( 'NONE', #6115, #37067, #14689, .T. ) ;
#32713=VECTOR ( 'NONE', #30218, 1000.000000000000000 ) ;
#32718=CARTESIAN_POINT ( 'NONE',  ( -40.97867591359219119, -24.55319635012989110, 6.800000000000000711 ) ) ;
#32733=VECTOR ( 'NONE', #8384, 1000.000000000000000 ) ;
#32737=DIRECTION ( 'NONE',  ( 1.000000000000000000, 0.000000000000000000, 0.000000000000000000 ) ) ;
#32740=PRODUCT_DEFINITION_FORMATION_WITH_SPECIFIED_SOURCE ( 'ANY', '', #26257, .NOT_KNOWN. ) ;
#32743=VECTOR ( 'NONE', #3865, 1000.000000000000000 ) ;
#32746=LINE ( 'NONE', #7607, #25065 ) ;
#32748=EDGE_LOOP ( 'NONE', ( #11288, #16250, #19375, #2948 ) ) ;
#32758=VERTEX_POINT ( 'NONE', #8675 ) ;
#32760=CARTESIAN_POINT ( 'NONE',  ( -28.24874870218063805, -26.64985754041175525, 6.800000000000000711 ) ) ;
#32765=AXIS2_PLACEMENT_3D ( 'NONE', #18260, #11461, #27329 ) ;
#32770=CARTESIAN_POINT ( 'NONE',  ( -6.348748702180634140, -26.64985754041175525, 6.700000000000000178 ) ) ;
#32778=CARTESIAN_POINT ( 'NONE',  ( -16.44874870218064089, -26.64985754041175525, 6.800000000000000711 ) ) ;
#32785=EDGE_LOOP ( 'NONE', ( #7026, #1623, #16873, #29340 ) ) ;
#32789=CARTESIAN_POINT ( 'NONE',  ( -4.878675913592187108, -26.64985754041175525, 6.700000000000000178 ) ) ;
#32791=DIRECTION ( 'NONE',  ( 0.000000000000000000, 0.000000000000000000, 1.000000000000000000 ) ) ;
#32795=ORIENTED_EDGE ( 'NONE', *, *, #16135, .T. ) ;
#32801=ORIENTED_EDGE ( 'NONE', *, *, #39491, .T. ) ;
#32802=CARTESIAN_POINT ( 'NONE',  ( -14.34874870218063769, -26.64985754041175525, 6.700000000000000178 ) ) ;
#32804=CARTESIAN_POINT ( 'NONE',  ( -2.248748702180634940, -26.64985754041175525, 6.800000000000000711 ) ) ;
#32814=CARTESIAN_POINT ( 'NONE',  ( -18.34874870218063947, -26.64985754041175525, 6.700000000000000178 ) ) ;
#32815=ORIENTED_EDGE ( 'NONE', *, *, #9428, .F. ) ;
#32820=ORIENTED_EDGE ( 'NONE', *, *, #19440, .T. ) ;
#32823=LINE ( 'NONE', #21067, #24877 ) ;
#32826=ORIENTED_EDGE ( 'NONE', *, *, #21184, .F. ) ;
#32829=ADVANCED_FACE ( 'NONE', ( #15472 ), #33430, .F. ) ;
#32840=ADVANCED_FACE ( 'NONE', ( #30525 ), #2334, .T. ) ;
#32855=AXIS2_PLACEMENT_3D ( 'NONE', #4180, #19810, #38131 ) ;
#32856=LINE ( 'NONE', #32658, #35936 ) ;
#32857=VERTEX_POINT ( 'NONE', #31959 ) ;
#32862=DIRECTION ( 'NONE',  ( 0.000000000000000000, 0.000000000000000000, 1.000000000000000000 ) ) ;
#32863=CARTESIAN_POINT ( 'NONE',  ( 1.121324086407811338, -24.55319635012989110, 6.800000000000000711 ) ) ;
#32866=LINE ( 'NONE', #23976, #37996 ) ;
#32868=VERTEX_POINT ( 'NONE', #3761 ) ;
#32878=DIRECTION ( 'NONE',  ( 1.000000000000000000, 0.000000000000000000, 0.000000000000000000 ) ) ;
#32897=EDGE_LOOP ( 'NONE', ( #34691, #23556, #16617, #24639 ) ) ;
#32903=LINE ( 'NONE', #35602, #10203 ) ;
#32908=CIRCLE ( 'NONE', #15140, 0.1000000000000028644 ) ;
#32910=DIRECTION ( 'NONE',  ( 1.000000000000000000, 0.000000000000000000, 0.000000000000000000 ) ) ;
#32924=ORIENTED_EDGE ( 'NONE', *, *, #17073, .T. ) ;
#32925=PLANE ( 'NONE',  #31944 ) ;
#32926=ORIENTED_EDGE ( 'NONE', *, *, #12468, .F. ) ;
#32928=CARTESIAN_POINT ( 'NONE',  ( -41.07867591359219972, -26.64985754041175525, 6.700000000000000178 ) ) ;
#32935=ORIENTED_EDGE ( 'NONE', *, *, #7128, .T. ) ;
#32936=LINE ( 'NONE', #7405, #15816 ) ;
#32937=AXIS2_PLACEMENT_3D ( 'NONE', #14480, #35930, #36525 ) ;
#32940=ORIENTED_EDGE ( 'NONE', *, *, #4528, .F. ) ;
#32941=VERTEX_POINT ( 'NONE', #34444 ) ;
#32953=ADVANCED_FACE ( 'NONE', ( #3168 ), #9709, .F. ) ;
#32967=VECTOR ( 'NONE', #8690, 1000.000000000000000 ) ;
#32970=DIRECTION ( 'NONE',  ( 1.000000000000000000, 0.000000000000000000, 0.000000000000000000 ) ) ;
#32972=CARTESIAN_POINT ( 'NONE',  ( -11.07867591359219794, -26.64985754041175525, 6.700000000000000178 ) ) ;
#32976=DIRECTION ( 'NONE',  ( -1.000000000000000000, 0.000000000000000000, 0.000000000000000000 ) ) ;
#32982=EDGE_CURVE ( 'NONE', #39757, #31915, #38911, .T. ) ;
#32984=EDGE_CURVE ( 'NONE', #29208, #699, #20379, .T. ) ;
#32985=DIRECTION ( 'NONE',  ( 1.000000000000000000, 1.273455763949465563E-16, 0.000000000000000000 ) ) ;
#32988=CYLINDRICAL_SURFACE ( 'NONE', #40150, 0.1000000000000028644 ) ;
#32995=ORIENTED_EDGE ( 'NONE', *, *, #30893, .T. ) ;
#32996=LINE ( 'NONE', #14037, #6839 ) ;
#33006=AXIS2_PLACEMENT_3D ( 'NONE', #39674, #8168, #2450 ) ;
#33012=EDGE_CURVE ( 'NONE', #39035, #2944, #20575, .T. ) ;
#33016=ORIENTED_EDGE ( 'NONE', *, *, #14164, .F. ) ;
#33018=LINE ( 'NONE', #33220, #39177 ) ;
#33023=ORIENTED_EDGE ( 'NONE', *, *, #35267, .T. ) ;
#33026=DIRECTION ( 'NONE',  ( 1.000000000000000000, 0.000000000000000000, 0.000000000000000000 ) ) ;
#33027=FACE_OUTER_BOUND ( 'NONE', #16398, .T. ) ;
#33029=LINE ( 'NONE', #38374, #35188 ) ;
#33041=AXIS2_PLACEMENT_3D ( 'NONE', #36085, #17115, #29887 ) ;
#33048=EDGE_CURVE ( 'NONE', #37911, #20726, #3574, .T. ) ;
#33053=ORIENTED_EDGE ( 'NONE', *, *, #22059, .F. ) ;
#33055=VERTEX_POINT ( 'NONE', #7828 ) ;
#33059=AXIS2_PLACEMENT_3D ( 'NONE', #1569, #14101, #36150 ) ;
#33062=CARTESIAN_POINT ( 'NONE',  ( -6.248748702180631831, -26.64985754041175525, 6.700000000000000178 ) ) ;
#33065=DIRECTION ( 'NONE',  ( 1.000000000000000000, 0.000000000000000000, 0.000000000000000000 ) ) ;
#33076=CARTESIAN_POINT ( 'NONE',  ( -20.24874870218063805, -26.64985754041175525, 6.800000000000000711 ) ) ;
#33077=DIRECTION ( 'NONE',  ( 0.000000000000000000, 0.000000000000000000, 1.000000000000000000 ) ) ;
#33079=CARTESIAN_POINT ( 'NONE',  ( 3.021324086407803478, -26.64985754041175525, 6.800000000000000711 ) ) ;
#33081=DIRECTION ( 'NONE',  ( 0.000000000000000000, 1.000000000000000000, 0.000000000000000000 ) ) ;
#33086=DIRECTION ( 'NONE',  ( 0.000000000000000000, 0.000000000000000000, 1.000000000000000000 ) ) ;
#33095=CARTESIAN_POINT ( 'NONE',  ( -14.97867591359219119, -26.64985754041175525, 6.800000000000000711 ) ) ;
#33105=EDGE_LOOP ( 'NONE', ( #3930, #37482, #12557, #10695 ) ) ;
#33106=ADVANCED_FACE ( 'NONE', ( #29858 ), #10507, .F. ) ;
#33109=FACE_OUTER_BOUND ( 'NONE', #12218, .T. ) ;
#33111=FACE_OUTER_BOUND ( 'NONE', #32139, .T. ) ;
#33113=CARTESIAN_POINT ( 'NONE',  ( -16.44874870218064089, -26.64985754041175525, 6.700000000000000178 ) ) ;
#33114=CARTESIAN_POINT ( 'NONE',  ( 1.021324086407808585, -24.55319635012989110, 6.700000000000000178 ) ) ;
#33115=DIRECTION ( 'NONE',  ( -0.000000000000000000, -0.000000000000000000, 1.000000000000000000 ) ) ;
#33119=VECTOR ( 'NONE', #9541, 1000.000000000000000 ) ;
#33127=VERTEX_POINT ( 'NONE', #30475 ) ;
#33130=PLANE ( 'NONE',  #13157 ) ;
#33133=DIRECTION ( 'NONE',  ( 1.000000000000000000, 0.000000000000000000, 0.000000000000000000 ) ) ;
#33135=CARTESIAN_POINT ( 'NONE',  ( -12.24874870218063627, -26.64985754041175525, 6.700000000000000178 ) ) ;
#33136=VERTEX_POINT ( 'NONE', #30688 ) ;
#33146=DIRECTION ( 'NONE',  ( 0.000000000000000000, 1.000000000000000000, 0.000000000000000000 ) ) ;
#33148=ORIENTED_EDGE ( 'NONE', *, *, #10188, .T. ) ;
#33150=ORIENTED_EDGE ( 'NONE', *, *, #34163, .T. ) ;
#33152=AXIS2_PLACEMENT_3D ( 'NONE', #5453, #10994, #17574 ) ;
#33161=EDGE_CURVE ( 'NONE', #15928, #18006, #5356, .T. ) ;
#33162=ORIENTED_EDGE ( 'NONE', *, *, #7658, .T. ) ;
#33167=ORIENTED_EDGE ( 'NONE', *, *, #23470, .T. ) ;
#33179=LINE ( 'NONE', #1689, #12999 ) ;
#33180=CIRCLE ( 'NONE', #6879, 0.1000000000000028644 ) ;
#33182=CARTESIAN_POINT ( 'NONE',  ( -42.83131703149249603, -32.06993018339340296, 6.000000000000000000 ) ) ;
#33183=CARTESIAN_POINT ( 'NONE',  ( 5.121324086407808451, -26.64985754041175525, 6.700000000000000178 ) ) ;
#33188=LINE ( 'NONE', #39754, #29616 ) ;
#33191=CARTESIAN_POINT ( 'NONE',  ( -18.34874870218063947, -26.64985754041175525, 6.700000000000000178 ) ) ;
#33197=AXIS2_PLACEMENT_3D ( 'NONE', #40611, #27851, #37324 ) ;
#33204=AXIS2_PLACEMENT_3D ( 'NONE', #21496, #3196, #14887 ) ;
#33207=ORIENTED_EDGE ( 'NONE', *, *, #12820, .F. ) ;
#33214=ORIENTED_EDGE ( 'NONE', *, *, #2921, .F. ) ;
#33220=CARTESIAN_POINT ( 'NONE',  ( -29.07867591359219617, -26.64985754041175525, 6.700000000000000178 ) ) ;
#33227=VERTEX_POINT ( 'NONE', #27581 ) ;
#33232=CIRCLE ( 'NONE', #11507, 0.1000000000000028644 ) ;
#33234=AXIS2_PLACEMENT_3D ( 'NONE', #3664, #34955, #16190 ) ;
#33257=CARTESIAN_POINT ( 'NONE',  ( 5.551251297819359110, -26.64985754041175525, 6.700000000000000178 ) ) ;
#33258=PLANE ( 'NONE',  #12831 ) ;
#33263=EDGE_CURVE ( 'NONE', #9354, #9750, #33382, .T. ) ;
#33264=VERTEX_POINT ( 'NONE', #27372 ) ;
#33269=ORIENTED_EDGE ( 'NONE', *, *, #11848, .F. ) ;
#33270=VECTOR ( 'NONE', #9299, 1000.000000000000000 ) ;
#33276=ORIENTED_EDGE ( 'NONE', *, *, #20266, .F. ) ;
#33293=DIRECTION ( 'NONE',  ( 1.000000000000000000, 0.000000000000000000, 0.000000000000000000 ) ) ;
#33294=EDGE_LOOP ( 'NONE', ( #27866, #40331, #8532, #26187 ) ) ;
#33309=DIRECTION ( 'NONE',  ( -0.000000000000000000, -1.000000000000000000, -0.000000000000000000 ) ) ;
#33313=CARTESIAN_POINT ( 'NONE',  ( -30.44874870218064089, -26.64985754041175525, 6.700000000000000178 ) ) ;
#33319=CARTESIAN_POINT ( 'NONE',  ( -40.34874870218063592, -25.49307895267003587, 6.700000000000000178 ) ) ;
#33321=LINE ( 'NONE', #20328, #39362 ) ;
#33324=FACE_OUTER_BOUND ( 'NONE', #8452, .T. ) ;
#33325=CARTESIAN_POINT ( 'NONE',  ( -41.07867591359219972, -24.55319635012989110, 6.800000000000000711 ) ) ;
#33331=EDGE_LOOP ( 'NONE', ( #13187, #15918, #19790, #24138 ) ) ;
#33332=EDGE_CURVE ( 'NONE', #4500, #31748, #38382, .T. ) ;
#33335=EDGE_LOOP ( 'NONE', ( #6409, #247, #12778, #10874 ) ) ;
#33341=CARTESIAN_POINT ( 'NONE',  ( -42.83131703149249603, -29.56993018339339940, 6.000000000000000000 ) ) ;
#33350=DIRECTION ( 'NONE',  ( 1.000000000000000000, 0.000000000000000000, 0.000000000000000000 ) ) ;
#33351=ORIENTED_EDGE ( 'NONE', *, *, #407, .T. ) ;
#33354=CIRCLE ( 'NONE', #9679, 0.1000000000000028644 ) ;
#33355=ADVANCED_FACE ( 'NONE', ( #9244 ), #3321, .F. ) ;
#33361=AXIS2_PLACEMENT_3D ( 'NONE', #21348, #40268, #8563 ) ;
#33364=DIRECTION ( 'NONE',  ( -0.000000000000000000, -0.000000000000000000, 1.000000000000000000 ) ) ;
#33369=VERTEX_POINT ( 'NONE', #25113 ) ;
#33375=VERTEX_POINT ( 'NONE', #12954 ) ;
#33381=LINE ( 'NONE', #39314, #16295 ) ;
#33382=LINE ( 'NONE', #33580, #32499 ) ;
#33397=VECTOR ( 'NONE', #534, 1000.000000000000000 ) ;
#33398=VECTOR ( 'NONE', #16028, 1000.000000000000000 ) ;
#33400=VERTEX_POINT ( 'NONE', #34607 ) ;
#33402=CARTESIAN_POINT ( 'NONE',  ( -38.87867591359218977, -24.55319635012989110, 6.800000000000000711 ) ) ;
#33404=LINE ( 'NONE', #5177, #24666 ) ;
#33406=DIRECTION ( 'NONE',  ( 1.000000000000000000, 0.000000000000000000, 0.000000000000000000 ) ) ;
#33407=DIRECTION ( 'NONE',  ( -0.000000000000000000, -0.000000000000000000, 1.000000000000000000 ) ) ;
#33410=EDGE_CURVE ( 'NONE', #33969, #39661, #28397, .T. ) ;
#33417=VECTOR ( 'NONE', #11667, 1000.000000000000000 ) ;
#33423=DIRECTION ( 'NONE',  ( 0.000000000000000000, 1.000000000000000000, 0.000000000000000000 ) ) ;
#33424=CIRCLE ( 'NONE', #38647, 2.000000000000000000 ) ;
#33426=ORIENTED_EDGE ( 'NONE', *, *, #12329, .F. ) ;
#33430=PLANE ( 'NONE',  #35765 ) ;
#33434=CYLINDRICAL_SURFACE ( 'NONE', #28270, 0.1000000000000028644 ) ;
#33443=DIRECTION ( 'NONE',  ( -0.000000000000000000, -1.000000000000000000, -0.000000000000000000 ) ) ;
#33446=DIRECTION ( 'NONE',  ( 0.000000000000000000, 1.000000000000000000, 0.000000000000000000 ) ) ;
#33447=PLANE ( 'NONE',  #35824 ) ;
#33455=CARTESIAN_POINT ( 'NONE',  ( 3.751251297819363728, -26.64985754041175525, 6.800000000000000711 ) ) ;
#33460=CARTESIAN_POINT ( 'NONE',  ( -24.24874870218063450, -26.64985754041175525, 6.700000000000000178 ) ) ;
#33472=DIRECTION ( 'NONE',  ( 1.000000000000000000, 0.000000000000000000, 0.000000000000000000 ) ) ;
#33477=DIRECTION ( 'NONE',  ( 1.000000000000000000, 0.000000000000000000, 0.000000000000000000 ) ) ;
#33490=ORIENTED_EDGE ( 'NONE', *, *, #4301, .T. ) ;
#33492=ADVANCED_FACE ( 'NONE', ( #38456 ), #39263, .T. ) ;
#33495=VECTOR ( 'NONE', #23817, 1000.000000000000000 ) ;
#33497=CARTESIAN_POINT ( 'NONE',  ( -36.34874870218064302, -25.49307895267003587, 6.700000000000000178 ) ) ;
#33500=CARTESIAN_POINT ( 'NONE',  ( -34.87867591359218977, -26.64985754041175525, 6.700000000000000178 ) ) ;
#33506=VERTEX_POINT ( 'NONE', #32511 ) ;
#33509=AXIS2_PLACEMENT_3D ( 'NONE', #21891, #34469, #12613 ) ;
#33515=CYLINDRICAL_SURFACE ( 'NONE', #20196, 0.1000000000000028644 ) ;
#33516=DIRECTION ( 'NONE',  ( -0.000000000000000000, -0.000000000000000000, 1.000000000000000000 ) ) ;
#33520=DIRECTION ( 'NONE',  ( 0.000000000000000000, 0.000000000000000000, -1.000000000000000000 ) ) ;
#33522=ORIENTED_EDGE ( 'NONE', *, *, #27696, .T. ) ;
#33528=EDGE_LOOP ( 'NONE', ( #6754, #26878, #41, #34639 ) ) ;
#33534=EDGE_CURVE ( 'NONE', #826, #6003, #21159, .T. ) ;
#33537=ORIENTED_EDGE ( 'NONE', *, *, #5109, .T. ) ;
#33538=ADVANCED_FACE ( 'NONE', ( #33109 ), #4892, .F. ) ;
#33549=CIRCLE ( 'NONE', #8534, 0.1000000000000028644 ) ;
#33558=VERTEX_POINT ( 'NONE', #18254 ) ;
#33568=CARTESIAN_POINT ( 'NONE',  ( -34.24874870218063450, -26.64985754041175525, 6.800000000000000711 ) ) ;
#33573=DIRECTION ( 'NONE',  ( 0.000000000000000000, 0.000000000000000000, 1.000000000000000000 ) ) ;
#33574=ORIENTED_EDGE ( 'NONE', *, *, #11187, .T. ) ;
#33575=EDGE_CURVE ( 'NONE', #8273, #33127, #19357, .T. ) ;
#33579=AXIS2_PLACEMENT_3D ( 'NONE', #29039, #29442, #1255 ) ;
#33580=CARTESIAN_POINT ( 'NONE',  ( 3.551251297819357777, -26.64985754041175525, 6.700000000000000178 ) ) ;
#33588=ADVANCED_FACE ( 'NONE', ( #36391 ), #20946, .F. ) ;
#33590=LINE ( 'NONE', #30078, #10480 ) ;
#33592=CARTESIAN_POINT ( 'NONE',  ( -16.24874870218063450, -26.64985754041175525, 6.700000000000000178 ) ) ;
#33596=FACE_OUTER_BOUND ( 'NONE', #25674, .T. ) ;
#33597=CIRCLE ( 'NONE', #39460, 0.1000000000000028644 ) ;
#33604=CARTESIAN_POINT ( 'NONE',  ( -28.44874870218064444, -25.49307895267003587, 6.800000000000000711 ) ) ;
#33613=FACE_OUTER_BOUND ( 'NONE', #19071, .T. ) ;
#33616=FACE_OUTER_BOUND ( 'NONE', #4790, .T. ) ;
#33618=DIRECTION ( 'NONE',  ( -0.000000000000000000, -0.000000000000000000, 1.000000000000000000 ) ) ;
#33620=CARTESIAN_POINT ( 'NONE',  ( 5.121324086407808451, -26.64985754041175525, 6.800000000000000711 ) ) ;
#33622=ORIENTED_EDGE ( 'NONE', *, *, #11418, .T. ) ;
#33627=DIRECTION ( 'NONE',  ( 1.000000000000000000, -0.000000000000000000, 0.000000000000000000 ) ) ;
#33634=ADVANCED_FACE ( 'NONE', ( #14547 ), #38013, .F. ) ;
#33637=AXIS2_PLACEMENT_3D ( 'NONE', #30251, #33146, #5749 ) ;
#33638=ADVANCED_FACE ( 'NONE', ( #16196 ), #366, .F. ) ;
#33647=CARTESIAN_POINT ( 'NONE',  ( -4.978675913592189417, -24.55319635012989110, 6.700000000000000178 ) ) ;
#33650=DIRECTION ( 'NONE',  ( 0.000000000000000000, 0.000000000000000000, 1.000000000000000000 ) ) ;
#33659=CARTESIAN_POINT ( 'NONE',  ( 4.921324086407802056, -26.64985754041175525, 6.700000000000000178 ) ) ;
#33660=VERTEX_POINT ( 'NONE', #25272 ) ;
#33664=CARTESIAN_POINT ( 'NONE',  ( -24.24874870218063450, -25.49307895267003587, 6.700000000000000178 ) ) ;
#33674=DIRECTION ( 'NONE',  ( 0.000000000000000000, 0.000000000000000000, 1.000000000000000000 ) ) ;
#33676=ORIENTED_EDGE ( 'NONE', *, *, #24975, .F. ) ;
#33683=EDGE_CURVE ( 'NONE', #744, #26853, #34962, .T. ) ;
#33685=VERTEX_POINT ( 'NONE', #19085 ) ;
#33695=FACE_OUTER_BOUND ( 'NONE', #29414, .T. ) ;
#33699=CARTESIAN_POINT ( 'NONE',  ( -10.44874870218064089, -26.64985754041175525, 6.800000000000000711 ) ) ;
#33709=CYLINDRICAL_SURFACE ( 'NONE', #16232, 0.1000000000000028644 ) ;
#33721=AXIS2_PLACEMENT_3D ( 'NONE', #21050, #6216, #15265 ) ;
#33722=DIRECTION ( 'NONE',  ( 1.000000000000000000, 0.000000000000000000, 0.000000000000000000 ) ) ;
#33729=PLANE ( 'NONE',  #27728 ) ;
#33732=VERTEX_POINT ( 'NONE', #22992 ) ;
#33739=DIRECTION ( 'NONE',  ( 0.000000000000000000, 1.000000000000000000, 0.000000000000000000 ) ) ;
#33741=FACE_OUTER_BOUND ( 'NONE', #8878, .T. ) ;
#33744=EDGE_CURVE ( 'NONE', #19079, #10898, #972, .T. ) ;
#33750=ORIENTED_EDGE ( 'NONE', *, *, #15565, .F. ) ;
#33752=DIRECTION ( 'NONE',  ( 0.000000000000000000, 0.000000000000000000, 1.000000000000000000 ) ) ;
#33753=AXIS2_PLACEMENT_3D ( 'NONE', #8714, #6469, #12626 ) ;
#33756=CARTESIAN_POINT ( 'NONE',  ( 5.651251297819362307, -25.49307895267003587, 6.700000000000000178 ) ) ;
#33765=DIRECTION ( 'NONE',  ( -0.000000000000000000, -0.000000000000000000, -1.000000000000000000 ) ) ;
#33767=ADVANCED_FACE ( 'NONE', ( #13109 ), #25669, .F. ) ;
#33770=VECTOR ( 'NONE', #37420, 1000.000000000000000 ) ;
#33771=ORIENTED_EDGE ( 'NONE', *, *, #22982, .T. ) ;
#33787=PLANE ( 'NONE',  #19694 ) ;
#33788=ORIENTED_EDGE ( 'NONE', *, *, #5011, .T. ) ;
#33792=CARTESIAN_POINT ( 'NONE',  ( -0.9786759135921931918, -24.55319635012989110, 6.700000000000000178 ) ) ;
#33795=VERTEX_POINT ( 'NONE', #32863 ) ;
#33796=ADVANCED_FACE ( 'NONE', ( #16390 ), #20087, .F. ) ;
#33801=CARTESIAN_POINT ( 'NONE',  ( -24.97867591359219475, -26.64985754041175525, 6.800000000000000711 ) ) ;
#33802=EDGE_CURVE ( 'NONE', #1190, #40382, #13717, .T. ) ;
#33804=VECTOR ( 'NONE', #4685, 1000.000000000000000 ) ;
#33807=CIRCLE ( 'NONE', #16698, 0.1000000000000028644 ) ;
#33812=EDGE_CURVE ( 'NONE', #12703, #9079, #29163, .T. ) ;
#33814=ORIENTED_EDGE ( 'NONE', *, *, #22427, .T. ) ;
#33818=CARTESIAN_POINT ( 'NONE',  ( -18.44874870218064089, -26.64985754041175525, 6.800000000000000711 ) ) ;
#33821=DIRECTION ( 'NONE',  ( -0.000000000000000000, -0.000000000000000000, 1.000000000000000000 ) ) ;
#33829=DIRECTION ( 'NONE',  ( 1.000000000000000000, 0.000000000000000000, -0.000000000000000000 ) ) ;
#33830=ORIENTED_EDGE ( 'NONE', *, *, #36561, .T. ) ;
#33835=DIRECTION ( 'NONE',  ( 1.000000000000000000, 0.000000000000000000, 0.000000000000000000 ) ) ;
#33842=CARTESIAN_POINT ( 'NONE',  ( -0.2487487021806331078, -26.64985754041175525, 6.700000000000000178 ) ) ;
#33849=CARTESIAN_POINT ( 'NONE',  ( -32.97867591359219119, -24.55319635012989110, 6.700000000000000178 ) ) ;
#33855=DIRECTION ( 'NONE',  ( -0.000000000000000000, -0.000000000000000000, 1.000000000000000000 ) ) ;
#33857=LINE ( 'NONE', #15093, #23302 ) ;
#33858=DIRECTION ( 'NONE',  ( -0.000000000000000000, -0.000000000000000000, 1.000000000000000000 ) ) ;
#33861=FACE_OUTER_BOUND ( 'NONE', #9134, .T. ) ;
#33862=VECTOR ( 'NONE', #18783, 1000.000000000000000 ) ;
#33864=CARTESIAN_POINT ( 'NONE',  ( -32.24874870218063450, -26.64985754041175525, 6.700000000000000178 ) ) ;
#33871=ORIENTED_EDGE ( 'NONE', *, *, #11795, .F. ) ;
#33874=LINE ( 'NONE', #40418, #20634 ) ;
#33876=CARTESIAN_POINT ( 'NONE',  ( -32.87867591359218977, -26.64985754041175525, 6.800000000000000711 ) ) ;
#33883=DIRECTION ( 'NONE',  ( -0.000000000000000000, -1.000000000000000000, -0.000000000000000000 ) ) ;
#33886=LINE ( 'NONE', #30377, #13811 ) ;
#33893=CYLINDRICAL_SURFACE ( 'NONE', #9108, 2.500000000000002220 ) ;
#33897=CARTESIAN_POINT ( 'NONE',  ( -2.978675913592195190, -24.55319635012989110, 6.700000000000000178 ) ) ;
#33899=AXIS2_PLACEMENT_3D ( 'NONE', #14091, #13902, #8107 ) ;
#33904=DIRECTION ( 'NONE',  ( -0.000000000000000000, -0.000000000000000000, 1.000000000000000000 ) ) ;
#33917=CARTESIAN_POINT ( 'NONE',  ( -22.24874870218063450, -26.64985754041175525, 6.700000000000000178 ) ) ;
#33918=AXIS2_PLACEMENT_3D ( 'NONE', #19736, #32310, #4107 ) ;
#33920=ADVANCED_FACE ( 'NONE', ( #2185 ), #18003, .T. ) ;
#33923=CARTESIAN_POINT ( 'NONE',  ( -10.97867591359219475, -26.64985754041175525, 6.700000000000000178 ) ) ;
#33927=CIRCLE ( 'NONE', #20721, 0.1000000000000028644 ) ;
#33929=VERTEX_POINT ( 'NONE', #14505 ) ;
#33930=PLANE ( 'NONE',  #23437 ) ;
#33938=CARTESIAN_POINT ( 'NONE',  ( 2.921324086407800280, -24.55319635012989110, 6.700000000000000178 ) ) ;
#33943=EDGE_CURVE ( 'NONE', #25803, #6772, #11407, .T. ) ;
#33945=ORIENTED_EDGE ( 'NONE', *, *, #2148, .F. ) ;
#33949=VECTOR ( 'NONE', #33821, 1000.000000000000000 ) ;
#33954=LINE ( 'NONE', #37011, #27273 ) ;
#33956=CARTESIAN_POINT ( 'NONE',  ( -24.24874870218063450, -26.64985754041175525, 6.800000000000000711 ) ) ;
#33958=EDGE_CURVE ( 'NONE', #17250, #29646, #5670, .T. ) ;
#33967=ADVANCED_FACE ( 'NONE', ( #4847 ), #8533, .T. ) ;
#33969=VERTEX_POINT ( 'NONE', #7929 ) ;
#33974=CARTESIAN_POINT ( 'NONE',  ( -8.878675913592189772, -26.64985754041175525, 6.800000000000000711 ) ) ;
#33975=FACE_OUTER_BOUND ( 'NONE', #34949, .T. ) ;
#33987=ORIENTED_EDGE ( 'NONE', *, *, #5582, .F. ) ;
#33991=ORIENTED_EDGE ( 'NONE', *, *, #32681, .F. ) ;
#33995=ADVANCED_FACE ( 'NONE', ( #26679 ), #20479, .F. ) ;
#34001=ORIENTED_EDGE ( 'NONE', *, *, #21184, .T. ) ;
#34006=DIRECTION ( 'NONE',  ( 0.000000000000000000, -1.000000000000000000, 0.000000000000000000 ) ) ;
#34007=EDGE_CURVE ( 'NONE', #33558, #15366, #23973, .T. ) ;
#34011=CARTESIAN_POINT ( 'NONE',  ( -25.07867591359219617, -26.64985754041175525, 6.800000000000000711 ) ) ;
#34025=DIRECTION ( 'NONE',  ( 1.000000000000000000, 0.000000000000000000, 0.000000000000000000 ) ) ;
#34031=LINE ( 'NONE', #18342, #29903 ) ;
#34032=ORIENTED_EDGE ( 'NONE', *, *, #730, .T. ) ;
#34033=CARTESIAN_POINT ( 'NONE',  ( -44.23414840393349579, -30.38627270959228710, 6.800000000000000711 ) ) ;
#34041=ORIENTED_EDGE ( 'NONE', *, *, #33332, .F. ) ;
#34051=AXIS2_PLACEMENT_3D ( 'NONE', #38665, #35416, #29420 ) ;
#34059=DIRECTION ( 'NONE',  ( 1.000000000000000000, 0.000000000000000000, 0.000000000000000000 ) ) ;
#34065=CARTESIAN_POINT ( 'NONE',  ( -4.448748702180642667, -25.49307895267003587, 6.700000000000000178 ) ) ;
#34066=LINE ( 'NONE', #33455, #2586 ) ;
#34069=LINE ( 'NONE', #30968, #12388 ) ;
#34072=FACE_OUTER_BOUND ( 'NONE', #1870, .T. ) ;
#34075=ADVANCED_FACE ( 'NONE', ( #12240 ), #19603, .F. ) ;
#34079=ORIENTED_EDGE ( 'NONE', *, *, #24940, .T. ) ;
#34082=VECTOR ( 'NONE', #16466, 1000.000000000000000 ) ;
#34093=ORIENTED_EDGE ( 'NONE', *, *, #35409, .T. ) ;
#34101=VECTOR ( 'NONE', #4668, 1000.000000000000000 ) ;
#34109=EDGE_CURVE ( 'NONE', #4930, #38778, #5877, .T. ) ;
#34118=DIRECTION ( 'NONE',  ( -0.000000000000000000, -0.000000000000000000, 1.000000000000000000 ) ) ;
#34120=CARTESIAN_POINT ( 'NONE',  ( -6.448748702180637338, -26.64985754041175525, 6.700000000000000178 ) ) ;
#34133=CYLINDRICAL_SURFACE ( 'NONE', #4446, 0.1000000000000028644 ) ;
#34136=ORIENTED_EDGE ( 'NONE', *, *, #22706, .F. ) ;
#34142=PLANE ( 'NONE',  #29348 ) ;
#34144=ORIENTED_EDGE ( 'NONE', *, *, #10304, .T. ) ;
#34147=DIRECTION ( 'NONE',  ( 0.000000000000000000, 0.000000000000000000, -1.000000000000000000 ) ) ;
#34152=DIRECTION ( 'NONE',  ( 0.000000000000000000, 0.000000000000000000, 1.000000000000000000 ) ) ;
#34153=DIRECTION ( 'NONE',  ( -0.000000000000000000, -0.000000000000000000, 1.000000000000000000 ) ) ;
#34155=DIRECTION ( 'NONE',  ( -0.000000000000000000, -0.000000000000000000, 1.000000000000000000 ) ) ;
#34156=CARTESIAN_POINT ( 'NONE',  ( -4.448748702180642667, -26.64985754041175525, 6.700000000000000178 ) ) ;
#34163=EDGE_CURVE ( 'NONE', #23072, #33660, #39526, .T. ) ;
#34169=ORIENTED_EDGE ( 'NONE', *, *, #16447, .F. ) ;
#34174=LINE ( 'NONE', #18275, #14909 ) ;
#34175=FACE_OUTER_BOUND ( 'NONE', #14106, .T. ) ;
#34180=VECTOR ( 'NONE', #17289, 1000.000000000000000 ) ;
#34183=LINE ( 'NONE', #31481, #27032 ) ;
#34184=DIRECTION ( 'NONE',  ( 0.000000000000000000, 1.000000000000000000, 0.000000000000000000 ) ) ;
#34186=ORIENTED_EDGE ( 'NONE', *, *, #24600, .T. ) ;
#34193=ORIENTED_EDGE ( 'NONE', *, *, #2836, .T. ) ;
#34199=ORIENTED_EDGE ( 'NONE', *, *, #19594, .F. ) ;
#34200=FACE_OUTER_BOUND ( 'NONE', #54, .T. ) ;
#34202=CARTESIAN_POINT ( 'NONE',  ( 3.751251297819363728, -25.49307895267003587, 6.800000000000000711 ) ) ;
#34203=CARTESIAN_POINT ( 'NONE',  ( -41.07867591359219972, -26.64985754041175525, 6.700000000000000178 ) ) ;
#34205=VERTEX_POINT ( 'NONE', #7638 ) ;
#34209=CARTESIAN_POINT ( 'NONE',  ( -6.878675913592188884, -24.55319635012989110, 6.700000000000000178 ) ) ;
#34210=EDGE_CURVE ( 'NONE', #9655, #33400, #8026, .T. ) ;
#34215=ORIENTED_EDGE ( 'NONE', *, *, #22056, .F. ) ;
#34225=DIRECTION ( 'NONE',  ( 1.000000000000000000, 0.000000000000000000, 0.000000000000000000 ) ) ;
#34231=EDGE_LOOP ( 'NONE', ( #7979, #6027, #21839, #8473 ) ) ;
#34236=VECTOR ( 'NONE', #6094, 1000.000000000000000 ) ;
#34237=CARTESIAN_POINT ( 'NONE',  ( -20.87867591359218977, -26.64985754041175525, 6.700000000000000178 ) ) ;
#34239=DIRECTION ( 'NONE',  ( -1.000000000000000000, 0.000000000000000000, 0.000000000000000000 ) ) ;
#34241=VERTEX_POINT ( 'NONE', #20188 ) ;
#34244=ADVANCED_FACE ( 'NONE', ( #29270 ), #26981, .F. ) ;
#34256=AXIS2_PLACEMENT_3D ( 'NONE', #5181, #8450, #14833 ) ;
#34259=ADVANCED_FACE ( 'NONE', ( #4369 ), #32370, .F. ) ;
#34273=DIRECTION ( 'NONE',  ( -0.000000000000000000, -0.000000000000000000, 1.000000000000000000 ) ) ;
#34289=VECTOR ( 'NONE', #19961, 1000.000000000000000 ) ;
#34294=EDGE_CURVE ( 'NONE', #31377, #17770, #1108, .T. ) ;
#34298=VERTEX_POINT ( 'NONE', #26388 ) ;
#34299=EDGE_CURVE ( 'NONE', #5793, #17630, #2064, .T. ) ;
#34301=AXIS2_PLACEMENT_3D ( 'NONE', #7445, #19613, #20401 ) ;
#34302=ORIENTED_EDGE ( 'NONE', *, *, #18441, .T. ) ;
#34311=DIRECTION ( 'NONE',  ( 1.000000000000000000, 0.000000000000000000, 0.000000000000000000 ) ) ;
#34327=CIRCLE ( 'NONE', #15865, 0.1000000000000028644 ) ;
#34335=CARTESIAN_POINT ( 'NONE',  ( -26.97867591359219475, -24.55319635012989110, 6.700000000000000178 ) ) ;
#34345=ORIENTED_EDGE ( 'NONE', *, *, #37274, .T. ) ;
#34346=CARTESIAN_POINT ( 'NONE',  ( -35.07867591359219972, -26.64985754041175525, 6.700000000000000178 ) ) ;
#34347=VECTOR ( 'NONE', #10344, 1000.000000000000000 ) ;
#34350=DIRECTION ( 'NONE',  ( 1.000000000000000000, -0.000000000000000000, 0.000000000000000000 ) ) ;
#34352=CARTESIAN_POINT ( 'NONE',  ( -2.978675913592195190, -24.55319635012989110, 6.800000000000000711 ) ) ;
#34354=CARTESIAN_POINT ( 'NONE',  ( -22.24874870218063450, -26.64985754041175525, 6.800000000000000711 ) ) ;
#34356=DIRECTION ( 'NONE',  ( 0.000000000000000000, 0.000000000000000000, 1.000000000000000000 ) ) ;
#34362=CIRCLE ( 'NONE', #6065, 6.781342077912186461 ) ;
#34365=PLANE ( 'NONE',  #21534 ) ;
#34371=PLANE ( 'NONE',  #25529 ) ;
#34387=ADVANCED_FACE ( 'NONE', ( #40339 ), #27177, .F. ) ;
#34391=EDGE_CURVE ( 'NONE', #25044, #3598, #24292, .T. ) ;
#34396=CARTESIAN_POINT ( 'NONE',  ( -12.34874870218063947, -25.49307895267003587, 6.700000000000000178 ) ) ;
#34397=VERTEX_POINT ( 'NONE', #19345 ) ;
#34403=CARTESIAN_POINT ( 'NONE',  ( -38.34874870218063592, -26.64985754041175525, 6.700000000000000178 ) ) ;
#34412=VERTEX_POINT ( 'NONE', #15645 ) ;
#34413=DIRECTION ( 'NONE',  ( 1.000000000000000000, 0.000000000000000000, 0.000000000000000000 ) ) ;
#34417=ORIENTED_EDGE ( 'NONE', *, *, #3346, .F. ) ;
#34434=ADVANCED_FACE ( 'NONE', ( #38271 ), #21830, .F. ) ;
#34436=FACE_BOUND ( 'NONE', #31757, .T. ) ;
#34444=CARTESIAN_POINT ( 'NONE',  ( -38.24874870218063450, -26.64985754041175525, 6.800000000000000711 ) ) ;
#34445=VERTEX_POINT ( 'NONE', #9874 ) ;
#34452=PLANE ( 'NONE',  #23462 ) ;
#34455=AXIS2_PLACEMENT_3D ( 'NONE', #16165, #7500, #28729 ) ;
#34462=EDGE_CURVE ( 'NONE', #12705, #13485, #30018, .T. ) ;
#34463=CARTESIAN_POINT ( 'NONE',  ( 5.121324086407808451, -26.64985754041175525, 6.700000000000000178 ) ) ;
#34467=CYLINDRICAL_SURFACE ( 'NONE', #28766, 0.1000000000000028644 ) ;
#34469=DIRECTION ( 'NONE',  ( 0.000000000000000000, 0.000000000000000000, 1.000000000000000000 ) ) ;
#34472=CARTESIAN_POINT ( 'NONE',  ( -10.87867591359219155, -26.64985754041175525, 6.700000000000000178 ) ) ;
#34476=CARTESIAN_POINT ( 'NONE',  ( -42.24874870218063450, -25.49307895267003587, 6.700000000000000178 ) ) ;
#34478=CARTESIAN_POINT ( 'NONE',  ( -15.07867591359219439, -26.64985754041175525, 6.700000000000000178 ) ) ;
#34480=ORIENTED_EDGE ( 'NONE', *, *, #18388, .F. ) ;
#34495=DIRECTION ( 'NONE',  ( 1.000000000000000000, 0.000000000000000000, -0.000000000000000000 ) ) ;
#34503=EDGE_CURVE ( 'NONE', #1874, #18519, #9267, .T. ) ;
#34508=FACE_OUTER_BOUND ( 'NONE', #31161, .T. ) ;
#34509=ORIENTED_EDGE ( 'NONE', *, *, #36402, .F. ) ;
#34512=ORIENTED_EDGE ( 'NONE', *, *, #13258, .T. ) ;
#34521=DIRECTION ( 'NONE',  ( 1.000000000000000000, -0.000000000000000000, 0.000000000000000000 ) ) ;
#34531=ORIENTED_EDGE ( 'NONE', *, *, #23445, .F. ) ;
#34544=AXIS2_PLACEMENT_3D ( 'NONE', #36924, #30140, #24569 ) ;
#34546=AXIS2_PLACEMENT_3D ( 'NONE', #19709, #12918, #29180 ) ;
#34548=DIRECTION ( 'NONE',  ( 0.000000000000000000, 0.000000000000000000, 1.000000000000000000 ) ) ;
#34551=AXIS2_PLACEMENT_3D ( 'NONE', #333, #34521, #24615 ) ;
#34556=ORIENTED_EDGE ( 'NONE', *, *, #10029, .F. ) ;
#34558=VECTOR ( 'NONE', #24278, 1000.000000000000000 ) ;
#34565=ORIENTED_EDGE ( 'NONE', *, *, #8969, .F. ) ;
#34567=ORIENTED_EDGE ( 'NONE', *, *, #27726, .T. ) ;
#34569=EDGE_CURVE ( 'NONE', #6772, #38905, #5994, .T. ) ;
#34577=DIRECTION ( 'NONE',  ( 0.000000000000000000, 0.000000000000000000, -1.000000000000000000 ) ) ;
#34585=VECTOR ( 'NONE', #6941, 1000.000000000000000 ) ;
#34587=ORIENTED_EDGE ( 'NONE', *, *, #38462, .T. ) ;
#34596=ORIENTED_EDGE ( 'NONE', *, *, #35267, .F. ) ;
#34604=EDGE_CURVE ( 'NONE', #12996, #2693, #2783, .T. ) ;
#34605=AXIS2_PLACEMENT_3D ( 'NONE', #21999, #21377, #9411 ) ;
#34607=CARTESIAN_POINT ( 'NONE',  ( -30.24874870218063450, -25.49307895267003587, 6.800000000000000711 ) ) ;
#34610=PLANE ( 'NONE',  #19195 ) ;
#34615=EDGE_CURVE ( 'NONE', #33127, #39661, #15719, .T. ) ;
#34616=AXIS2_PLACEMENT_3D ( 'NONE', #4761, #32976, #17295 ) ;
#34618=ADVANCED_FACE ( 'NONE', ( #12624 ), #14892, .F. ) ;
#34620=ORIENTED_EDGE ( 'NONE', *, *, #17999, .F. ) ;
#34624=EDGE_LOOP ( 'NONE', ( #1923, #23897, #32267, #31203 ) ) ;
#34633=DIRECTION ( 'NONE',  ( 0.000000000000000000, 0.000000000000000000, 1.000000000000000000 ) ) ;
#34635=ORIENTED_EDGE ( 'NONE', *, *, #8302, .F. ) ;
#34639=ORIENTED_EDGE ( 'NONE', *, *, #9115, .T. ) ;
#34649=FACE_BOUND ( 'NONE', #39659, .T. ) ;
#34650=DIRECTION ( 'NONE',  ( 0.000000000000000000, 0.000000000000000000, 1.000000000000000000 ) ) ;
#34665=DIRECTION ( 'NONE',  ( -0.000000000000000000, -0.000000000000000000, 1.000000000000000000 ) ) ;
#34668=DIRECTION ( 'NONE',  ( -0.000000000000000000, -0.000000000000000000, 1.000000000000000000 ) ) ;
#34672=CIRCLE ( 'NONE', #40554, 2.000000000000000000 ) ;
#34675=VECTOR ( 'NONE', #12214, 1000.000000000000000 ) ;
#34676=EDGE_CURVE ( 'NONE', #650, #20163, #21291, .T. ) ;
#34691=ORIENTED_EDGE ( 'NONE', *, *, #3427, .T. ) ;
#34701=CARTESIAN_POINT ( 'NONE',  ( -40.44874870218063734, -26.64985754041175525, 6.800000000000000711 ) ) ;
#34702=ORIENTED_EDGE ( 'NONE', *, *, #19594, .T. ) ;
#34704=DIRECTION ( 'NONE',  ( 0.000000000000000000, 0.000000000000000000, -1.000000000000000000 ) ) ;
#34707=ORIENTED_EDGE ( 'NONE', *, *, #8115, .T. ) ;
#34715=CARTESIAN_POINT ( 'NONE',  ( -12.87867591359218977, -24.55319635012989110, 6.700000000000000178 ) ) ;
#34720=ORIENTED_EDGE ( 'NONE', *, *, #7128, .F. ) ;
#34731=DIRECTION ( 'NONE',  ( 1.000000000000000000, 0.000000000000000000, 0.000000000000000000 ) ) ;
#34733=DIRECTION ( 'NONE',  ( -0.000000000000000000, -0.000000000000000000, 1.000000000000000000 ) ) ;
#34734=CARTESIAN_POINT ( 'NONE',  ( 6.921324086407803833, -26.64985754041175525, 6.800000000000000711 ) ) ;
#34738=ORIENTED_EDGE ( 'NONE', *, *, #26724, .F. ) ;
#34753=ORIENTED_EDGE ( 'NONE', *, *, #5858, .F. ) ;
#34754=DIRECTION ( 'NONE',  ( 1.000000000000000000, 0.000000000000000000, 0.000000000000000000 ) ) ;
#34756=ORIENTED_EDGE ( 'NONE', *, *, #26276, .T. ) ;
#34759=PLANE ( 'NONE',  #9560 ) ;
#34760=VECTOR ( 'NONE', #4113, 1000.000000000000000 ) ;
#34763=ORIENTED_EDGE ( 'NONE', *, *, #40558, .T. ) ;
#34764=ADVANCED_FACE ( 'NONE', ( #13034 ), #1303, .F. ) ;
#34769=VERTEX_POINT ( 'NONE', #18281 ) ;
#34770=CARTESIAN_POINT ( 'NONE',  ( 3.121324086407806231, -24.55319635012989110, 6.700000000000000178 ) ) ;
#34781=CARTESIAN_POINT ( 'NONE',  ( -17.07867591359219617, -26.64985754041175525, 6.700000000000000178 ) ) ;
#34784=CARTESIAN_POINT ( 'NONE',  ( -32.87867591359218977, -26.64985754041175525, 6.700000000000000178 ) ) ;
#34787=CARTESIAN_POINT ( 'NONE',  ( 5.021324086407805254, -26.64985754041175525, 6.700000000000000178 ) ) ;
#34791=ORIENTED_EDGE ( 'NONE', *, *, #80, .T. ) ;
#34793=CARTESIAN_POINT ( 'NONE',  ( 5.551251297819359110, -26.64985754041175525, 6.800000000000000711 ) ) ;
#34795=ORIENTED_EDGE ( 'NONE', *, *, #39213, .F. ) ;
#34796=DIRECTION ( 'NONE',  ( -0.000000000000000000, -0.000000000000000000, 1.000000000000000000 ) ) ;
#34800=CIRCLE ( 'NONE', #38691, 0.1000000000000028644 ) ;
#34804=EDGE_CURVE ( 'NONE', #19388, #34205, #794, .T. ) ;
#34807=VERTEX_POINT ( 'NONE', #26506 ) ;
#34809=EDGE_CURVE ( 'NONE', #26136, #212, #38843, .T. ) ;
#34814=PLANE ( 'NONE',  #29704 ) ;
#34820=ORIENTED_EDGE ( 'NONE', *, *, #9733, .F. ) ;
#34821=ORIENTED_EDGE ( 'NONE', *, *, #22982, .F. ) ;
#34825=CARTESIAN_POINT ( 'NONE',  ( -28.44874870218064444, -26.64985754041175525, 6.800000000000000711 ) ) ;
#34835=EDGE_LOOP ( 'NONE', ( #26949, #3545, #32011, #22168 ) ) ;
#34836=LINE ( 'NONE', #31725, #39474 ) ;
#34848=EDGE_CURVE ( 'NONE', #25004, #33375, #32296, .T. ) ;
#34852=FACE_BOUND ( 'NONE', #36381, .T. ) ;
#34853=EDGE_LOOP ( 'NONE', ( #20373, #37967, #10500, #3136 ) ) ;
#34855=EDGE_CURVE ( 'NONE', #3598, #39064, #33927, .T. ) ;
#34858=AXIS2_PLACEMENT_3D ( 'NONE', #31855, #38613, #35160 ) ;
#34859=CARTESIAN_POINT ( 'NONE',  ( -24.44874870218064089, -26.64985754041175525, 6.700000000000000178 ) ) ;
#34860=ORIENTED_EDGE ( 'NONE', *, *, #20970, .F. ) ;
#34878=DIRECTION ( 'NONE',  ( 0.000000000000000000, 0.000000000000000000, -1.000000000000000000 ) ) ;
#34882=FACE_OUTER_BOUND ( 'NONE', #19925, .T. ) ;
#34886=CARTESIAN_POINT ( 'NONE',  ( -12.87867591359218977, -24.55319635012989110, 6.700000000000000178 ) ) ;
#34891=CIRCLE ( 'NONE', #17079, 0.1000000000000028644 ) ;
#34902=DIRECTION ( 'NONE',  ( -1.000000000000000000, 0.000000000000000000, 0.000000000000000000 ) ) ;
#34906=ADVANCED_FACE ( 'NONE', ( #10041 ), #6962, .F. ) ;
#34910=EDGE_CURVE ( 'NONE', #4144, #1810, #13537, .T. ) ;
#34918=CIRCLE ( 'NONE', #5284, 0.1000000000000028644 ) ;
#34924=LINE ( 'NONE', #9976, #12762 ) ;
#34932=DIRECTION ( 'NONE',  ( 0.000000000000000000, 0.000000000000000000, 1.000000000000000000 ) ) ;
#34934=VECTOR ( 'NONE', #36270, 1000.000000000000000 ) ;
#34939=VERTEX_POINT ( 'NONE', #7358 ) ;
#34944=EDGE_LOOP ( 'NONE', ( #23313, #14509, #14543, #34079 ) ) ;
#34949=EDGE_LOOP ( 'NONE', ( #18150, #5981, #12865, #30667, #6155, #16426, #9893, #22028 ) ) ;
#34950=CARTESIAN_POINT ( 'NONE',  ( -18.97867591359219475, -26.64985754041175525, 6.700000000000000178 ) ) ;
#34951=ORIENTED_EDGE ( 'NONE', *, *, #39024, .F. ) ;
#34952=ADVANCED_FACE ( 'NONE', ( #4286 ), #1211, .F. ) ;
#34955=DIRECTION ( 'NONE',  ( -0.000000000000000000, -0.000000000000000000, 1.000000000000000000 ) ) ;
#34960=CIRCLE ( 'NONE', #38209, 0.1000000000000028644 ) ;
#34962=LINE ( 'NONE', #34354, #32422 ) ;
#34967=ORIENTED_EDGE ( 'NONE', *, *, #3095, .F. ) ;
#34982=EDGE_CURVE ( 'NONE', #38489, #32700, #7557, .T. ) ;
#34995=ORIENTED_EDGE ( 'NONE', *, *, #14719, .T. ) ;
#35018=EDGE_CURVE ( 'NONE', #35446, #1672, #3698, .T. ) ;
#35032=ADVANCED_FACE ( 'NONE', ( #27101 ), #2427, .F. ) ;
#35050=FACE_BOUND ( 'NONE', #35293, .T. ) ;
#35051=DIRECTION ( 'NONE',  ( 1.000000000000000000, 0.000000000000000000, 0.000000000000000000 ) ) ;
#35057=VERTEX_POINT ( 'NONE', #23797 ) ;
#35064=EDGE_LOOP ( 'NONE', ( #36408, #27598, #27949, #14768 ) ) ;
#35068=DIRECTION ( 'NONE',  ( 0.000000000000000000, 0.000000000000000000, 1.000000000000000000 ) ) ;
#35076=ADVANCED_FACE ( 'NONE', ( #23998 ), #14729, .F. ) ;
#35080=EDGE_CURVE ( 'NONE', #3524, #2073, #21343, .T. ) ;
#35092=PLANE ( 'NONE',  #15280 ) ;
#35094=ORIENTED_EDGE ( 'NONE', *, *, #18430, .T. ) ;
#35105=ORIENTED_EDGE ( 'NONE', *, *, #38740, .T. ) ;
#35117=EDGE_LOOP ( 'NONE', ( #11393, #5648, #2267, #10292 ) ) ;
#35120=ORIENTED_EDGE ( 'NONE', *, *, #36349, .T. ) ;
#35122=ORIENTED_EDGE ( 'NONE', *, *, #36997, .F. ) ;
#35123=LINE ( 'NONE', #7294, #18337 ) ;
#35131=CARTESIAN_POINT ( 'NONE',  ( -2.878675913592191993, -26.64985754041175525, 6.700000000000000178 ) ) ;
#35132=EDGE_CURVE ( 'NONE', #36027, #21196, #15357, .T. ) ;
#35140=ORIENTED_EDGE ( 'NONE', *, *, #5633, .F. ) ;
#35146=VERTEX_POINT ( 'NONE', #37582 ) ;
#35150=LINE ( 'NONE', #25657, #28595 ) ;
#35152=CARTESIAN_POINT ( 'NONE',  ( -38.24874870218063450, -26.64985754041175525, 6.700000000000000178 ) ) ;
#35160=DIRECTION ( 'NONE',  ( 1.000000000000000000, 0.000000000000000000, 0.000000000000000000 ) ) ;
#35168=AXIS2_PLACEMENT_3D ( 'NONE', #30555, #36519, #11581 ) ;
#35180=VERTEX_POINT ( 'NONE', #28534 ) ;
#35181=EDGE_CURVE ( 'NONE', #29204, #3657, #15151, .T. ) ;
#35185=CARTESIAN_POINT ( 'NONE',  ( -4.448748702180642667, -25.49307895267003587, 6.800000000000000711 ) ) ;
#35188=VECTOR ( 'NONE', #13473, 1000.000000000000000 ) ;
#35194=CARTESIAN_POINT ( 'NONE',  ( 0.9213240864078056092, -26.64985754041175525, 6.800000000000000711 ) ) ;
#35195=AXIS2_PLACEMENT_3D ( 'NONE', #941, #25844, #32641 ) ;
#35197=EDGE_LOOP ( 'NONE', ( #31598, #10153, #17062, #31290 ) ) ;
#35198=FACE_OUTER_BOUND ( 'NONE', #39219, .T. ) ;
#35199=AXIS2_PLACEMENT_3D ( 'NONE', #11953, #40570, #21456 ) ;
#35212=LINE ( 'NONE', #13162, #138 ) ;
#35219=VECTOR ( 'NONE', #16464, 1000.000000000000000 ) ;
#35221=VECTOR ( 'NONE', #7177, 1000.000000000000000 ) ;
#35226=ORIENTED_EDGE ( 'NONE', *, *, #19678, .F. ) ;
#35227=LINE ( 'NONE', #6999, #14963 ) ;
#35234=DIRECTION ( 'NONE',  ( 1.000000000000000000, 0.000000000000000000, 0.000000000000000000 ) ) ;
#35235=CARTESIAN_POINT ( 'NONE',  ( -16.24874870218063450, -26.64985754041175525, 6.700000000000000178 ) ) ;
#35236=EDGE_LOOP ( 'NONE', ( #35105, #9083, #35510, #13862 ) ) ;
#35240=VERTEX_POINT ( 'NONE', #15775 ) ;
#35244=VECTOR ( 'NONE', #17808, 1000.000000000000000 ) ;
#35246=AXIS2_PLACEMENT_3D ( 'NONE', #24951, #37487, #11546 ) ;
#35247=CARTESIAN_POINT ( 'NONE',  ( -24.24874870218063450, -25.49307895267003587, 6.700000000000000178 ) ) ;
#35250=FACE_BOUND ( 'NONE', #16521, .T. ) ;
#35252=CARTESIAN_POINT ( 'NONE',  ( -36.44874870218064444, -26.64985754041175525, 6.700000000000000178 ) ) ;
#35260=CARTESIAN_POINT ( 'NONE',  ( -8.978675913592192970, -24.55319635012989110, 6.700000000000000178 ) ) ;
#35267=EDGE_CURVE ( 'NONE', #26162, #25891, #27709, .T. ) ;
#35269=CARTESIAN_POINT ( 'NONE',  ( -31.07867591359219617, -24.55319635012989110, 6.700000000000000178 ) ) ;
#35270=FACE_OUTER_BOUND ( 'NONE', #32785, .T. ) ;
#35277=DIRECTION ( 'NONE',  ( -0.000000000000000000, -0.000000000000000000, 1.000000000000000000 ) ) ;
#35286=CIRCLE ( 'NONE', #31989, 0.1000000000000028644 ) ;
#35287=PLANE ( 'NONE',  #1794 ) ;
#35290=CARTESIAN_POINT ( 'NONE',  ( -28.24874870218063805, -26.64985754041175525, 6.700000000000000178 ) ) ;
#35292=ADVANCED_FACE ( 'NONE', ( #31227 ), #12267, .F. ) ;
#35293=EDGE_LOOP ( 'NONE', ( #12833, #35685, #14535, #22729 ) ) ;
#35307=ORIENTED_EDGE ( 'NONE', *, *, #37080, .T. ) ;
#35312=EDGE_CURVE ( 'NONE', #36632, #14653, #40464, .T. ) ;
#35317=PRODUCT_DEFINITION ( 'UNKNOWN', '', #32740, #2437 ) ;
#35328=EDGE_LOOP ( 'NONE', ( #2226, #24007, #8406, #13855 ) ) ;
#35336=DIRECTION ( 'NONE',  ( 1.000000000000000000, 0.000000000000000000, 0.000000000000000000 ) ) ;
#35338=LINE ( 'NONE', #7108, #739 ) ;
#35344=VECTOR ( 'NONE', #22803, 1000.000000000000000 ) ;
#35354=ORIENTED_EDGE ( 'NONE', *, *, #1267, .F. ) ;
#35369=VERTEX_POINT ( 'NONE', #19474 ) ;
#35377=CARTESIAN_POINT ( 'NONE',  ( -31.07867591359219617, -24.55319635012989110, 6.800000000000000711 ) ) ;
#35380=DIRECTION ( 'NONE',  ( 0.000000000000000000, 0.000000000000000000, 1.000000000000000000 ) ) ;
#35383=ORIENTED_EDGE ( 'NONE', *, *, #12129, .T. ) ;
#35385=DIRECTION ( 'NONE',  ( -0.000000000000000000, -0.000000000000000000, 1.000000000000000000 ) ) ;
#35398=ORIENTED_EDGE ( 'NONE', *, *, #28785, .T. ) ;
#35399=CARTESIAN_POINT ( 'NONE',  ( -8.448748702180639114, -26.64985754041175525, 6.800000000000000711 ) ) ;
#35404=PLANE ( 'NONE',  #33918 ) ;
#35407=ORIENTED_EDGE ( 'NONE', *, *, #30798, .T. ) ;
#35409=EDGE_CURVE ( 'NONE', #40638, #24427, #21094, .T. ) ;
#35412=AXIS2_PLACEMENT_3D ( 'NONE', #24601, #27682, #5878 ) ;
#35416=DIRECTION ( 'NONE',  ( 0.000000000000000000, 0.000000000000000000, 1.000000000000000000 ) ) ;
#35432=DIRECTION ( 'NONE',  ( -0.000000000000000000, -0.000000000000000000, 1.000000000000000000 ) ) ;
#35438=AXIS2_PLACEMENT_3D ( 'NONE', #40609, #24777, #37322 ) ;
#35446=VERTEX_POINT ( 'NONE', #3477 ) ;
#35447=CARTESIAN_POINT ( 'NONE',  ( -16.87867591359218977, -24.55319635012989110, 6.800000000000000711 ) ) ;
#35448=CARTESIAN_POINT ( 'NONE',  ( 0.000000000000000000, 0.000000000000000000, 0.000000000000000000 ) ) ;
#35452=ORIENTED_EDGE ( 'NONE', *, *, #23889, .T. ) ;
#35461=DIRECTION ( 'NONE',  ( -0.000000000000000000, -0.000000000000000000, 1.000000000000000000 ) ) ;
#35464=DIRECTION ( 'NONE',  ( 0.000000000000000000, 1.000000000000000000, 0.000000000000000000 ) ) ;
#35472=FACE_OUTER_BOUND ( 'NONE', #25509, .T. ) ;
#35478=CARTESIAN_POINT ( 'NONE',  ( -39.07867591359219261, -26.64985754041175525, 6.700000000000000178 ) ) ;
#35482=EDGE_CURVE ( 'NONE', #24284, #21608, #22204, .T. ) ;
#35487=DIRECTION ( 'NONE',  ( 0.000000000000000000, 1.000000000000000000, 0.000000000000000000 ) ) ;
#35490=EDGE_CURVE ( 'NONE', #8717, #13364, #375, .T. ) ;
#35492=DIRECTION ( 'NONE',  ( -0.000000000000000000, -0.000000000000000000, 1.000000000000000000 ) ) ;
#35496=LINE ( 'NONE', #706, #12979 ) ;
#35499=ORIENTED_EDGE ( 'NONE', *, *, #17053, .F. ) ;
#35503=ADVANCED_FACE ( 'NONE', ( #10425 ), #13119, .T. ) ;
#35510=ORIENTED_EDGE ( 'NONE', *, *, #12641, .F. ) ;
#35512=DIRECTION ( 'NONE',  ( 0.000000000000000000, 0.000000000000000000, 1.000000000000000000 ) ) ;
#35514=PLANE ( 'NONE',  #24904 ) ;
#35523=LINE ( 'NONE', #1344, #17037 ) ;
#35530=FACE_OUTER_BOUND ( 'NONE', #15120, .T. ) ;
#35538=ORIENTED_EDGE ( 'NONE', *, *, #4539, .F. ) ;
#35542=AXIS2_PLACEMENT_3D ( 'NONE', #16168, #10185, #740 ) ;
#35543=FACE_OUTER_BOUND ( 'NONE', #24039, .T. ) ;
#35549=DIRECTION ( 'NONE',  ( 1.000000000000000000, -0.000000000000000000, 0.000000000000000000 ) ) ;
#35552=AXIS2_PLACEMENT_3D ( 'NONE', #36665, #8240, #24518 ) ;
#35566=VECTOR ( 'NONE', #16515, 1000.000000000000000 ) ;
#35567=EDGE_CURVE ( 'NONE', #32407, #14576, #11367, .T. ) ;
#35580=EDGE_CURVE ( 'NONE', #25319, #19232, #35763, .T. ) ;
#35581=DIRECTION ( 'NONE',  ( 0.000000000000000000, 0.000000000000000000, 1.000000000000000000 ) ) ;
#35587=CARTESIAN_POINT ( 'NONE',  ( 7.021324086407807030, -24.55319635012989110, 6.800000000000000711 ) ) ;
#35594=VECTOR ( 'NONE', #20555, 1000.000000000000000 ) ;
#35596=EDGE_LOOP ( 'NONE', ( #5753, #21062, #12123, #26483 ) ) ;
#35601=AXIS2_PLACEMENT_3D ( 'NONE', #7187, #23441, #38873 ) ;
#35602=CARTESIAN_POINT ( 'NONE',  ( -28.24874870218063805, -26.64985754041175525, 6.700000000000000178 ) ) ;
#35609=CARTESIAN_POINT ( 'NONE',  ( -8.248748702180632719, -25.49307895267003587, 6.700000000000000178 ) ) ;
#35622=DIRECTION ( 'NONE',  ( 0.000000000000000000, 0.000000000000000000, 1.000000000000000000 ) ) ;
#35623=ORIENTED_EDGE ( 'NONE', *, *, #17372, .T. ) ;
#35626=CARTESIAN_POINT ( 'NONE',  ( -6.248748702180631831, -25.49307895267003587, 6.700000000000000178 ) ) ;
#35628=DIRECTION ( 'NONE',  ( -0.000000000000000000, -0.000000000000000000, 1.000000000000000000 ) ) ;
#35632=EDGE_CURVE ( 'NONE', #32941, #39924, #8279, .T. ) ;
#35635=VECTOR ( 'NONE', #37646, 1000.000000000000000 ) ;
#35636=EDGE_CURVE ( 'NONE', #1269, #40280, #30958, .T. ) ;
#35638=ORIENTED_EDGE ( 'NONE', *, *, #1267, .T. ) ;
#35639=EDGE_LOOP ( 'NONE', ( #22329, #10135, #37742, #32595 ) ) ;
#35649=EDGE_LOOP ( 'NONE', ( #33148, #19630, #11751, #5159 ) ) ;
#35652=DIRECTION ( 'NONE',  ( 0.000000000000000000, 0.000000000000000000, 1.000000000000000000 ) ) ;
#35654=ORIENTED_EDGE ( 'NONE', *, *, #17343, .T. ) ;
#35666=DIRECTION ( 'NONE',  ( 1.000000000000000000, 0.000000000000000000, 0.000000000000000000 ) ) ;
#35672=CIRCLE ( 'NONE', #17876, 0.1000000000000028644 ) ;
#35677=PLANE ( 'NONE',  #6899 ) ;
#35679=DIRECTION ( 'NONE',  ( 1.000000000000000000, 0.000000000000000000, 0.000000000000000000 ) ) ;
#35685=ORIENTED_EDGE ( 'NONE', *, *, #9864, .F. ) ;
#35691=CARTESIAN_POINT ( 'NONE',  ( -16.44874870218064089, -26.64985754041175525, 6.700000000000000178 ) ) ;
#35698=ORIENTED_EDGE ( 'NONE', *, *, #17592, .T. ) ;
#35709=ORIENTED_EDGE ( 'NONE', *, *, #4092, .T. ) ;
#35715=ORIENTED_EDGE ( 'NONE', *, *, #29842, .T. ) ;
#35718=EDGE_CURVE ( 'NONE', #12332, #23121, #35286, .T. ) ;
#35722=CARTESIAN_POINT ( 'NONE',  ( -13.07867591359219617, -26.64985754041175525, 6.700000000000000178 ) ) ;
#35724=DIRECTION ( 'NONE',  ( 1.000000000000000000, 0.000000000000000000, 0.000000000000000000 ) ) ;
#35727=AXIS2_PLACEMENT_3D ( 'NONE', #11458, #33115, #20529 ) ;
#35742=PLANE ( 'NONE',  #39089 ) ;
#35743=EDGE_CURVE ( 'NONE', #34769, #38692, #40600, .T. ) ;
#35752=VERTEX_POINT ( 'NONE', #12809 ) ;
#35755=LINE ( 'NONE', #19887, #22245 ) ;
#35763=LINE ( 'NONE', #30336, #4329 ) ;
#35765=AXIS2_PLACEMENT_3D ( 'NONE', #30319, #33627, #2128 ) ;
#35777=EDGE_CURVE ( 'NONE', #6472, #3076, #29076, .T. ) ;
#35779=DIRECTION ( 'NONE',  ( 1.000000000000000000, 0.000000000000000000, 0.000000000000000000 ) ) ;
#35786=VERTEX_POINT ( 'NONE', #13828 ) ;
#35788=DIRECTION ( 'NONE',  ( 1.000000000000000000, -0.000000000000000000, 0.000000000000000000 ) ) ;
#35791=AXIS2_PLACEMENT_3D ( 'NONE', #13435, #26012, #38542 ) ;
#35792=VECTOR ( 'NONE', #30422, 1000.000000000000000 ) ;
#35804=CIRCLE ( 'NONE', #30535, 0.1000000000000028644 ) ;
#35808=FACE_OUTER_BOUND ( 'NONE', #31905, .T. ) ;
#35823=CIRCLE ( 'NONE', #1001, 0.1000000000000028644 ) ;
#35824=AXIS2_PLACEMENT_3D ( 'NONE', #30959, #23737, #36308 ) ;
#35850=EDGE_CURVE ( 'NONE', #23072, #25044, #20197, .T. ) ;
#35852=ORIENTED_EDGE ( 'NONE', *, *, #32001, .F. ) ;
#35854=DIRECTION ( 'NONE',  ( 0.000000000000000000, 0.000000000000000000, 1.000000000000000000 ) ) ;
#35859=DIRECTION ( 'NONE',  ( 0.000000000000000000, 0.000000000000000000, 1.000000000000000000 ) ) ;
#35862=EDGE_CURVE ( 'NONE', #39757, #2177, #17492, .T. ) ;
#35869=CARTESIAN_POINT ( 'NONE',  ( -20.87867591359218977, -26.64985754041175525, 6.700000000000000178 ) ) ;
#35871=DIRECTION ( 'NONE',  ( 1.000000000000000000, 0.000000000000000000, 0.000000000000000000 ) ) ;
#35875=DIRECTION ( 'NONE',  ( -0.000000000000000000, -0.000000000000000000, 1.000000000000000000 ) ) ;
#35876=DIRECTION ( 'NONE',  ( -1.000000000000000000, 0.000000000000000000, 0.000000000000000000 ) ) ;
#35879=AXIS2_PLACEMENT_3D ( 'NONE', #33341, #2466, #5118 ) ;
#35880=CARTESIAN_POINT ( 'NONE',  ( -20.97867591359219475, -24.55319635012989110, 6.800000000000000711 ) ) ;
#35881=CIRCLE ( 'NONE', #40429, 0.1000000000000028644 ) ;
#35882=CARTESIAN_POINT ( 'NONE',  ( -14.34874870218063769, -25.49307895267003587, 6.700000000000000178 ) ) ;
#35890=DIRECTION ( 'NONE',  ( -0.000000000000000000, -0.000000000000000000, 1.000000000000000000 ) ) ;
#35901=ORIENTED_EDGE ( 'NONE', *, *, #865, .T. ) ;
#35908=VECTOR ( 'NONE', #34118, 1000.000000000000000 ) ;
#35919=VECTOR ( 'NONE', #24557, 1000.000000000000000 ) ;
#35920=DIRECTION ( 'NONE',  ( -0.000000000000000000, -0.000000000000000000, 1.000000000000000000 ) ) ;
#35922=CARTESIAN_POINT ( 'NONE',  ( -0.8786759135921904385, -26.64985754041175525, 6.700000000000000178 ) ) ;
#35929=DIRECTION ( 'NONE',  ( 1.000000000000000000, 0.000000000000000000, 0.000000000000000000 ) ) ;
#35930=DIRECTION ( 'NONE',  ( -0.000000000000000000, -0.000000000000000000, 1.000000000000000000 ) ) ;
#35931=EDGE_LOOP ( 'NONE', ( #12474, #20563, #9032, #23711 ) ) ;
#35935=DIRECTION ( 'NONE',  ( 1.000000000000000000, 0.000000000000000000, 0.000000000000000000 ) ) ;
#35936=VECTOR ( 'NONE', #29949, 1000.000000000000000 ) ;
#35941=DIRECTION ( 'NONE',  ( 0.000000000000000000, 0.000000000000000000, 1.000000000000000000 ) ) ;
#35950=CARTESIAN_POINT ( 'NONE',  ( -23.07867591359219617, -26.64985754041175525, 6.700000000000000178 ) ) ;
#35953=CARTESIAN_POINT ( 'NONE',  ( -16.87867591359218977, -26.64985754041175525, 6.700000000000000178 ) ) ;
#35955=CARTESIAN_POINT ( 'NONE',  ( -14.24874870218063450, -26.64985754041175525, 6.800000000000000711 ) ) ;
#35956=ORIENTED_EDGE ( 'NONE', *, *, #29522, .T. ) ;
#35970=CIRCLE ( 'NONE', #17534, 0.1000000000000028644 ) ;
#35983=VERTEX_POINT ( 'NONE', #5573 ) ;
#35985=CARTESIAN_POINT ( 'NONE',  ( -4.978675913592189417, -24.55319635012989110, 6.800000000000000711 ) ) ;
#35991=PLANE ( 'NONE',  #20081 ) ;
#35997=AXIS2_PLACEMENT_3D ( 'NONE', #31454, #31658, #15800 ) ;
#35999=EDGE_CURVE ( 'NONE', #3093, #15456, #39745, .T. ) ;
#36002=DIRECTION ( 'NONE',  ( -0.000000000000000000, -1.000000000000000000, -0.000000000000000000 ) ) ;
#36004=CARTESIAN_POINT ( 'NONE',  ( -12.34874870218063947, -26.64985754041175525, 6.700000000000000178 ) ) ;
#36010=ORIENTED_EDGE ( 'NONE', *, *, #2540, .T. ) ;
#36016=VERTEX_POINT ( 'NONE', #24091 ) ;
#36018=LINE ( 'NONE', #34120, #34236 ) ;
#36020=ADVANCED_FACE ( 'NONE', ( #23502 ), #7846, .F. ) ;
#36027=VERTEX_POINT ( 'NONE', #29873 ) ;
#36029=DIRECTION ( 'NONE',  ( 1.000000000000000000, 0.000000000000000000, -0.000000000000000000 ) ) ;
#36042=CARTESIAN_POINT ( 'NONE',  ( -12.34874870218063947, -26.64985754041175525, 6.700000000000000178 ) ) ;
#36044=ORIENTED_EDGE ( 'NONE', *, *, #37080, .F. ) ;
#36060=CARTESIAN_POINT ( 'NONE',  ( -26.87867591359219333, -24.55319635012989110, 6.700000000000000178 ) ) ;
#36071=EDGE_CURVE ( 'NONE', #35752, #12705, #10905, .T. ) ;
#36075=DIRECTION ( 'NONE',  ( 1.000000000000000000, 0.000000000000000000, -0.000000000000000000 ) ) ;
#36082=EDGE_CURVE ( 'NONE', #23016, #36632, #4213, .T. ) ;
#36085=CARTESIAN_POINT ( 'NONE',  ( -6.978675913592191193, -24.55319635012989110, 6.700000000000000178 ) ) ;
#36089=DIRECTION ( 'NONE',  ( -0.000000000000000000, -1.000000000000000000, -0.000000000000000000 ) ) ;
#36111=DIRECTION ( 'NONE',  ( 1.000000000000000000, 0.000000000000000000, 0.000000000000000000 ) ) ;
#36115=ORIENTED_EDGE ( 'NONE', *, *, #16177, .F. ) ;
#36119=CARTESIAN_POINT ( 'NONE',  ( -12.97867591359219297, -24.55319635012989110, 6.700000000000000178 ) ) ;
#36122=DIRECTION ( 'NONE',  ( 0.000000000000000000, 0.000000000000000000, 1.000000000000000000 ) ) ;
#36128=VECTOR ( 'NONE', #7974, 1000.000000000000000 ) ;
#36132=EDGE_CURVE ( 'NONE', #8785, #17194, #26437, .T. ) ;
#36141=CYLINDRICAL_SURFACE ( 'NONE', #39120, 0.1000000000000028644 ) ;
#36148=ORIENTED_EDGE ( 'NONE', *, *, #40018, .T. ) ;
#36150=DIRECTION ( 'NONE',  ( 1.000000000000000000, 0.000000000000000000, -0.000000000000000000 ) ) ;
#36156=DIRECTION ( 'NONE',  ( -0.000000000000000000, -0.000000000000000000, 1.000000000000000000 ) ) ;
#36159=DIRECTION ( 'NONE',  ( 1.000000000000000000, 0.000000000000000000, 0.000000000000000000 ) ) ;
#36162=CARTESIAN_POINT ( 'NONE',  ( 3.651251297819360531, -25.49307895267003587, 6.800000000000000711 ) ) ;
#36180=VERTEX_POINT ( 'NONE', #16343 ) ;
#36198=EDGE_LOOP ( 'NONE', ( #4362, #30570, #34967, #12227 ) ) ;
#36203=LINE ( 'NONE', #7982, #26149 ) ;
#36206=DIRECTION ( 'NONE',  ( 1.000000000000000000, -0.000000000000000000, 0.000000000000000000 ) ) ;
#36207=EDGE_LOOP ( 'NONE', ( #34193, #27097, #746, #15460 ) ) ;
#36213=DIRECTION ( 'NONE',  ( 0.000000000000000000, 0.000000000000000000, 1.000000000000000000 ) ) ;
#36219=LINE ( 'NONE', #10289, #34289 ) ;
#36221=EDGE_CURVE ( 'NONE', #26557, #30200, #29521, .T. ) ;
#36225=AXIS2_PLACEMENT_3D ( 'NONE', #19556, #38072, #31506 ) ;
#36233=CARTESIAN_POINT ( 'NONE',  ( -12.87867591359218977, -26.64985754041175525, 6.700000000000000178 ) ) ;
#36235=ORIENTED_EDGE ( 'NONE', *, *, #17399, .T. ) ;
#36244=DIRECTION ( 'NONE',  ( -0.000000000000000000, -0.000000000000000000, 1.000000000000000000 ) ) ;
#36253=FACE_OUTER_BOUND ( 'NONE', #35064, .T. ) ;
#36264=DIRECTION ( 'NONE',  ( 1.000000000000000000, 0.000000000000000000, 0.000000000000000000 ) ) ;
#36270=DIRECTION ( 'NONE',  ( 0.000000000000000000, 1.000000000000000000, 0.000000000000000000 ) ) ;
#36271=EDGE_CURVE ( 'NONE', #27940, #25461, #33018, .T. ) ;
#36278=ORIENTED_EDGE ( 'NONE', *, *, #22662, .F. ) ;
#36291=VERTEX_POINT ( 'NONE', #30125 ) ;
#36296=LINE ( 'NONE', #20632, #13691 ) ;
#36299=EDGE_LOOP ( 'NONE', ( #9813, #31904, #25514, #24231 ) ) ;
#36306=DIRECTION ( 'NONE',  ( -0.000000000000000000, -0.000000000000000000, 1.000000000000000000 ) ) ;
#36308=DIRECTION ( 'NONE',  ( 1.000000000000000000, 0.000000000000000000, -0.000000000000000000 ) ) ;
#36309=ORIENTED_EDGE ( 'NONE', *, *, #9779, .T. ) ;
#36323=CARTESIAN_POINT ( 'NONE',  ( 11.65737507970504439, -29.56993018339339940, 6.800000000000000711 ) ) ;
#36326=EDGE_CURVE ( 'NONE', #29204, #7215, #37218, .T. ) ;
#36329=AXIS2_PLACEMENT_3D ( 'NONE', #25811, #512, #10551 ) ;
#36339=DIRECTION ( 'NONE',  ( 1.000000000000000000, 0.000000000000000000, 0.000000000000000000 ) ) ;
#36342=ORIENTED_EDGE ( 'NONE', *, *, #34615, .F. ) ;
#36348=DIRECTION ( 'NONE',  ( 1.000000000000000000, 0.000000000000000000, 0.000000000000000000 ) ) ;
#36349=EDGE_CURVE ( 'NONE', #13245, #36422, #31352, .T. ) ;
#36356=EDGE_CURVE ( 'NONE', #20068, #9480, #21680, .T. ) ;
#36358=EDGE_CURVE ( 'NONE', #32142, #33506, #14839, .T. ) ;
#36364=DIRECTION ( 'NONE',  ( 1.000000000000000000, 0.000000000000000000, 0.000000000000000000 ) ) ;
#36371=VERTEX_POINT ( 'NONE', #9508 ) ;
#36380=DIRECTION ( 'NONE',  ( 1.000000000000000000, 0.000000000000000000, 0.000000000000000000 ) ) ;
#36381=EDGE_LOOP ( 'NONE', ( #11106, #34565, #25497, #27766 ) ) ;
#36388=ORIENTED_EDGE ( 'NONE', *, *, #7349, .F. ) ;
#36391=FACE_OUTER_BOUND ( 'NONE', #14899, .T. ) ;
#36393=CARTESIAN_POINT ( 'NONE',  ( -38.97867591359219119, -24.55319635012989110, 6.700000000000000178 ) ) ;
#36394=DIRECTION ( 'NONE',  ( 0.000000000000000000, 0.000000000000000000, -1.000000000000000000 ) ) ;
#36395=DIRECTION ( 'NONE',  ( 1.000000000000000000, 0.000000000000000000, 0.000000000000000000 ) ) ;
#36396=DIRECTION ( 'NONE',  ( -0.000000000000000000, -0.000000000000000000, 1.000000000000000000 ) ) ;
#36398=ORIENTED_EDGE ( 'NONE', *, *, #23652, .F. ) ;
#36402=EDGE_CURVE ( 'NONE', #9101, #1346, #12601, .T. ) ;
#36404=CARTESIAN_POINT ( 'NONE',  ( 11.65737507970504439, -23.60493063168009442, 6.800000000000000711 ) ) ;
#36408=ORIENTED_EDGE ( 'NONE', *, *, #20472, .T. ) ;
#36415=CARTESIAN_POINT ( 'NONE',  ( -0.3487487021806359722, -26.64985754041175525, 6.800000000000000711 ) ) ;
#36416=ORIENTED_EDGE ( 'NONE', *, *, #29943, .F. ) ;
#36422=VERTEX_POINT ( 'NONE', #37914 ) ;
#36424=DIRECTION ( 'NONE',  ( -0.000000000000000000, -0.000000000000000000, 1.000000000000000000 ) ) ;
#36432=ORIENTED_EDGE ( 'NONE', *, *, #34848, .F. ) ;
#36440=ADVANCED_FACE ( 'NONE', ( #5618 ), #18158, .F. ) ;
#36443=CARTESIAN_POINT ( 'NONE',  ( -36.24874870218063450, -25.49307895267003587, 6.700000000000000178 ) ) ;
#36450=FACE_OUTER_BOUND ( 'NONE', #38301, .T. ) ;
#36460=DIRECTION ( 'NONE',  ( 0.000000000000000000, 0.000000000000000000, 1.000000000000000000 ) ) ;
#36462=CARTESIAN_POINT ( 'NONE',  ( -42.44874870218064444, -26.64985754041175525, 6.700000000000000178 ) ) ;
#36464=CYLINDRICAL_SURFACE ( 'NONE', #35552, 0.1000000000000028644 ) ;
#36471=CARTESIAN_POINT ( 'NONE',  ( -22.24874870218063450, -25.49307895267003587, 6.800000000000000711 ) ) ;
#36472=EDGE_CURVE ( 'NONE', #169, #30629, #29986, .T. ) ;
#36476=VECTOR ( 'NONE', #6247, 1000.000000000000000 ) ;
#36485=DIRECTION ( 'NONE',  ( 1.000000000000000000, 0.000000000000000000, 0.000000000000000000 ) ) ;
#36487=VERTEX_POINT ( 'NONE', #4168 ) ;
#36509=CARTESIAN_POINT ( 'NONE',  ( -14.87867591359218977, -24.55319635012989110, 6.700000000000000178 ) ) ;
#36512=AXIS2_PLACEMENT_3D ( 'NONE', #23646, #36213, #33133 ) ;
#36514=VECTOR ( 'NONE', #1611, 1000.000000000000000 ) ;
#36515=FACE_OUTER_BOUND ( 'NONE', #40637, .T. ) ;
#36519=DIRECTION ( 'NONE',  ( 0.000000000000000000, 0.000000000000000000, 1.000000000000000000 ) ) ;
#36524=EDGE_CURVE ( 'NONE', #20068, #37067, #38720, .T. ) ;
#36525=DIRECTION ( 'NONE',  ( 1.000000000000000000, 0.000000000000000000, 0.000000000000000000 ) ) ;
#36526=EDGE_CURVE ( 'NONE', #9395, #25044, #8284, .T. ) ;
#36531=FACE_OUTER_BOUND ( 'NONE', #35596, .T. ) ;
#36534=EDGE_CURVE ( 'NONE', #38171, #4832, #40527, .T. ) ;
#36541=AXIS2_PLACEMENT_3D ( 'NONE', #2248, #14988, #36813 ) ;
#36546=AXIS2_PLACEMENT_3D ( 'NONE', #28043, #18994, #8891 ) ;
#36553=DIRECTION ( 'NONE',  ( 0.000000000000000000, 0.000000000000000000, 1.000000000000000000 ) ) ;
#36556=CARTESIAN_POINT ( 'NONE',  ( -28.34874870218063947, -26.64985754041175525, 6.700000000000000178 ) ) ;
#36561=EDGE_CURVE ( 'NONE', #1980, #30840, #876, .T. ) ;
#36563=DIRECTION ( 'NONE',  ( 1.000000000000000000, 0.000000000000000000, 0.000000000000000000 ) ) ;
#36573=ADVANCED_FACE ( 'NONE', ( #13615 ), #4370, .T. ) ;
#36574=CARTESIAN_POINT ( 'NONE',  ( -22.97867591359219119, -24.55319635012989110, 6.700000000000000178 ) ) ;
#36585=ADVANCED_FACE ( 'NONE', ( #25574 ), #17696, .F. ) ;
#36593=EDGE_LOOP ( 'NONE', ( #28891, #4940, #37474, #31592 ) ) ;
#36596=LINE ( 'NONE', #14153, #23895 ) ;
#36599=LINE ( 'NONE', #38869, #23843 ) ;
#36601=ORIENTED_EDGE ( 'NONE', *, *, #5633, .T. ) ;
#36609=CARTESIAN_POINT ( 'NONE',  ( -19.07867591359219972, -26.64985754041175525, 6.700000000000000178 ) ) ;
#36610=ORIENTED_EDGE ( 'NONE', *, *, #36082, .T. ) ;
#36632=VERTEX_POINT ( 'NONE', #36060 ) ;
#36635=LINE ( 'NONE', #11905, #23329 ) ;
#36653=LINE ( 'NONE', #5567, #34180 ) ;
#36654=CARTESIAN_POINT ( 'NONE',  ( -4.348748702180639469, -26.64985754041175525, 6.800000000000000711 ) ) ;
#36665=CARTESIAN_POINT ( 'NONE',  ( -40.97867591359219119, -24.55319635012989110, 6.700000000000000178 ) ) ;
#36675=ORIENTED_EDGE ( 'NONE', *, *, #29942, .F. ) ;
#36681=FACE_OUTER_BOUND ( 'NONE', #4308, .T. ) ;
#36682=ORIENTED_EDGE ( 'NONE', *, *, #12742, .F. ) ;
#36683=DIRECTION ( 'NONE',  ( 1.000000000000000000, 0.000000000000000000, 0.000000000000000000 ) ) ;
#36684=EDGE_CURVE ( 'NONE', #23873, #1854, #5694, .T. ) ;
#36686=CYLINDRICAL_SURFACE ( 'NONE', #192, 0.1000000000000028644 ) ;
#36687=ORIENTED_EDGE ( 'NONE', *, *, #33958, .F. ) ;
#36708=ORIENTED_EDGE ( 'NONE', *, *, #10039, .T. ) ;
#36718=LINE ( 'NONE', #8501, #38355 ) ;
#36724=LINE ( 'NONE', #27250, #24374 ) ;
#36736=DIRECTION ( 'NONE',  ( -0.000000000000000000, -0.000000000000000000, 1.000000000000000000 ) ) ;
#36738=DIRECTION ( 'NONE',  ( 0.000000000000000000, 0.000000000000000000, 1.000000000000000000 ) ) ;
#36739=ORIENTED_EDGE ( 'NONE', *, *, #39881, .F. ) ;
#36740=CYLINDRICAL_SURFACE ( 'NONE', #26654, 0.1000000000000028644 ) ;
#36746=EDGE_LOOP ( 'NONE', ( #20993, #9382, #25269, #40115 ) ) ;
#36747=AXIS2_PLACEMENT_3D ( 'NONE', #30919, #11943, #14428 ) ;
#36750=CARTESIAN_POINT ( 'NONE',  ( -20.87867591359218977, -26.64985754041175525, 6.700000000000000178 ) ) ;
#36766=DIRECTION ( 'NONE',  ( -0.000000000000000000, -0.000000000000000000, 1.000000000000000000 ) ) ;
#36775=CARTESIAN_POINT ( 'NONE',  ( -36.34874870218064302, -26.64985754041175525, 6.700000000000000178 ) ) ;
#36778=CARTESIAN_POINT ( 'NONE',  ( -8.978675913592192970, -26.64985754041175525, 6.800000000000000711 ) ) ;
#36780=CARTESIAN_POINT ( 'NONE',  ( -42.34874870218063592, -25.49307895267003587, 6.800000000000000711 ) ) ;
#36788=LINE ( 'NONE', #27113, #1670 ) ;
#36797=CARTESIAN_POINT ( 'NONE',  ( -5.078675913592192614, -26.64985754041175525, 6.700000000000000178 ) ) ;
#36798=DIRECTION ( 'NONE',  ( -0.000000000000000000, -0.000000000000000000, 1.000000000000000000 ) ) ;
#36804=AXIS2_PLACEMENT_3D ( 'NONE', #21435, #21843, #40349 ) ;
#36813=DIRECTION ( 'NONE',  ( 1.000000000000000000, 0.000000000000000000, -0.000000000000000000 ) ) ;
#36816=VECTOR ( 'NONE', #36766, 1000.000000000000000 ) ;
#36823=ADVANCED_FACE ( 'NONE', ( #33596 ), #27184, .F. ) ;
#36824=DIRECTION ( 'NONE',  ( 1.000000000000000000, 0.000000000000000000, 0.000000000000000000 ) ) ;
#36826=ORIENTED_EDGE ( 'NONE', *, *, #12641, .T. ) ;
#36832=VERTEX_POINT ( 'NONE', #21221 ) ;
#36833=AXIS2_PLACEMENT_3D ( 'NONE', #12092, #6758, #13531 ) ;
#36835=ORIENTED_EDGE ( 'NONE', *, *, #2596, .T. ) ;
#36840=CARTESIAN_POINT ( 'NONE',  ( -2.878675913592191993, -26.64985754041175525, 6.800000000000000711 ) ) ;
#36848=VERTEX_POINT ( 'NONE', #39949 ) ;
#36862=CARTESIAN_POINT ( 'NONE',  ( -40.44874870218063734, -26.64985754041175525, 6.700000000000000178 ) ) ;
#36864=VECTOR ( 'NONE', #16966, 1000.000000000000000 ) ;
#36865=EDGE_CURVE ( 'NONE', #24116, #26557, #4390, .T. ) ;
#36873=DIRECTION ( 'NONE',  ( -0.000000000000000000, -0.000000000000000000, 1.000000000000000000 ) ) ;
#36874=CARTESIAN_POINT ( 'NONE',  ( -28.87867591359218977, -24.55319635012989110, 6.800000000000000711 ) ) ;
#36877=ORIENTED_EDGE ( 'NONE', *, *, #31498, .T. ) ;
#36887=DIRECTION ( 'NONE',  ( 1.000000000000000000, 0.000000000000000000, 0.000000000000000000 ) ) ;
#36897=DIRECTION ( 'NONE',  ( 0.000000000000000000, 0.000000000000000000, 1.000000000000000000 ) ) ;
#36898=ORIENTED_EDGE ( 'NONE', *, *, #35312, .T. ) ;
#36902=CARTESIAN_POINT ( 'NONE',  ( -53.21549048184568420, -30.38627270959228710, -4.152976064860135708 ) ) ;
#36919=CARTESIAN_POINT ( 'NONE',  ( 11.65737507970504439, -23.60493063168009442, 6.000000000000000000 ) ) ;
#36924=CARTESIAN_POINT ( 'NONE',  ( -26.97867591359219475, -26.64985754041175525, 6.800000000000000711 ) ) ;
#36926=CARTESIAN_POINT ( 'NONE',  ( -30.24874870218063450, -25.49307895267003587, 6.700000000000000178 ) ) ;
#36931=DIRECTION ( 'NONE',  ( 0.000000000000000000, 0.000000000000000000, 1.000000000000000000 ) ) ;
#36932=ORIENTED_EDGE ( 'NONE', *, *, #11134, .F. ) ;
#36935=DIRECTION ( 'NONE',  ( 0.000000000000000000, 1.000000000000000000, 0.000000000000000000 ) ) ;
#36936=VECTOR ( 'NONE', #8427, 1000.000000000000000 ) ;
#36941=EDGE_CURVE ( 'NONE', #7215, #26593, #11931, .T. ) ;
#36945=EDGE_LOOP ( 'NONE', ( #13050, #37396, #20989, #11293 ) ) ;
#36955=CARTESIAN_POINT ( 'NONE',  ( -8.978675913592192970, -26.64985754041175525, 6.700000000000000178 ) ) ;
#36956=PLANE ( 'NONE',  #35412 ) ;
#36958=EDGE_LOOP ( 'NONE', ( #22471, #17482, #11633, #37188 ) ) ;
#36961=DIRECTION ( 'NONE',  ( -0.000000000000000000, -0.000000000000000000, 1.000000000000000000 ) ) ;
#36966=DIRECTION ( 'NONE',  ( 1.000000000000000000, 0.000000000000000000, 0.000000000000000000 ) ) ;
#36968=DIRECTION ( 'NONE',  ( 0.000000000000000000, 0.000000000000000000, 1.000000000000000000 ) ) ;
#36973=CARTESIAN_POINT ( 'NONE',  ( -6.248748702180631831, -26.64985754041175525, 6.800000000000000711 ) ) ;
#36983=CARTESIAN_POINT ( 'NONE',  ( -37.07867591359219261, -24.55319635012989110, 6.800000000000000711 ) ) ;
#36988=ORIENTED_EDGE ( 'NONE', *, *, #2345, .F. ) ;
#36992=DIRECTION ( 'NONE',  ( -0.000000000000000000, -1.000000000000000000, -0.000000000000000000 ) ) ;
#36997=EDGE_CURVE ( 'NONE', #25969, #8273, #29375, .T. ) ;
#37001=DIRECTION ( 'NONE',  ( -0.000000000000000000, -0.000000000000000000, 1.000000000000000000 ) ) ;
#37004=ORIENTED_EDGE ( 'NONE', *, *, #877, .F. ) ;
#37011=CARTESIAN_POINT ( 'NONE',  ( -32.44874870218063734, -26.64985754041175525, 6.700000000000000178 ) ) ;
#37019=FACE_OUTER_BOUND ( 'NONE', #6139, .T. ) ;
#37021=CARTESIAN_POINT ( 'NONE',  ( -10.24874870218063450, -25.49307895267003587, 6.800000000000000711 ) ) ;
#37024=VERTEX_POINT ( 'NONE', #22807 ) ;
#37028=CARTESIAN_POINT ( 'NONE',  ( -40.34874870218063592, -26.64985754041175525, 6.700000000000000178 ) ) ;
#37033=VECTOR ( 'NONE', #24669, 1000.000000000000000 ) ;
#37034=ORIENTED_EDGE ( 'NONE', *, *, #31175, .F. ) ;
#37035=CARTESIAN_POINT ( 'NONE',  ( -52.01549048184568846, -30.38627270959228710, 6.800000000000000711 ) ) ;
#37038=EDGE_CURVE ( 'NONE', #10273, #26136, #15536, .T. ) ;
#37045=DIRECTION ( 'NONE',  ( -0.000000000000000000, -1.000000000000000000, -0.000000000000000000 ) ) ;
#37059=CARTESIAN_POINT ( 'NONE',  ( -53.21549048184568420, -30.38627270959228710, 4.000000000000000000 ) ) ;
#37062=VECTOR ( 'NONE', #9540, 1000.000000000000000 ) ;
#37067=VERTEX_POINT ( 'NONE', #35377 ) ;
#37068=CARTESIAN_POINT ( 'NONE',  ( -18.34874870218063947, -25.49307895267003587, 6.800000000000000711 ) ) ;
#37070=VECTOR ( 'NONE', #37588, 1000.000000000000000 ) ;
#37077=CARTESIAN_POINT ( 'NONE',  ( -24.34874870218063592, -26.64985754041175525, 6.700000000000000178 ) ) ;
#37078=ORIENTED_EDGE ( 'NONE', *, *, #34391, .T. ) ;
#37080=EDGE_CURVE ( 'NONE', #4406, #26593, #4271, .T. ) ;
#37081=DIRECTION ( 'NONE',  ( -0.000000000000000000, -0.000000000000000000, 1.000000000000000000 ) ) ;
#37083=DIRECTION ( 'NONE',  ( 1.000000000000000000, 0.000000000000000000, -0.000000000000000000 ) ) ;
#37085=VERTEX_POINT ( 'NONE', #7742 ) ;
#37086=CARTESIAN_POINT ( 'NONE',  ( 6.921324086407803833, -26.64985754041175525, 6.700000000000000178 ) ) ;
#37096=EDGE_LOOP ( 'NONE', ( #12456, #32926, #17385, #12978 ) ) ;
#37105=VERTEX_POINT ( 'NONE', #23196 ) ;
#37109=ORIENTED_EDGE ( 'NONE', *, *, #14915, .T. ) ;
#37115=CARTESIAN_POINT ( 'NONE',  ( -2.448748702180640446, -25.49307895267003587, 6.700000000000000178 ) ) ;
#37126=DIRECTION ( 'NONE',  ( 0.000000000000000000, 0.000000000000000000, 1.000000000000000000 ) ) ;
#37134=ORIENTED_EDGE ( 'NONE', *, *, #3654, .T. ) ;
#37142=CARTESIAN_POINT ( 'NONE',  ( -26.97867591359219475, -24.55319635012989110, 6.800000000000000711 ) ) ;
#37145=EDGE_CURVE ( 'NONE', #6781, #30761, #20290, .T. ) ;
#37147=ADVANCED_FACE ( 'NONE', ( #29177 ), #19900, .T. ) ;
#37148=ORIENTED_EDGE ( 'NONE', *, *, #24214, .T. ) ;
#37155=VECTOR ( 'NONE', #40012, 1000.000000000000000 ) ;
#37156=CARTESIAN_POINT ( 'NONE',  ( -42.83131703149249603, -29.56993018339339940, 6.800000000000000711 ) ) ;
#37161=CARTESIAN_POINT ( 'NONE',  ( -40.87867591359218977, -26.64985754041175525, 6.700000000000000178 ) ) ;
#37162=AXIS2_PLACEMENT_3D ( 'NONE', #8315, #35941, #11398 ) ;
#37169=CYLINDRICAL_SURFACE ( 'NONE', #29174, 0.1000000000000028644 ) ;
#37180=VECTOR ( 'NONE', #5395, 1000.000000000000000 ) ;
#37186=AXIS2_PLACEMENT_3D ( 'NONE', #5486, #33086, #39441 ) ;
#37188=ORIENTED_EDGE ( 'NONE', *, *, #17840, .T. ) ;
#37189=DIRECTION ( 'NONE',  ( -0.000000000000000000, -1.000000000000000000, -0.000000000000000000 ) ) ;
#37191=VERTEX_POINT ( 'NONE', #6946 ) ;
#37199=DIRECTION ( 'NONE',  ( 1.000000000000000000, 0.000000000000000000, 0.000000000000000000 ) ) ;
#37201=CARTESIAN_POINT ( 'NONE',  ( -41.07867591359219972, -26.64985754041175525, 6.800000000000000711 ) ) ;
#37203=DIRECTION ( 'NONE',  ( 1.000000000000000000, 0.000000000000000000, 0.000000000000000000 ) ) ;
#37205=ORIENTED_EDGE ( 'NONE', *, *, #18491, .T. ) ;
#37209=CARTESIAN_POINT ( 'NONE',  ( -40.44874870218063734, -26.64985754041175525, 6.800000000000000711 ) ) ;
#37214=ORIENTED_EDGE ( 'NONE', *, *, #27330, .F. ) ;
#37217=EDGE_CURVE ( 'NONE', #8986, #22388, #35970, .T. ) ;
#37218=CIRCLE ( 'NONE', #24735, 2.000000000000000000 ) ;
#37223=DIRECTION ( 'NONE',  ( 1.000000000000000000, 0.000000000000000000, 0.000000000000000000 ) ) ;
#37224=DIRECTION ( 'NONE',  ( -0.000000000000000000, -0.000000000000000000, 1.000000000000000000 ) ) ;
#37229=DIRECTION ( 'NONE',  ( -0.000000000000000000, -1.000000000000000000, -0.000000000000000000 ) ) ;
#37233=VERTEX_POINT ( 'NONE', #18014 ) ;
#37234=CYLINDRICAL_SURFACE ( 'NONE', #29951, 0.1000000000000028644 ) ;
#37239=EDGE_CURVE ( 'NONE', #11841, #13011, #13596, .T. ) ;
#37241=VECTOR ( 'NONE', #29840, 1000.000000000000000 ) ;
#37246=ORIENTED_EDGE ( 'NONE', *, *, #6289, .F. ) ;
#37250=VERTEX_POINT ( 'NONE', #11620 ) ;
#37251=LINE ( 'NONE', #18509, #21993 ) ;
#37253=DIRECTION ( 'NONE',  ( -0.000000000000000000, -0.000000000000000000, 1.000000000000000000 ) ) ;
#37257=ORIENTED_EDGE ( 'NONE', *, *, #19496, .T. ) ;
#37258=ADVANCED_FACE ( 'NONE', ( #23986 ), #40051, .T. ) ;
#37261=ORIENTED_EDGE ( 'NONE', *, *, #16374, .F. ) ;
#37266=ORIENTED_EDGE ( 'NONE', *, *, #5966, .F. ) ;
#37274=EDGE_CURVE ( 'NONE', #16705, #1634, #34174, .T. ) ;
#37289=FACE_OUTER_BOUND ( 'NONE', #8977, .T. ) ;
#37292=CARTESIAN_POINT ( 'NONE',  ( -32.97867591359219119, -26.64985754041175525, 6.700000000000000178 ) ) ;
#37293=ORIENTED_EDGE ( 'NONE', *, *, #35850, .T. ) ;
#37301=PLANE ( 'NONE',  #697 ) ;
#37314=DIRECTION ( 'NONE',  ( 0.000000000000000000, 0.000000000000000000, 1.000000000000000000 ) ) ;
#37322=DIRECTION ( 'NONE',  ( 1.000000000000000000, 0.000000000000000000, -0.000000000000000000 ) ) ;
#37324=DIRECTION ( 'NONE',  ( 1.000000000000000000, 0.000000000000000000, 0.000000000000000000 ) ) ;
#37329=DIRECTION ( 'NONE',  ( 0.000000000000000000, 0.000000000000000000, 1.000000000000000000 ) ) ;
#37334=ORIENTED_EDGE ( 'NONE', *, *, #29394, .F. ) ;
#37357=ORIENTED_EDGE ( 'NONE', *, *, #3300, .T. ) ;
#37368=DIRECTION ( 'NONE',  ( -0.000000000000000000, -1.000000000000000000, -0.000000000000000000 ) ) ;
#37371=CARTESIAN_POINT ( 'NONE',  ( 1.021324086407808585, -26.64985754041175525, 6.700000000000000178 ) ) ;
#37386=DIRECTION ( 'NONE',  ( 0.000000000000000000, 0.000000000000000000, -1.000000000000000000 ) ) ;
#37392=CIRCLE ( 'NONE', #24920, 0.1000000000000028644 ) ;
#37396=ORIENTED_EDGE ( 'NONE', *, *, #1104, .F. ) ;
#37403=CARTESIAN_POINT ( 'NONE',  ( -22.44874870218064089, -25.49307895267003587, 6.700000000000000178 ) ) ;
#37404=CARTESIAN_POINT ( 'NONE',  ( -37.07867591359219261, -24.55319635012989110, 6.700000000000000178 ) ) ;
#37418=AXIS2_PLACEMENT_3D ( 'NONE', #36119, #5425, #11376 ) ;
#37420=DIRECTION ( 'NONE',  ( -0.000000000000000000, -1.000000000000000000, -0.000000000000000000 ) ) ;
#37432=CARTESIAN_POINT ( 'NONE',  ( -8.978675913592192970, -24.55319635012989110, 6.800000000000000711 ) ) ;
#37434=DIRECTION ( 'NONE',  ( 1.000000000000000000, 0.000000000000000000, 0.000000000000000000 ) ) ;
#37450=CARTESIAN_POINT ( 'NONE',  ( -14.24874870218063450, -26.64985754041175525, 6.700000000000000178 ) ) ;
#37459=ORIENTED_EDGE ( 'NONE', *, *, #37504, .T. ) ;
#37463=ORIENTED_EDGE ( 'NONE', *, *, #793, .T. ) ;
#37466=DIRECTION ( 'NONE',  ( -0.000000000000000000, -1.000000000000000000, -0.000000000000000000 ) ) ;
#37472=VECTOR ( 'NONE', #32040, 1000.000000000000000 ) ;
#37474=ORIENTED_EDGE ( 'NONE', *, *, #16813, .F. ) ;
#37475=EDGE_LOOP ( 'NONE', ( #40388, #24876, #20448, #4828 ) ) ;
#37478=VERTEX_POINT ( 'NONE', #19516 ) ;
#37482=ORIENTED_EDGE ( 'NONE', *, *, #20394, .F. ) ;
#37487=DIRECTION ( 'NONE',  ( 1.000000000000000000, -0.000000000000000000, 0.000000000000000000 ) ) ;
#37488=CARTESIAN_POINT ( 'NONE',  ( -28.24874870218063805, -25.49307895267003587, 6.800000000000000711 ) ) ;
#37500=EDGE_CURVE ( 'NONE', #27940, #26477, #32050, .T. ) ;
#37503=EDGE_LOOP ( 'NONE', ( #13589, #32826, #39269, #27720 ) ) ;
#37504=EDGE_CURVE ( 'NONE', #33375, #18637, #40556, .T. ) ;
#37527=LINE ( 'NONE', #9321, #4916 ) ;
#37531=VERTEX_POINT ( 'NONE', #5434 ) ;
#37536=CARTESIAN_POINT ( 'NONE',  ( -32.87867591359218977, -26.64985754041175525, 6.700000000000000178 ) ) ;
#37542=EDGE_LOOP ( 'NONE', ( #292, #26362, #23388, #10050 ) ) ;
#37545=ADVANCED_FACE ( 'NONE', ( #32686 ), #7752, .T. ) ;
#37556=FACE_OUTER_BOUND ( 'NONE', #7673, .T. ) ;
#37559=EDGE_LOOP ( 'NONE', ( #36278, #12752, #4243, #35901, #35307, #33522, #28851, #23490 ) ) ;
#37574=VECTOR ( 'NONE', #14582, 1000.000000000000000 ) ;
#37582=CARTESIAN_POINT ( 'NONE',  ( -10.44874870218064089, -25.49307895267003587, 6.700000000000000178 ) ) ;
#37585=ORIENTED_EDGE ( 'NONE', *, *, #30765, .F. ) ;
#37587=EDGE_CURVE ( 'NONE', #38497, #24389, #13740, .T. ) ;
#37588=DIRECTION ( 'NONE',  ( -0.000000000000000000, -0.000000000000000000, 1.000000000000000000 ) ) ;
#37591=EDGE_CURVE ( 'NONE', #8738, #35146, #1135, .T. ) ;
#37592=EDGE_LOOP ( 'NONE', ( #12489, #33269, #26715, #21201 ) ) ;
#37610=DIRECTION ( 'NONE',  ( 1.000000000000000000, 0.000000000000000000, -0.000000000000000000 ) ) ;
#37614=CARTESIAN_POINT ( 'NONE',  ( -8.978675913592192970, -26.64985754041175525, 6.700000000000000178 ) ) ;
#37616=DIRECTION ( 'NONE',  ( -0.000000000000000000, -1.000000000000000000, -0.000000000000000000 ) ) ;
#37630=EDGE_LOOP ( 'NONE', ( #1364, #2894, #8614, #3531 ) ) ;
#37633=CARTESIAN_POINT ( 'NONE',  ( -36.97867591359219119, -26.64985754041175525, 6.700000000000000178 ) ) ;
#37643=EDGE_CURVE ( 'NONE', #14571, #25004, #18585, .T. ) ;
#37644=DIRECTION ( 'NONE',  ( 1.000000000000000000, 0.000000000000000000, 0.000000000000000000 ) ) ;
#37646=DIRECTION ( 'NONE',  ( -0.000000000000000000, -1.000000000000000000, -0.000000000000000000 ) ) ;
#37649=ORIENTED_EDGE ( 'NONE', *, *, #34604, .T. ) ;
#37652=VERTEX_POINT ( 'NONE', #31173 ) ;
#37666=DIRECTION ( 'NONE',  ( 0.000000000000000000, 0.000000000000000000, 1.000000000000000000 ) ) ;
#37667=LINE ( 'NONE', #29240, #34082 ) ;
#37676=ADVANCED_FACE ( 'NONE', ( #2991 ), #28268, .F. ) ;
#37683=FACE_BOUND ( 'NONE', #26870, .T. ) ;
#37685=ORIENTED_EDGE ( 'NONE', *, *, #4214, .F. ) ;
#37691=ORIENTED_EDGE ( 'NONE', *, *, #30982, .T. ) ;
#37694=DIRECTION ( 'NONE',  ( 1.000000000000000000, 0.000000000000000000, 0.000000000000000000 ) ) ;
#37698=ORIENTED_EDGE ( 'NONE', *, *, #31451, .T. ) ;
#37700=AXIS2_PLACEMENT_3D ( 'NONE', #32814, #32410, #16725 ) ;
#37703=CARTESIAN_POINT ( 'NONE',  ( 5.551251297819359110, -25.49307895267003587, 6.700000000000000178 ) ) ;
#37717=CARTESIAN_POINT ( 'NONE',  ( -18.97867591359219475, -26.64985754041175525, 6.700000000000000178 ) ) ;
#37720=EDGE_CURVE ( 'NONE', #25870, #36371, #12821, .T. ) ;
#37726=EDGE_CURVE ( 'NONE', #23756, #25426, #37934, .T. ) ;
#37730=CIRCLE ( 'NONE', #18010, 0.1000000000000028644 ) ;
#37732=CARTESIAN_POINT ( 'NONE',  ( -5.078675913592192614, -26.64985754041175525, 6.700000000000000178 ) ) ;
#37740=DIRECTION ( 'NONE',  ( -0.000000000000000000, -0.000000000000000000, 1.000000000000000000 ) ) ;
#37742=ORIENTED_EDGE ( 'NONE', *, *, #11696, .F. ) ;
#37745=CIRCLE ( 'NONE', #20006, 0.1000000000000028644 ) ;
#37749=DIRECTION ( 'NONE',  ( -0.000000000000000000, -0.000000000000000000, 1.000000000000000000 ) ) ;
#37753=CARTESIAN_POINT ( 'NONE',  ( 3.121324086407806231, -26.64985754041175525, 6.800000000000000711 ) ) ;
#37756=DIRECTION ( 'NONE',  ( -1.000000000000000000, 0.000000000000000000, 0.000000000000000000 ) ) ;
#37772=CARTESIAN_POINT ( 'NONE',  ( -2.348748702180637693, -25.49307895267003587, 6.800000000000000711 ) ) ;
#37777=ORIENTED_EDGE ( 'NONE', *, *, #12329, .T. ) ;
#37786=ORIENTED_EDGE ( 'NONE', *, *, #3378, .T. ) ;
#37795=CIRCLE ( 'NONE', #2994, 0.1000000000000028644 ) ;
#37798=VECTOR ( 'NONE', #31408, 1000.000000000000000 ) ;
#37799=FACE_OUTER_BOUND ( 'NONE', #28179, .T. ) ;
#37801=CARTESIAN_POINT ( 'NONE',  ( -10.87867591359219155, -26.64985754041175525, 6.800000000000000711 ) ) ;
#37802=ORIENTED_EDGE ( 'NONE', *, *, #2692, .T. ) ;
#37803=VECTOR ( 'NONE', #11292, 1000.000000000000000 ) ;
#37819=EDGE_LOOP ( 'NONE', ( #39845, #26168, #4625, #15115 ) ) ;
#37822=ADVANCED_FACE ( 'NONE', ( #38332 ), #35287, .F. ) ;
#37824=VECTOR ( 'NONE', #8185, 1000.000000000000000 ) ;
#37829=DIRECTION ( 'NONE',  ( 0.000000000000000000, 0.000000000000000000, 1.000000000000000000 ) ) ;
#37833=AXIS2_PLACEMENT_3D ( 'NONE', #19520, #32101, #29392 ) ;
#37851=ORIENTED_EDGE ( 'NONE', *, *, #5402, .T. ) ;
#37853=VECTOR ( 'NONE', #1316, 1000.000000000000000 ) ;
#37854=DIRECTION ( 'NONE',  ( -0.000000000000000000, -0.000000000000000000, 1.000000000000000000 ) ) ;
#37858=CARTESIAN_POINT ( 'NONE',  ( -24.44874870218064089, -25.49307895267003587, 6.800000000000000711 ) ) ;
#37863=ORIENTED_EDGE ( 'NONE', *, *, #5735, .T. ) ;
#37865=ORIENTED_EDGE ( 'NONE', *, *, #30798, .F. ) ;
#37868=CARTESIAN_POINT ( 'NONE',  ( -1.078675913592196167, -24.55319635012989110, 6.700000000000000178 ) ) ;
#37884=ORIENTED_EDGE ( 'NONE', *, *, #24869, .T. ) ;
#37896=PLANE ( 'NONE',  #20744 ) ;
#37897=DIRECTION ( 'NONE',  ( 1.000000000000000000, 0.000000000000000000, 0.000000000000000000 ) ) ;
#37911=VERTEX_POINT ( 'NONE', #34203 ) ;
#37912=VERTEX_POINT ( 'NONE', #27781 ) ;
#37913=VECTOR ( 'NONE', #37995, 1000.000000000000000 ) ;
#37914=CARTESIAN_POINT ( 'NONE',  ( -39.07867591359219261, -26.64985754041175525, 6.700000000000000178 ) ) ;
#37924=DIRECTION ( 'NONE',  ( 0.000000000000000000, 0.000000000000000000, 1.000000000000000000 ) ) ;
#37934=LINE ( 'NONE', #9743, #39233 ) ;
#37939=DIRECTION ( 'NONE',  ( -0.000000000000000000, -0.000000000000000000, 1.000000000000000000 ) ) ;
#37941=CIRCLE ( 'NONE', #27459, 0.1000000000000028644 ) ;
#37946=VECTOR ( 'NONE', #30154, 1000.000000000000000 ) ;
#37948=AXIS2_PLACEMENT_3D ( 'NONE', #31614, #3437, #22761 ) ;
#37949=CARTESIAN_POINT ( 'NONE',  ( -16.97867591359219475, -26.64985754041175525, 6.700000000000000178 ) ) ;
#37953=ORIENTED_EDGE ( 'NONE', *, *, #34615, .T. ) ;
#37963=DIRECTION ( 'NONE',  ( -0.000000000000000000, -0.000000000000000000, 1.000000000000000000 ) ) ;
#37967=ORIENTED_EDGE ( 'NONE', *, *, #31579, .F. ) ;
#37983=CARTESIAN_POINT ( 'NONE',  ( -18.24874870218063450, -26.64985754041175525, 6.800000000000000711 ) ) ;
#37985=AXIS2_PLACEMENT_3D ( 'NONE', #39206, #38605, #10995 ) ;
#37990=EDGE_CURVE ( 'NONE', #33400, #30328, #3116, .T. ) ;
#37995=DIRECTION ( 'NONE',  ( -0.000000000000000000, -0.000000000000000000, 1.000000000000000000 ) ) ;
#37996=VECTOR ( 'NONE', #5055, 1000.000000000000000 ) ;
#38001=DIRECTION ( 'NONE',  ( 0.000000000000000000, 0.000000000000000000, -1.000000000000000000 ) ) ;
#38002=ADVANCED_FACE ( 'NONE', ( #33324 ), #17844, .F. ) ;
#38003=ORIENTED_EDGE ( 'NONE', *, *, #19032, .T. ) ;
#38004=CARTESIAN_POINT ( 'NONE',  ( -36.44874870218064444, -25.49307895267003587, 6.700000000000000178 ) ) ;
#38005=DIRECTION ( 'NONE',  ( 1.000000000000000000, 0.000000000000000000, 0.000000000000000000 ) ) ;
#38013=CYLINDRICAL_SURFACE ( 'NONE', #17271, 0.1000000000000028644 ) ;
#38016=EDGE_CURVE ( 'NONE', #8738, #3771, #39675, .T. ) ;
#38017=ADVANCED_FACE ( 'NONE', ( #11058 ), #11663, .F. ) ;
#38024=CARTESIAN_POINT ( 'NONE',  ( -8.248748702180632719, -25.49307895267003587, 6.700000000000000178 ) ) ;
#38032=VECTOR ( 'NONE', #23341, 1000.000000000000000 ) ;
#38034=CARTESIAN_POINT ( 'NONE',  ( -10.97867591359219475, -24.55319635012989110, 6.700000000000000178 ) ) ;
#38036=CARTESIAN_POINT ( 'NONE',  ( -18.24874870218063450, -25.49307895267003587, 6.800000000000000711 ) ) ;
#38038=PLANE ( 'NONE',  #8243 ) ;
#38045=VERTEX_POINT ( 'NONE', #22197 ) ;
#38050=LINE ( 'NONE', #9850, #21132 ) ;
#38061=EDGE_CURVE ( 'NONE', #18594, #38404, #14939, .T. ) ;
#38071=EDGE_LOOP ( 'NONE', ( #29760, #19131, #35407, #22585 ) ) ;
#38072=DIRECTION ( 'NONE',  ( 1.000000000000000000, -0.000000000000000000, 0.000000000000000000 ) ) ;
#38074=ORIENTED_EDGE ( 'NONE', *, *, #2408, .T. ) ;
#38087=ORIENTED_EDGE ( 'NONE', *, *, #25204, .T. ) ;
#38096=ADVANCED_FACE ( 'NONE', ( #18884 ), #27733, .F. ) ;
#38102=VERTEX_POINT ( 'NONE', #28562 ) ;
#38103=FACE_BOUND ( 'NONE', #970, .T. ) ;
#38104=CARTESIAN_POINT ( 'NONE',  ( -24.34874870218063592, -26.64985754041175525, 6.800000000000000711 ) ) ;
#38110=ORIENTED_EDGE ( 'NONE', *, *, #19990, .F. ) ;
#38131=DIRECTION ( 'NONE',  ( 0.000000000000000000, 0.000000000000000000, 1.000000000000000000 ) ) ;
#38141=ORIENTED_EDGE ( 'NONE', *, *, #543, .T. ) ;
#38150=CARTESIAN_POINT ( 'NONE',  ( 5.751251297819365504, -25.49307895267003587, 6.800000000000000711 ) ) ;
#38153=CARTESIAN_POINT ( 'NONE',  ( -40.34874870218063592, -25.49307895267003587, 6.800000000000000711 ) ) ;
#38171=VERTEX_POINT ( 'NONE', #34156 ) ;
#38183=DIRECTION ( 'NONE',  ( 1.000000000000000000, -0.000000000000000000, 0.000000000000000000 ) ) ;
#38184=AXIS2_PLACEMENT_3D ( 'NONE', #27460, #36931, #40015 ) ;
#38185=CARTESIAN_POINT ( 'NONE',  ( -9.078675913592196167, -24.55319635012989110, 6.700000000000000178 ) ) ;
#38199=LINE ( 'NONE', #26466, #25165 ) ;
#38203=EDGE_LOOP ( 'NONE', ( #11916, #31525, #32704, #29812 ) ) ;
#38207=CARTESIAN_POINT ( 'NONE',  ( -34.44874870218064444, -25.49307895267003587, 6.700000000000000178 ) ) ;
#38209=AXIS2_PLACEMENT_3D ( 'NONE', #23266, #4536, #7207 ) ;
#38210=DIRECTION ( 'NONE',  ( -1.000000000000000000, 0.000000000000000000, 0.000000000000000000 ) ) ;
#38219=ORIENTED_EDGE ( 'NONE', *, *, #28685, .T. ) ;
#38221=CARTESIAN_POINT ( 'NONE',  ( -11.07867591359219794, -26.64985754041175525, 6.700000000000000178 ) ) ;
#38225=DIRECTION ( 'NONE',  ( 0.000000000000000000, 1.000000000000000000, 0.000000000000000000 ) ) ;
#38242=ORIENTED_EDGE ( 'NONE', *, *, #17587, .F. ) ;
#38249=DIRECTION ( 'NONE',  ( 1.000000000000000000, 0.000000000000000000, 0.000000000000000000 ) ) ;
#38250=EDGE_LOOP ( 'NONE', ( #1846, #37585, #9539, #27319 ) ) ;
#38252=EDGE_CURVE ( 'NONE', #36487, #25629, #24842, .T. ) ;
#38254=ORIENTED_EDGE ( 'NONE', *, *, #36082, .F. ) ;
#38255=ORIENTED_EDGE ( 'NONE', *, *, #5858, .T. ) ;
#38262=ADVANCED_FACE ( 'NONE', ( #2635 ), #34133, .F. ) ;
#38268=ORIENTED_EDGE ( 'NONE', *, *, #4572, .F. ) ;
#38271=FACE_OUTER_BOUND ( 'NONE', #21401, .T. ) ;
#38272=ORIENTED_EDGE ( 'NONE', *, *, #34462, .T. ) ;
#38278=ORIENTED_EDGE ( 'NONE', *, *, #35312, .F. ) ;
#38282=CARTESIAN_POINT ( 'NONE',  ( -10.24874870218063450, -25.49307895267003587, 6.700000000000000178 ) ) ;
#38284=CARTESIAN_POINT ( 'NONE',  ( -34.44874870218064444, -26.64985754041175525, 6.700000000000000178 ) ) ;
#38285=LINE ( 'NONE', #32147, #27255 ) ;
#38287=ORIENTED_EDGE ( 'NONE', *, *, #35567, .F. ) ;
#38291=ORIENTED_EDGE ( 'NONE', *, *, #32049, .T. ) ;
#38297=EDGE_CURVE ( 'NONE', #19232, #2584, #19574, .T. ) ;
#38298=EDGE_LOOP ( 'NONE', ( #7319, #24281, #9547, #28279 ) ) ;
#38301=EDGE_LOOP ( 'NONE', ( #19892, #3909, #39932, #31708 ) ) ;
#38302=CARTESIAN_POINT ( 'NONE',  ( 11.65737507970504616, -30.94667987854474234, 6.800000000000000711 ) ) ;
#38303=DIRECTION ( 'NONE',  ( 0.000000000000000000, 0.000000000000000000, 1.000000000000000000 ) ) ;
#38304=ORIENTED_EDGE ( 'NONE', *, *, #21484, .T. ) ;
#38310=CARTESIAN_POINT ( 'NONE',  ( -3.078675913592197944, -26.64985754041175525, 6.700000000000000178 ) ) ;
#38314=ORIENTED_EDGE ( 'NONE', *, *, #21484, .F. ) ;
#38315=VECTOR ( 'NONE', #5657, 1000.000000000000000 ) ;
#38323=CARTESIAN_POINT ( 'NONE',  ( 3.121324086407806231, -26.64985754041175525, 6.700000000000000178 ) ) ;
#38325=PLANE ( 'NONE',  #32855 ) ;
#38332=FACE_OUTER_BOUND ( 'NONE', #17943, .T. ) ;
#38340=MECHANICAL_DESIGN_GEOMETRIC_PRESENTATION_REPRESENTATION('',(#15334),#16612);
#38342=ORIENTED_EDGE ( 'NONE', *, *, #36132, .F. ) ;
#38344=EDGE_CURVE ( 'NONE', #25619, #25932, #1166, .T. ) ;
#38349=DIRECTION ( 'NONE',  ( 1.000000000000000000, 0.000000000000000000, 0.000000000000000000 ) ) ;
#38350=DIRECTION ( 'NONE',  ( -0.000000000000000000, -0.000000000000000000, 1.000000000000000000 ) ) ;
#38353=DIRECTION ( 'NONE',  ( 0.000000000000000000, 0.000000000000000000, 1.000000000000000000 ) ) ;
#38355=VECTOR ( 'NONE', #4435, 1000.000000000000000 ) ;
#38356=DIRECTION ( 'NONE',  ( -0.000000000000000000, -0.000000000000000000, 1.000000000000000000 ) ) ;
#38374=CARTESIAN_POINT ( 'NONE',  ( -42.83131703149249603, -32.06993018339340296, 6.800000000000000711 ) ) ;
#38379=DIRECTION ( 'NONE',  ( 1.000000000000000000, 0.000000000000000000, 0.000000000000000000 ) ) ;
#38382=CIRCLE ( 'NONE', #25912, 7.341749246864647915 ) ;
#38388=ADVANCED_FACE ( 'NONE', ( #12481 ), #39198, .F. ) ;
#38389=EDGE_CURVE ( 'NONE', #18938, #24066, #32077, .T. ) ;
#38390=CIRCLE ( 'NONE', #7485, 0.1000000000000028644 ) ;
#38395=ORIENTED_EDGE ( 'NONE', *, *, #35636, .T. ) ;
#38400=EDGE_LOOP ( 'NONE', ( #32995, #9072, #32053, #1886, #9992 ) ) ;
#38404=VERTEX_POINT ( 'NONE', #1759 ) ;
#38410=DIRECTION ( 'NONE',  ( -0.000000000000000000, -0.000000000000000000, 1.000000000000000000 ) ) ;
#38414=LINE ( 'NONE', #35953, #32123 ) ;
#38420=CARTESIAN_POINT ( 'NONE',  ( 3.651251297819360531, -26.64985754041175525, 6.800000000000000711 ) ) ;
#38427=DIRECTION ( 'NONE',  ( 0.000000000000000000, 0.000000000000000000, 1.000000000000000000 ) ) ;
#38429=CARTESIAN_POINT ( 'NONE',  ( 0.9213240864078056092, -26.64985754041175525, 6.700000000000000178 ) ) ;
#38437=CIRCLE ( 'NONE', #34546, 0.1000000000000028644 ) ;
#38439=ADVANCED_FACE ( 'NONE', ( #35543 ), #19680, .T. ) ;
#38443=DIRECTION ( 'NONE',  ( -0.000000000000000000, -1.000000000000000000, -0.000000000000000000 ) ) ;
#38445=PLANE ( 'NONE',  #23403 ) ;
#38446=VECTOR ( 'NONE', #17932, 1000.000000000000000 ) ;
#38449=ORIENTED_EDGE ( 'NONE', *, *, #2853, .F. ) ;
#38452=DIRECTION ( 'NONE',  ( 0.000000000000000000, 0.000000000000000000, 1.000000000000000000 ) ) ;
#38456=FACE_OUTER_BOUND ( 'NONE', #40123, .T. ) ;
#38459=CARTESIAN_POINT ( 'NONE',  ( -20.24874870218063805, -25.49307895267003587, 6.700000000000000178 ) ) ;
#38462=EDGE_CURVE ( 'NONE', #18594, #35446, #4242, .T. ) ;
#38464=ORIENTED_EDGE ( 'NONE', *, *, #12742, .T. ) ;
#38489=VERTEX_POINT ( 'NONE', #17778 ) ;
#38492=CARTESIAN_POINT ( 'NONE',  ( -6.978675913592191193, -24.55319635012989110, 6.800000000000000711 ) ) ;
#38495=VERTEX_POINT ( 'NONE', #33876 ) ;
#38497=VERTEX_POINT ( 'NONE', #39828 ) ;
#38499=ORIENTED_EDGE ( 'NONE', *, *, #13641, .T. ) ;
#38504=AXIS2_PLACEMENT_3D ( 'NONE', #32221, #35512, #22549 ) ;
#38512=FACE_OUTER_BOUND ( 'NONE', #10270, .T. ) ;
#38514=EDGE_LOOP ( 'NONE', ( #31729, #12221, #13725, #3931 ) ) ;
#38522=EDGE_CURVE ( 'NONE', #18637, #24328, #8926, .T. ) ;
#38527=CARTESIAN_POINT ( 'NONE',  ( -18.87867591359219333, -26.64985754041175525, 6.700000000000000178 ) ) ;
#38535=AXIS2_PLACEMENT_3D ( 'NONE', #14413, #1682, #4753 ) ;
#38542=DIRECTION ( 'NONE',  ( 1.000000000000000000, 0.000000000000000000, 0.000000000000000000 ) ) ;
#38544=DIRECTION ( 'NONE',  ( 1.000000000000000000, 0.000000000000000000, 0.000000000000000000 ) ) ;
#38559=VECTOR ( 'NONE', #34184, 1000.000000000000000 ) ;
#38562=CIRCLE ( 'NONE', #13594, 0.1000000000000028644 ) ;
#38563=ORIENTED_EDGE ( 'NONE', *, *, #1249, .F. ) ;
#38567=EDGE_CURVE ( 'NONE', #31406, #11548, #27870, .T. ) ;
#38584=CARTESIAN_POINT ( 'NONE',  ( -42.44874870218064444, -25.49307895267003587, 6.800000000000000711 ) ) ;
#38585=AXIS2_PLACEMENT_3D ( 'NONE', #26536, #10071, #23446 ) ;
#38586=LINE ( 'NONE', #19467, #37472 ) ;
#38589=CARTESIAN_POINT ( 'NONE',  ( -6.448748702180637338, -26.64985754041175525, 6.700000000000000178 ) ) ;
#38605=DIRECTION ( 'NONE',  ( 1.000000000000000000, -0.000000000000000000, 0.000000000000000000 ) ) ;
#38606=VERTEX_POINT ( 'NONE', #26616 ) ;
#38607=ORIENTED_EDGE ( 'NONE', *, *, #18400, .T. ) ;
#38613=DIRECTION ( 'NONE',  ( 0.000000000000000000, 0.000000000000000000, 1.000000000000000000 ) ) ;
#38614=DIRECTION ( 'NONE',  ( 0.000000000000000000, 1.000000000000000000, 0.000000000000000000 ) ) ;
#38622=DIRECTION ( 'NONE',  ( -0.000000000000000000, -0.000000000000000000, 1.000000000000000000 ) ) ;
#38623=VECTOR ( 'NONE', #30574, 1000.000000000000000 ) ;
#38628=EDGE_CURVE ( 'NONE', #7900, #17955, #35496, .T. ) ;
#38631=DIRECTION ( 'NONE',  ( 1.000000000000000000, 0.000000000000000000, 0.000000000000000000 ) ) ;
#38637=LINE ( 'NONE', #38429, #16437 ) ;
#38641=CIRCLE ( 'NONE', #12338, 0.1000000000000028644 ) ;
#38647=AXIS2_PLACEMENT_3D ( 'NONE', #11078, #20157, #23649 ) ;
#38650=ORIENTED_EDGE ( 'NONE', *, *, #25531, .T. ) ;
#38652=ORIENTED_EDGE ( 'NONE', *, *, #2886, .F. ) ;
#38654=ORIENTED_EDGE ( 'NONE', *, *, #32705, .T. ) ;
#38665=CARTESIAN_POINT ( 'NONE',  ( -30.34874870218063947, -25.49307895267003587, 6.800000000000000711 ) ) ;
#38675=ORIENTED_EDGE ( 'NONE', *, *, #10916, .T. ) ;
#38676=CARTESIAN_POINT ( 'NONE',  ( -10.34874870218063769, -26.64985754041175525, 6.700000000000000178 ) ) ;
#38686=CARTESIAN_POINT ( 'NONE',  ( -6.348748702180634140, -25.49307895267003587, 6.700000000000000178 ) ) ;
#38691=AXIS2_PLACEMENT_3D ( 'NONE', #8086, #30965, #8700 ) ;
#38692=VERTEX_POINT ( 'NONE', #4007 ) ;
#38703=DIRECTION ( 'NONE',  ( 1.000000000000000000, 0.000000000000000000, 0.000000000000000000 ) ) ;
#38707=EDGE_LOOP ( 'NONE', ( #12901, #2435, #38816, #33351 ) ) ;
#38711=EDGE_CURVE ( 'NONE', #8281, #24389, #27210, .T. ) ;
#38712=DIRECTION ( 'NONE',  ( 0.000000000000000000, 0.000000000000000000, 1.000000000000000000 ) ) ;
#38720=LINE ( 'NONE', #35269, #27370 ) ;
#38722=ADVANCED_FACE ( 'NONE', ( #30515 ), #11544, .F. ) ;
#38732=DIRECTION ( 'NONE',  ( -0.000000000000000000, -1.000000000000000000, -0.000000000000000000 ) ) ;
#38736=DIRECTION ( 'NONE',  ( -0.000000000000000000, -1.000000000000000000, -0.000000000000000000 ) ) ;
#38739=VECTOR ( 'NONE', #29130, 1000.000000000000000 ) ;
#38740=EDGE_CURVE ( 'NONE', #39064, #9395, #2324, .T. ) ;
#38741=DIRECTION ( 'NONE',  ( -0.000000000000000000, -0.000000000000000000, 1.000000000000000000 ) ) ;
#38748=DIRECTION ( 'NONE',  ( 0.000000000000000000, 0.000000000000000000, 1.000000000000000000 ) ) ;
#38750=FACE_OUTER_BOUND ( 'NONE', #31090, .T. ) ;
#38751=VECTOR ( 'NONE', #31104, 1000.000000000000000 ) ;
#38771=VECTOR ( 'NONE', #10608, 1000.000000000000000 ) ;
#38778=VERTEX_POINT ( 'NONE', #33818 ) ;
#38784=VECTOR ( 'NONE', #22160, 1000.000000000000000 ) ;
#38788=CARTESIAN_POINT ( 'NONE',  ( -6.448748702180637338, -26.64985754041175525, 6.800000000000000711 ) ) ;
#38795=ORIENTED_EDGE ( 'NONE', *, *, #39545, .T. ) ;
#38808=DIRECTION ( 'NONE',  ( 1.000000000000000000, 0.000000000000000000, 0.000000000000000000 ) ) ;
#38809=VECTOR ( 'NONE', #32344, 1000.000000000000000 ) ;
#38813=EDGE_CURVE ( 'NONE', #1662, #4028, #26120, .T. ) ;
#38816=ORIENTED_EDGE ( 'NONE', *, *, #16777, .F. ) ;
#38837=CARTESIAN_POINT ( 'NONE',  ( -22.97867591359219119, -26.64985754041175525, 6.700000000000000178 ) ) ;
#38843=LINE ( 'NONE', #4490, #40437 ) ;
#38845=EDGE_CURVE ( 'NONE', #9487, #19232, #18920, .T. ) ;
#38851=VECTOR ( 'NONE', #34668, 1000.000000000000000 ) ;
#38854=EDGE_CURVE ( 'NONE', #2584, #26610, #26516, .T. ) ;
#38858=ORIENTED_EDGE ( 'NONE', *, *, #36524, .T. ) ;
#38860=CARTESIAN_POINT ( 'NONE',  ( -27.07867591359219972, -26.64985754041175525, 6.700000000000000178 ) ) ;
#38864=VECTOR ( 'NONE', #9228, 1000.000000000000000 ) ;
#38867=LINE ( 'NONE', #7780, #33495 ) ;
#38869=CARTESIAN_POINT ( 'NONE',  ( -26.87867591359219333, -24.55319635012989110, 6.700000000000000178 ) ) ;
#38873=DIRECTION ( 'NONE',  ( 1.000000000000000000, 0.000000000000000000, 0.000000000000000000 ) ) ;
#38877=CARTESIAN_POINT ( 'NONE',  ( -14.87867591359218977, -26.64985754041175525, 6.800000000000000711 ) ) ;
#38889=DIRECTION ( 'NONE',  ( 0.000000000000000000, 0.000000000000000000, -1.000000000000000000 ) ) ;
#38895=ORIENTED_EDGE ( 'NONE', *, *, #3378, .F. ) ;
#38905=VERTEX_POINT ( 'NONE', #13947 ) ;
#38907=LINE ( 'NONE', #14592, #30449 ) ;
#38911=LINE ( 'NONE', #1074, #12071 ) ;
#38923=DIRECTION ( 'NONE',  ( -0.000000000000000000, -0.000000000000000000, 1.000000000000000000 ) ) ;
#38928=CARTESIAN_POINT ( 'NONE',  ( 11.65737507970504616, -38.28842912540938670, 6.800000000000000711 ) ) ;
#38933=CARTESIAN_POINT ( 'NONE',  ( -42.34874870218063592, -26.64985754041175525, 6.700000000000000178 ) ) ;
#38953=EDGE_LOOP ( 'NONE', ( #31285, #4924, #29847, #11471 ) ) ;
#38965=LINE ( 'NONE', #10764, #38032 ) ;
#38969=EDGE_LOOP ( 'NONE', ( #24119, #31138, #13086, #11707 ) ) ;
#38979=DIRECTION ( 'NONE',  ( -0.000000000000000000, -0.000000000000000000, 1.000000000000000000 ) ) ;
#38981=DIRECTION ( 'NONE',  ( 0.000000000000000000, 0.000000000000000000, 1.000000000000000000 ) ) ;
#38982=AXIS2_PLACEMENT_3D ( 'NONE', #38104, #32359, #35051 ) ;
#38986=ORIENTED_EDGE ( 'NONE', *, *, #15363, .F. ) ;
#38990=AXIS2_PLACEMENT_3D ( 'NONE', #24334, #36897, #33829 ) ;
#38992=EDGE_CURVE ( 'NONE', #34807, #12332, #30834, .T. ) ;
#38996=FACE_OUTER_BOUND ( 'NONE', #36945, .T. ) ;
#38999=VERTEX_POINT ( 'NONE', #2643 ) ;
#39005=ADVANCED_FACE ( 'NONE', ( #40467 ), #33930, .T. ) ;
#39008=DIRECTION ( 'NONE',  ( -0.000000000000000000, -0.000000000000000000, 1.000000000000000000 ) ) ;
#39016=CARTESIAN_POINT ( 'NONE',  ( -53.21549048184568420, -38.28842912540938670, 6.000000000000000000 ) ) ;
#39024=EDGE_CURVE ( 'NONE', #6453, #19329, #31236, .T. ) ;
#39025=ADVANCED_FACE ( 'NONE', ( #30630 ), #34142, .F. ) ;
#39026=ADVANCED_FACE ( 'NONE', ( #5910 ), #15577, .F. ) ;
#39027=AXIS2_PLACEMENT_3D ( 'NONE', #27717, #24429, #30197 ) ;
#39029=CARTESIAN_POINT ( 'NONE',  ( -30.44874870218064089, -25.49307895267003587, 6.700000000000000178 ) ) ;
#39035=VERTEX_POINT ( 'NONE', #28131 ) ;
#39045=ORIENTED_EDGE ( 'NONE', *, *, #24551, .F. ) ;
#39048=CIRCLE ( 'NONE', #4881, 0.1000000000000028644 ) ;
#39049=ORIENTED_EDGE ( 'NONE', *, *, #10460, .F. ) ;
#39051=DIRECTION ( 'NONE',  ( 0.000000000000000000, 0.000000000000000000, 1.000000000000000000 ) ) ;
#39054=VERTEX_POINT ( 'NONE', #39872 ) ;
#39061=LINE ( 'NONE', #38459, #6062 ) ;
#39064=VERTEX_POINT ( 'NONE', #759 ) ;
#39066=ADVANCED_FACE ( 'NONE', ( #25057 ), #32060, .T. ) ;
#39080=CIRCLE ( 'NONE', #14100, 0.1000000000000028644 ) ;
#39084=LINE ( 'NONE', #14567, #27300 ) ;
#39087=ORIENTED_EDGE ( 'NONE', *, *, #23159, .F. ) ;
#39088=CARTESIAN_POINT ( 'NONE',  ( -32.97867591359219119, -26.64985754041175525, 6.700000000000000178 ) ) ;
#39089=AXIS2_PLACEMENT_3D ( 'NONE', #25860, #35549, #6728 ) ;
#39090=DIRECTION ( 'NONE',  ( 0.000000000000000000, 0.000000000000000000, 1.000000000000000000 ) ) ;
#39099=ORIENTED_EDGE ( 'NONE', *, *, #23790, .T. ) ;
#39100=EDGE_LOOP ( 'NONE', ( #4507, #6744, #30776, #7164 ) ) ;
#39103=CARTESIAN_POINT ( 'NONE',  ( -6.448748702180637338, -25.49307895267003587, 6.700000000000000178 ) ) ;
#39109=AXIS2_PLACEMENT_3D ( 'NONE', #34787, #15399, #12310 ) ;
#39111=DIRECTION ( 'NONE',  ( 1.000000000000000000, 0.000000000000000000, 0.000000000000000000 ) ) ;
#39119=CARTESIAN_POINT ( 'NONE',  ( -30.24874870218063450, -26.64985754041175525, 6.800000000000000711 ) ) ;
#39120=AXIS2_PLACEMENT_3D ( 'NONE', #10794, #39615, #33477 ) ;
#39123=DIRECTION ( 'NONE',  ( 1.000000000000000000, -0.000000000000000000, 0.000000000000000000 ) ) ;
#39124=CARTESIAN_POINT ( 'NONE',  ( -20.24874870218063805, -25.49307895267003587, 6.700000000000000178 ) ) ;
#39129=EDGE_CURVE ( 'NONE', #22571, #39924, #10001, .T. ) ;
#39130=EDGE_CURVE ( 'NONE', #18363, #9395, #31643, .T. ) ;
#39133=EDGE_CURVE ( 'NONE', #35180, #33558, #25418, .T. ) ;
#39139=CARTESIAN_POINT ( 'NONE',  ( 5.651251297819362307, -25.49307895267003587, 6.700000000000000178 ) ) ;
#39141=VERTEX_POINT ( 'NONE', #15978 ) ;
#39148=LINE ( 'NONE', #7867, #22663 ) ;
#39156=FACE_OUTER_BOUND ( 'NONE', #18807, .T. ) ;
#39158=DIRECTION ( 'NONE',  ( 0.000000000000000000, 0.000000000000000000, 1.000000000000000000 ) ) ;
#39165=VECTOR ( 'NONE', #9577, 1000.000000000000000 ) ;
#39170=FACE_OUTER_BOUND ( 'NONE', #32565, .T. ) ;
#39171=EDGE_LOOP ( 'NONE', ( #26505, #38087, #15664, #27118 ) ) ;
#39177=VECTOR ( 'NONE', #4805, 1000.000000000000000 ) ;
#39181=EDGE_CURVE ( 'NONE', #12640, #22571, #28544, .T. ) ;
#39188=PLANE ( 'NONE',  #719 ) ;
#39191=ORIENTED_EDGE ( 'NONE', *, *, #2114, .T. ) ;
#39198=PLANE ( 'NONE',  #27435 ) ;
#39200=DIRECTION ( 'NONE',  ( -0.000000000000000000, -0.000000000000000000, 1.000000000000000000 ) ) ;
#39201=EDGE_CURVE ( 'NONE', #13011, #6524, #16382, .T. ) ;
#39205=CARTESIAN_POINT ( 'NONE',  ( -26.87867591359219333, -26.64985754041175525, 6.700000000000000178 ) ) ;
#39206=CARTESIAN_POINT ( 'NONE',  ( -10.24874870218063450, -26.64985754041175525, 6.700000000000000178 ) ) ;
#39208=ORIENTED_EDGE ( 'NONE', *, *, #34910, .T. ) ;
#39212=DIRECTION ( 'NONE',  ( 1.000000000000000000, 0.000000000000000000, 0.000000000000000000 ) ) ;
#39213=EDGE_CURVE ( 'NONE', #24867, #20522, #13559, .T. ) ;
#39219=EDGE_LOOP ( 'NONE', ( #21148, #37214, #20173, #36835 ) ) ;
#39220=CARTESIAN_POINT ( 'NONE',  ( -28.87867591359218977, -26.64985754041175525, 6.700000000000000178 ) ) ;
#39228=DIRECTION ( 'NONE',  ( 0.000000000000000000, 0.000000000000000000, 1.000000000000000000 ) ) ;
#39230=CARTESIAN_POINT ( 'NONE',  ( 4.921324086407802056, -26.64985754041175525, 6.700000000000000178 ) ) ;
#39233=VECTOR ( 'NONE', #22321, 1000.000000000000000 ) ;
#39243=DIRECTION ( 'NONE',  ( 0.000000000000000000, 0.000000000000000000, 1.000000000000000000 ) ) ;
#39246=ORIENTED_EDGE ( 'NONE', *, *, #29433, .T. ) ;
#39249=ORIENTED_EDGE ( 'NONE', *, *, #29895, .T. ) ;
#39251=VECTOR ( 'NONE', #9207, 1000.000000000000000 ) ;
#39260=ORIENTED_EDGE ( 'NONE', *, *, #5391, .F. ) ;
#39261=AXIS2_PLACEMENT_3D ( 'NONE', #28948, #18645, #3050 ) ;
#39263=PLANE ( 'NONE',  #21325 ) ;
#39269=ORIENTED_EDGE ( 'NONE', *, *, #27126, .F. ) ;
#39271=ORIENTED_EDGE ( 'NONE', *, *, #33943, .F. ) ;
#39276=EDGE_CURVE ( 'NONE', #5299, #29204, #32856, .T. ) ;
#39282=VERTEX_POINT ( 'NONE', #1765 ) ;
#39283=FACE_OUTER_BOUND ( 'NONE', #22723, .T. ) ;
#39295=DIRECTION ( 'NONE',  ( 0.000000000000000000, 0.000000000000000000, 1.000000000000000000 ) ) ;
#39298=ORIENTED_EDGE ( 'NONE', *, *, #8349, .T. ) ;
#39300=DIRECTION ( 'NONE',  ( -0.000000000000000000, -0.000000000000000000, 1.000000000000000000 ) ) ;
#39302=EDGE_CURVE ( 'NONE', #3866, #3076, #16835, .T. ) ;
#39304=ORIENTED_EDGE ( 'NONE', *, *, #2791, .F. ) ;
#39310=ORIENTED_EDGE ( 'NONE', *, *, #32681, .T. ) ;
#39312=ADVANCED_FACE ( 'NONE', ( #16980 ), #26072, .F. ) ;
#39314=CARTESIAN_POINT ( 'NONE',  ( -39.07867591359219261, -26.64985754041175525, 6.800000000000000711 ) ) ;
#39315=CARTESIAN_POINT ( 'NONE',  ( -40.97867591359219119, -26.64985754041175525, 6.700000000000000178 ) ) ;
#39323=ORIENTED_EDGE ( 'NONE', *, *, #29394, .T. ) ;
#39325=VECTOR ( 'NONE', #33904, 1000.000000000000000 ) ;
#39327=CARTESIAN_POINT ( 'NONE',  ( -54.01549048184568846, -30.38627270959228710, 4.800000000000001599 ) ) ;
#39337=AXIS2_PLACEMENT_3D ( 'NONE', #7633, #29466, #10108 ) ;
#39342=DIRECTION ( 'NONE',  ( 0.000000000000000000, 0.000000000000000000, 1.000000000000000000 ) ) ;
#39356=DIRECTION ( 'NONE',  ( -0.000000000000000000, -0.000000000000000000, 1.000000000000000000 ) ) ;
#39362=VECTOR ( 'NONE', #5103, 1000.000000000000000 ) ;
#39398=ORIENTED_EDGE ( 'NONE', *, *, #5963, .T. ) ;
#39407=EDGE_CURVE ( 'NONE', #28211, #16705, #8961, .T. ) ;
#39416=DIRECTION ( 'NONE',  ( -0.000000000000000000, -0.000000000000000000, 1.000000000000000000 ) ) ;
#39417=CIRCLE ( 'NONE', #21043, 0.1000000000000028644 ) ;
#39421=ORIENTED_EDGE ( 'NONE', *, *, #15724, .T. ) ;
#39428=CARTESIAN_POINT ( 'NONE',  ( -36.24874870218063450, -26.64985754041175525, 6.800000000000000711 ) ) ;
#39432=VECTOR ( 'NONE', #9987, 1000.000000000000000 ) ;
#39436=DIRECTION ( 'NONE',  ( -0.000000000000000000, -0.000000000000000000, 1.000000000000000000 ) ) ;
#39441=DIRECTION ( 'NONE',  ( 1.000000000000000000, 0.000000000000000000, 0.000000000000000000 ) ) ;
#39443=VECTOR ( 'NONE', #24963, 1000.000000000000000 ) ;
#39450=VERTEX_POINT ( 'NONE', #11399 ) ;
#39453=EDGE_CURVE ( 'NONE', #15824, #30074, #5455, .T. ) ;
#39454=ORIENTED_EDGE ( 'NONE', *, *, #12683, .T. ) ;
#39460=AXIS2_PLACEMENT_3D ( 'NONE', #17713, #5382, #39756 ) ;
#39474=VECTOR ( 'NONE', #12567, 1000.000000000000000 ) ;
#39475=LINE ( 'NONE', #5315, #4509 ) ;
#39476=CARTESIAN_POINT ( 'NONE',  ( -2.878675913592191993, -24.55319635012989110, 6.700000000000000178 ) ) ;
#39479=DIRECTION ( 'NONE',  ( -0.000000000000000000, -0.000000000000000000, 1.000000000000000000 ) ) ;
#39481=ADVANCED_FACE ( 'NONE', ( #15118 ), #2388, .F. ) ;
#39485=CARTESIAN_POINT ( 'NONE',  ( -17.07867591359219617, -24.55319635012989110, 6.800000000000000711 ) ) ;
#39491=EDGE_CURVE ( 'NONE', #24999, #26805, #14870, .T. ) ;
#39496=ORIENTED_EDGE ( 'NONE', *, *, #14563, .T. ) ;
#39501=CARTESIAN_POINT ( 'NONE',  ( -35.07867591359219972, -26.64985754041175525, 6.800000000000000711 ) ) ;
#39505=AXIS2_PLACEMENT_3D ( 'NONE', #36778, #18031, #8561 ) ;
#39506=ORIENTED_EDGE ( 'NONE', *, *, #32242, .T. ) ;
#39510=ORIENTED_EDGE ( 'NONE', *, *, #40021, .F. ) ;
#39514=PLANE ( 'NONE',  #8506 ) ;
#39519=ORIENTED_EDGE ( 'NONE', *, *, #31728, .T. ) ;
#39525=ORIENTED_EDGE ( 'NONE', *, *, #14221, .F. ) ;
#39526=LINE ( 'NONE', #17287, #26074 ) ;
#39531=DIRECTION ( 'NONE',  ( 0.000000000000000000, 1.000000000000000000, 0.000000000000000000 ) ) ;
#39533=SHAPE_REPRESENTATION ( 'Measuring Ruler', ( #30744 ), #40552 ) ;
#39543=EDGE_CURVE ( 'NONE', #24757, #33685, #25609, .T. ) ;
#39545=EDGE_CURVE ( 'NONE', #13364, #31915, #24098, .T. ) ;
#39547=DIRECTION ( 'NONE',  ( 1.000000000000000000, 0.000000000000000000, 0.000000000000000000 ) ) ;
#39567=DIRECTION ( 'NONE',  ( -0.000000000000000000, -1.000000000000000000, -0.000000000000000000 ) ) ;
#39571=FACE_OUTER_BOUND ( 'NONE', #16098, .T. ) ;
#39591=ADVANCED_FACE ( 'NONE', ( #3009 ), #40636, .F. ) ;
#39592=DIRECTION ( 'NONE',  ( 0.000000000000000000, 1.000000000000000000, 0.000000000000000000 ) ) ;
#39602=ADVANCED_FACE ( 'NONE', ( #31390 ), #31795, .F. ) ;
#39607=ORIENTED_EDGE ( 'NONE', *, *, #27615, .F. ) ;
#39608=LINE ( 'NONE', #27257, #15373 ) ;
#39609=CARTESIAN_POINT ( 'NONE',  ( -6.248748702180631831, -26.64985754041175525, 6.700000000000000178 ) ) ;
#39615=DIRECTION ( 'NONE',  ( -0.000000000000000000, -0.000000000000000000, 1.000000000000000000 ) ) ;
#39625=DIRECTION ( 'NONE',  ( 0.000000000000000000, 1.000000000000000000, 0.000000000000000000 ) ) ;
#39631=VECTOR ( 'NONE', #21293, 1000.000000000000000 ) ;
#39638=DIRECTION ( 'NONE',  ( 1.000000000000000000, 0.000000000000000000, 0.000000000000000000 ) ) ;
#39644=DIRECTION ( 'NONE',  ( 0.000000000000000000, 0.000000000000000000, 1.000000000000000000 ) ) ;
#39645=ADVANCED_FACE ( 'NONE', ( #9341 ), #12842, .T. ) ;
#39647=VERTEX_POINT ( 'NONE', #6269 ) ;
#39655=DIRECTION ( 'NONE',  ( -0.000000000000000000, -0.000000000000000000, 1.000000000000000000 ) ) ;
#39659=EDGE_LOOP ( 'NONE', ( #33276, #26470, #22631, #25007 ) ) ;
#39661=VERTEX_POINT ( 'NONE', #31595 ) ;
#39673=PLANE ( 'NONE',  #30873 ) ;
#39674=CARTESIAN_POINT ( 'NONE',  ( -0.3487487021806359722, -26.64985754041175525, 6.700000000000000178 ) ) ;
#39675=LINE ( 'NONE', #29809, #32713 ) ;
#39679=DIRECTION ( 'NONE',  ( 0.000000000000000000, 1.000000000000000000, 0.000000000000000000 ) ) ;
#39686=LINE ( 'NONE', #36609, #25973 ) ;
#39695=DIRECTION ( 'NONE',  ( 0.000000000000000000, 0.000000000000000000, 1.000000000000000000 ) ) ;
#39696=EDGE_LOOP ( 'NONE', ( #26430, #3964, #7354, #239 ) ) ;
#39698=AXIS2_PLACEMENT_3D ( 'NONE', #6061, #18595, #31181 ) ;
#39706=DIRECTION ( 'NONE',  ( 0.000000000000000000, 1.000000000000000000, 0.000000000000000000 ) ) ;
#39709=DIRECTION ( 'NONE',  ( 0.000000000000000000, 0.000000000000000000, 1.000000000000000000 ) ) ;
#39710=AXIS2_PLACEMENT_3D ( 'NONE', #13753, #31535, #13943 ) ;
#39715=AXIS2_PLACEMENT_3D ( 'NONE', #27778, #22031, #5968 ) ;
#39721=DIRECTION ( 'NONE',  ( 0.000000000000000000, 0.000000000000000000, 1.000000000000000000 ) ) ;
#39729=LINE ( 'NONE', #11512, #36936 ) ;
#39735=VECTOR ( 'NONE', #7262, 1000.000000000000000 ) ;
#39737=VECTOR ( 'NONE', #17146, 1000.000000000000000 ) ;
#39738=CYLINDRICAL_SURFACE ( 'NONE', #16391, 0.1000000000000028644 ) ;
#39744=CARTESIAN_POINT ( 'NONE',  ( -30.24874870218063450, -26.64985754041175525, 6.700000000000000178 ) ) ;
#39745=LINE ( 'NONE', #2298, #11539 ) ;
#39754=CARTESIAN_POINT ( 'NONE',  ( -27.07867591359219972, -26.64985754041175525, 6.700000000000000178 ) ) ;
#39756=DIRECTION ( 'NONE',  ( 1.000000000000000000, 0.000000000000000000, 0.000000000000000000 ) ) ;
#39757=VERTEX_POINT ( 'NONE', #1125 ) ;
#39764=AXIS2_PLACEMENT_3D ( 'NONE', #23308, #32190, #29679 ) ;
#39765=ORIENTED_EDGE ( 'NONE', *, *, #31350, .F. ) ;
#39771=VECTOR ( 'NONE', #25393, 1000.000000000000000 ) ;
#39772=CARTESIAN_POINT ( 'NONE',  ( -8.978675913592192970, -24.55319635012989110, 6.700000000000000178 ) ) ;
#39774=ORIENTED_EDGE ( 'NONE', *, *, #14447, .T. ) ;
#39786=EDGE_CURVE ( 'NONE', #39282, #5089, #7013, .T. ) ;
#39790=ORIENTED_EDGE ( 'NONE', *, *, #36997, .T. ) ;
#39791=ADVANCED_FACE ( 'NONE', ( #39156 ), #20030, .T. ) ;
#39793=ORIENTED_EDGE ( 'NONE', *, *, #9581, .T. ) ;
#39803=DIRECTION ( 'NONE',  ( -0.000000000000000000, -0.000000000000000000, 1.000000000000000000 ) ) ;
#39806=VECTOR ( 'NONE', #36992, 1000.000000000000000 ) ;
#39828=CARTESIAN_POINT ( 'NONE',  ( -10.87867591359219155, -24.55319635012989110, 6.700000000000000178 ) ) ;
#39835=AXIS2_PLACEMENT_3D ( 'NONE', #403, #15829, #28384 ) ;
#39837=EDGE_LOOP ( 'NONE', ( #18506, #10057, #28146, #14695 ) ) ;
#39839=DIRECTION ( 'NONE',  ( -0.000000000000000000, -0.000000000000000000, 1.000000000000000000 ) ) ;
#39845=ORIENTED_EDGE ( 'NONE', *, *, #30918, .T. ) ;
#39871=EDGE_LOOP ( 'NONE', ( #23724, #28820, #22069, #25727 ) ) ;
#39872=CARTESIAN_POINT ( 'NONE',  ( -42.83131703149249603, -27.06993018339339585, 6.000000000000000000 ) ) ;
#39875=CARTESIAN_POINT ( 'NONE',  ( -37.07867591359219261, -26.64985754041175525, 6.800000000000000711 ) ) ;
#39881=EDGE_CURVE ( 'NONE', #1672, #10219, #7412, .T. ) ;
#39886=LINE ( 'NONE', #14549, #40693 ) ;
#39907=CARTESIAN_POINT ( 'NONE',  ( -30.44874870218064089, -26.64985754041175525, 6.800000000000000711 ) ) ;
#39910=VECTOR ( 'NONE', #31712, 1000.000000000000000 ) ;
#39921=ORIENTED_EDGE ( 'NONE', *, *, #34676, .F. ) ;
#39923=ORIENTED_EDGE ( 'NONE', *, *, #39129, .F. ) ;
#39924=VERTEX_POINT ( 'NONE', #20561 ) ;
#39925=DIRECTION ( 'NONE',  ( -0.000000000000000000, -0.000000000000000000, 1.000000000000000000 ) ) ;
#39926=DIRECTION ( 'NONE',  ( -0.000000000000000000, -0.000000000000000000, 1.000000000000000000 ) ) ;
#39931=CARTESIAN_POINT ( 'NONE',  ( -20.34874870218063947, -26.64985754041175525, 6.800000000000000711 ) ) ;
#39932=ORIENTED_EDGE ( 'NONE', *, *, #10577, .F. ) ;
#39936=ADVANCED_FACE ( 'NONE', ( #11691 ), #2068, .F. ) ;
#39938=DIRECTION ( 'NONE',  ( 0.000000000000000000, 0.000000000000000000, 1.000000000000000000 ) ) ;
#39944=CARTESIAN_POINT ( 'NONE',  ( -17.07867591359219617, -26.64985754041175525, 6.800000000000000711 ) ) ;
#39949=CARTESIAN_POINT ( 'NONE',  ( -8.878675913592189772, -26.64985754041175525, 6.700000000000000178 ) ) ;
#39953=VECTOR ( 'NONE', #25459, 1000.000000000000000 ) ;
#39958=LINE ( 'NONE', #11129, #2288 ) ;
#39963=CARTESIAN_POINT ( 'NONE',  ( -0.4487487021806388365, -26.64985754041175525, 6.800000000000000711 ) ) ;
#39964=VERTEX_POINT ( 'NONE', #24684 ) ;
#39966=CIRCLE ( 'NONE', #10376, 0.1000000000000028644 ) ;
#39977=CYLINDRICAL_SURFACE ( 'NONE', #3691, 0.1000000000000028644 ) ;
#39985=ORIENTED_EDGE ( 'NONE', *, *, #32001, .T. ) ;
#40010=CARTESIAN_POINT ( 'NONE',  ( -24.34874870218063592, -26.64985754041175525, 6.700000000000000178 ) ) ;
#40012=DIRECTION ( 'NONE',  ( 0.000000000000000000, 1.000000000000000000, 0.000000000000000000 ) ) ;
#40015=DIRECTION ( 'NONE',  ( 1.000000000000000000, 0.000000000000000000, 0.000000000000000000 ) ) ;
#40018=EDGE_CURVE ( 'NONE', #38606, #23338, #8197, .T. ) ;
#40021=EDGE_CURVE ( 'NONE', #28284, #2900, #11898, .T. ) ;
#40028=LINE ( 'NONE', #11194, #37946 ) ;
#40041=CARTESIAN_POINT ( 'NONE',  ( -33.07867591359219972, -24.55319635012989110, 6.700000000000000178 ) ) ;
#40043=ORIENTED_EDGE ( 'NONE', *, *, #3447, .F. ) ;
#40050=DIRECTION ( 'NONE',  ( -0.000000000000000000, -0.000000000000000000, 1.000000000000000000 ) ) ;
#40051=PLANE ( 'NONE',  #26765 ) ;
#40057=LINE ( 'NONE', #12256, #25676 ) ;
#40066=DIRECTION ( 'NONE',  ( 0.000000000000000000, 0.000000000000000000, -1.000000000000000000 ) ) ;
#40072=DIRECTION ( 'NONE',  ( 1.000000000000000000, 0.000000000000000000, 0.000000000000000000 ) ) ;
#40093=EDGE_CURVE ( 'NONE', #2900, #36291, #23467, .T. ) ;
#40100=DIRECTION ( 'NONE',  ( 0.000000000000000000, 0.000000000000000000, -1.000000000000000000 ) ) ;
#40105=AXIS2_PLACEMENT_3D ( 'NONE', #967, #20475, #13906 ) ;
#40108=DIRECTION ( 'NONE',  ( -1.000000000000000000, 0.000000000000000000, 0.000000000000000000 ) ) ;
#40110=ORIENTED_EDGE ( 'NONE', *, *, #730, .F. ) ;
#40115=ORIENTED_EDGE ( 'NONE', *, *, #8921, .F. ) ;
#40116=ORIENTED_EDGE ( 'NONE', *, *, #10188, .F. ) ;
#40120=FACE_OUTER_BOUND ( 'NONE', #26007, .T. ) ;
#40123=EDGE_LOOP ( 'NONE', ( #13656, #24938, #2343, #37802 ) ) ;
#40125=LINE ( 'NONE', #7518, #16757 ) ;
#40127=CARTESIAN_POINT ( 'NONE',  ( 7.021324086407807030, -26.64985754041175525, 6.700000000000000178 ) ) ;
#40128=ORIENTED_EDGE ( 'NONE', *, *, #3699, .F. ) ;
#40133=CIRCLE ( 'NONE', #31604, 0.1000000000000028644 ) ;
#40136=CYLINDRICAL_SURFACE ( 'NONE', #4241, 0.1000000000000028644 ) ;
#40143=CARTESIAN_POINT ( 'NONE',  ( -28.97867591359219475, -24.55319635012989110, 6.700000000000000178 ) ) ;
#40150=AXIS2_PLACEMENT_3D ( 'NONE', #26211, #16914, #29494 ) ;
#40156=FACE_OUTER_BOUND ( 'NONE', #38514, .T. ) ;
#40160=ADVANCED_FACE ( 'NONE', ( #18914 ), #40513, .F. ) ;
#40164=ORIENTED_EDGE ( 'NONE', *, *, #7304, .F. ) ;
#40170=ORIENTED_EDGE ( 'NONE', *, *, #37038, .F. ) ;
#40171=CARTESIAN_POINT ( 'NONE',  ( -38.44874870218063734, -26.64985754041175525, 6.700000000000000178 ) ) ;
#40178=CIRCLE ( 'NONE', #18280, 0.1000000000000028644 ) ;
#40182=VERTEX_POINT ( 'NONE', #28381 ) ;
#40191=DIRECTION ( 'NONE',  ( 0.000000000000000000, 0.000000000000000000, 1.000000000000000000 ) ) ;
#40213=CYLINDRICAL_SURFACE ( 'NONE', #19767, 0.1000000000000028644 ) ;
#40216=ORIENTED_EDGE ( 'NONE', *, *, #14897, .T. ) ;
#40223=DIRECTION ( 'NONE',  ( 0.000000000000000000, 0.000000000000000000, 1.000000000000000000 ) ) ;
#40226=LINE ( 'NONE', #12008, #26033 ) ;
#40236=EDGE_CURVE ( 'NONE', #2729, #3866, #4294, .T. ) ;
#40250=CARTESIAN_POINT ( 'NONE',  ( -40.34874870218063592, -26.64985754041175525, 6.800000000000000711 ) ) ;
#40252=FACE_OUTER_BOUND ( 'NONE', #26950, .T. ) ;
#40268=DIRECTION ( 'NONE',  ( 0.000000000000000000, 0.000000000000000000, 1.000000000000000000 ) ) ;
#40280=VERTEX_POINT ( 'NONE', #16425 ) ;
#40283=CYLINDRICAL_SURFACE ( 'NONE', #12717, 0.1000000000000028644 ) ;
#40290=EDGE_LOOP ( 'NONE', ( #15854, #16271, #39496, #16733 ) ) ;
#40292=EDGE_CURVE ( 'NONE', #20694, #2944, #28764, .T. ) ;
#40302=CYLINDRICAL_SURFACE ( 'NONE', #36833, 0.1000000000000028644 ) ;
#40310=DIRECTION ( 'NONE',  ( 0.000000000000000000, 0.000000000000000000, 1.000000000000000000 ) ) ;
#40311=VERTEX_POINT ( 'NONE', #36983 ) ;
#40318=EDGE_LOOP ( 'NONE', ( #25914, #4252, #1563, #20510 ) ) ;
#40319=EDGE_LOOP ( 'NONE', ( #37109, #25179, #18899, #8842 ) ) ;
#40326=ADVANCED_FACE ( 'NONE', ( #12054 ), #27106, .T. ) ;
#40328=VECTOR ( 'NONE', #17366, 1000.000000000000000 ) ;
#40331=ORIENTED_EDGE ( 'NONE', *, *, #31072, .F. ) ;
#40332=CARTESIAN_POINT ( 'NONE',  ( -16.34874870218063592, -25.49307895267003587, 6.700000000000000178 ) ) ;
#40339=FACE_OUTER_BOUND ( 'NONE', #1552, .T. ) ;
#40340=ADVANCED_FACE ( 'NONE', ( #21143 ), #11236, .F. ) ;
#40349=DIRECTION ( 'NONE',  ( 1.000000000000000000, 0.000000000000000000, 0.000000000000000000 ) ) ;
#40354=ORIENTED_EDGE ( 'NONE', *, *, #7073, .F. ) ;
#40355=CARTESIAN_POINT ( 'NONE',  ( -10.44874870218064089, -26.64985754041175525, 6.700000000000000178 ) ) ;
#40361=CARTESIAN_POINT ( 'NONE',  ( -8.448748702180639114, -26.64985754041175525, 6.800000000000000711 ) ) ;
#40367=LINE ( 'NONE', #2121, #37180 ) ;
#40368=LINE ( 'NONE', #30732, #18593 ) ;
#40378=CARTESIAN_POINT ( 'NONE',  ( -18.34874870218063947, -25.49307895267003587, 6.700000000000000178 ) ) ;
#40382=VERTEX_POINT ( 'NONE', #5489 ) ;
#40383=ADVANCED_FACE ( 'NONE', ( #20719 ), #33515, .F. ) ;
#40386=DIRECTION ( 'NONE',  ( -0.000000000000000000, -0.000000000000000000, 1.000000000000000000 ) ) ;
#40388=ORIENTED_EDGE ( 'NONE', *, *, #3402, .F. ) ;
#40395=LINE ( 'NONE', #12197, #33862 ) ;
#40406=DIRECTION ( 'NONE',  ( 1.000000000000000000, 0.000000000000000000, -0.000000000000000000 ) ) ;
#40407=CARTESIAN_POINT ( 'NONE',  ( 1.021324086407808585, -26.64985754041175525, 6.800000000000000711 ) ) ;
#40411=DIRECTION ( 'NONE',  ( -0.000000000000000000, -1.000000000000000000, -0.000000000000000000 ) ) ;
#40415=AXIS2_PLACEMENT_3D ( 'NONE', #7220, #1065, #7817 ) ;
#40417=CARTESIAN_POINT ( 'NONE',  ( -36.87867591359218977, -24.55319635012989110, 6.700000000000000178 ) ) ;
#40418=CARTESIAN_POINT ( 'NONE',  ( 3.751251297819363728, -26.64985754041175525, 6.700000000000000178 ) ) ;
#40429=AXIS2_PLACEMENT_3D ( 'NONE', #11047, #38452, #4504 ) ;
#40437=VECTOR ( 'NONE', #10242, 1000.000000000000000 ) ;
#40442=CARTESIAN_POINT ( 'NONE',  ( 1.651251297819358754, -25.49307895267003587, 6.700000000000000178 ) ) ;
#40444=CARTESIAN_POINT ( 'NONE',  ( -38.44874870218063734, -26.64985754041175525, 6.800000000000000711 ) ) ;
#40447=CARTESIAN_POINT ( 'NONE',  ( -26.97867591359219475, -26.64985754041175525, 6.700000000000000178 ) ) ;
#40451=ORIENTED_EDGE ( 'NONE', *, *, #40512, .T. ) ;
#40456=VECTOR ( 'NONE', #33081, 1000.000000000000000 ) ;
#40464=CIRCLE ( 'NONE', #31275, 0.1000000000000028644 ) ;
#40465=LINE ( 'NONE', #25656, #37070 ) ;
#40467=FACE_OUTER_BOUND ( 'NONE', #29044, .T. ) ;
#40471=DIRECTION ( 'NONE',  ( 0.000000000000000000, 0.000000000000000000, 1.000000000000000000 ) ) ;
#40483=ORIENTED_EDGE ( 'NONE', *, *, #1049, .T. ) ;
#40497=DIRECTION ( 'NONE',  ( -1.000000000000000000, 0.000000000000000000, 0.000000000000000000 ) ) ;
#40498=LINE ( 'NONE', #182, #33770 ) ;
#40506=EDGE_LOOP ( 'NONE', ( #6632, #6817, #3569, #32439 ) ) ;
#40508=CARTESIAN_POINT ( 'NONE',  ( -21.07867591359219617, -26.64985754041175525, 6.800000000000000711 ) ) ;
#40512=EDGE_CURVE ( 'NONE', #21149, #9410, #40028, .T. ) ;
#40513=CYLINDRICAL_SURFACE ( 'NONE', #16237, 0.1000000000000028644 ) ;
#40519=ORIENTED_EDGE ( 'NONE', *, *, #9288, .T. ) ;
#40521=AXIS2_PLACEMENT_3D ( 'NONE', #37028, #24272, #11493 ) ;
#40527=CIRCLE ( 'NONE', #23442, 0.1000000000000028644 ) ;
#40537=EDGE_LOOP ( 'NONE', ( #26797, #31938, #6369, #31993 ) ) ;
#40547=CIRCLE ( 'NONE', #13614, 2.499999999999996891 ) ;
#40550=CARTESIAN_POINT ( 'NONE',  ( -14.44874870218064089, -26.64985754041175525, 6.700000000000000178 ) ) ;
#40551=CARTESIAN_POINT ( 'NONE',  ( -42.83131703149249603, -29.56993018339339940, 6.800000000000000711 ) ) ;
#40552=( GEOMETRIC_REPRESENTATION_CONTEXT ( 3 ) GLOBAL_UNCERTAINTY_ASSIGNED_CONTEXT ( ( #12276 ) ) GLOBAL_UNIT_ASSIGNED_CONTEXT ( ( #15675, #22683, #28646 ) ) REPRESENTATION_CONTEXT ( 'NONE', 'WORKASPACE' ) );
#40554=AXIS2_PLACEMENT_3D ( 'NONE', #14013, #20390, #19802 ) ;
#40555=EDGE_CURVE ( 'NONE', #37478, #10099, #7918, .T. ) ;
#40556=CIRCLE ( 'NONE', #14260, 0.1000000000000028644 ) ;
#40557=DIRECTION ( 'NONE',  ( 1.000000000000000000, 0.000000000000000000, 0.000000000000000000 ) ) ;
#40558=EDGE_CURVE ( 'NONE', #37250, #7879, #1555, .T. ) ;
#40566=ADVANCED_FACE ( 'NONE', ( #8518 ), #29945, .T. ) ;
#40567=EDGE_LOOP ( 'NONE', ( #7009, #5587, #12371, #17611 ) ) ;
#40570=DIRECTION ( 'NONE',  ( 0.000000000000000000, 0.000000000000000000, 1.000000000000000000 ) ) ;
#40584=LINE ( 'NONE', #12795, #29849 ) ;
#40591=AXIS2_PLACEMENT_3D ( 'NONE', #33849, #9116, #12411 ) ;
#40600=LINE ( 'NONE', #34463, #35919 ) ;
#40604=FACE_OUTER_BOUND ( 'NONE', #25738, .T. ) ;
#40607=PLANE ( 'NONE',  #18195 ) ;
#40609=CARTESIAN_POINT ( 'NONE',  ( -0.3487487021806359722, -26.64985754041175525, 6.700000000000000178 ) ) ;
#40611=CARTESIAN_POINT ( 'NONE',  ( -4.348748702180639469, -26.64985754041175525, 6.700000000000000178 ) ) ;
#40619=AXIS2_PLACEMENT_3D ( 'NONE', #2039, #14554, #30430 ) ;
#40636=PLANE ( 'NONE',  #11597 ) ;
#40637=EDGE_LOOP ( 'NONE', ( #23228, #51, #9386, #17624 ) ) ;
#40638=VERTEX_POINT ( 'NONE', #35247 ) ;
#40644=ORIENTED_EDGE ( 'NONE', *, *, #17922, .F. ) ;
#40655=AXIS2_PLACEMENT_3D ( 'NONE', #36162, #39228, #23598 ) ;
#40667=CARTESIAN_POINT ( 'NONE',  ( -11.07867591359219794, -26.64985754041175525, 6.800000000000000711 ) ) ;
#40683=EDGE_LOOP ( 'NONE', ( #14035, #25258, #11332, #9396 ) ) ;
#40688=CARTESIAN_POINT ( 'NONE',  ( -19.07867591359219972, -26.64985754041175525, 6.700000000000000178 ) ) ;
#40691=VERTEX_POINT ( 'NONE', #28435 ) ;
#40693=VECTOR ( 'NONE', #2233, 1000.000000000000000 ) ;
#40700=ORIENTED_EDGE ( 'NONE', *, *, #14342, .F. ) ;
#40714=DIRECTION ( 'NONE',  ( 0.000000000000000000, 1.000000000000000000, 0.000000000000000000 ) ) ;
#40767=COLOUR_RGB('Off White',0.89,0.88,0.83);
#40768=FILL_AREA_STYLE_COLOUR('',#40767);
#40769=FILL_AREA_STYLE('',(#40768));
#40770=SURFACE_STYLE_FILL_AREA(#40769);
#40771=SURFACE_SIDE_STYLE('',(#40770));
#40772=SURFACE_STYLE_USAGE(.BOTH.,#40771);
#40773=PRESENTATION_STYLE_ASSIGNMENT((#40772));
ENDSEC;
END-ISO-10303-21;
